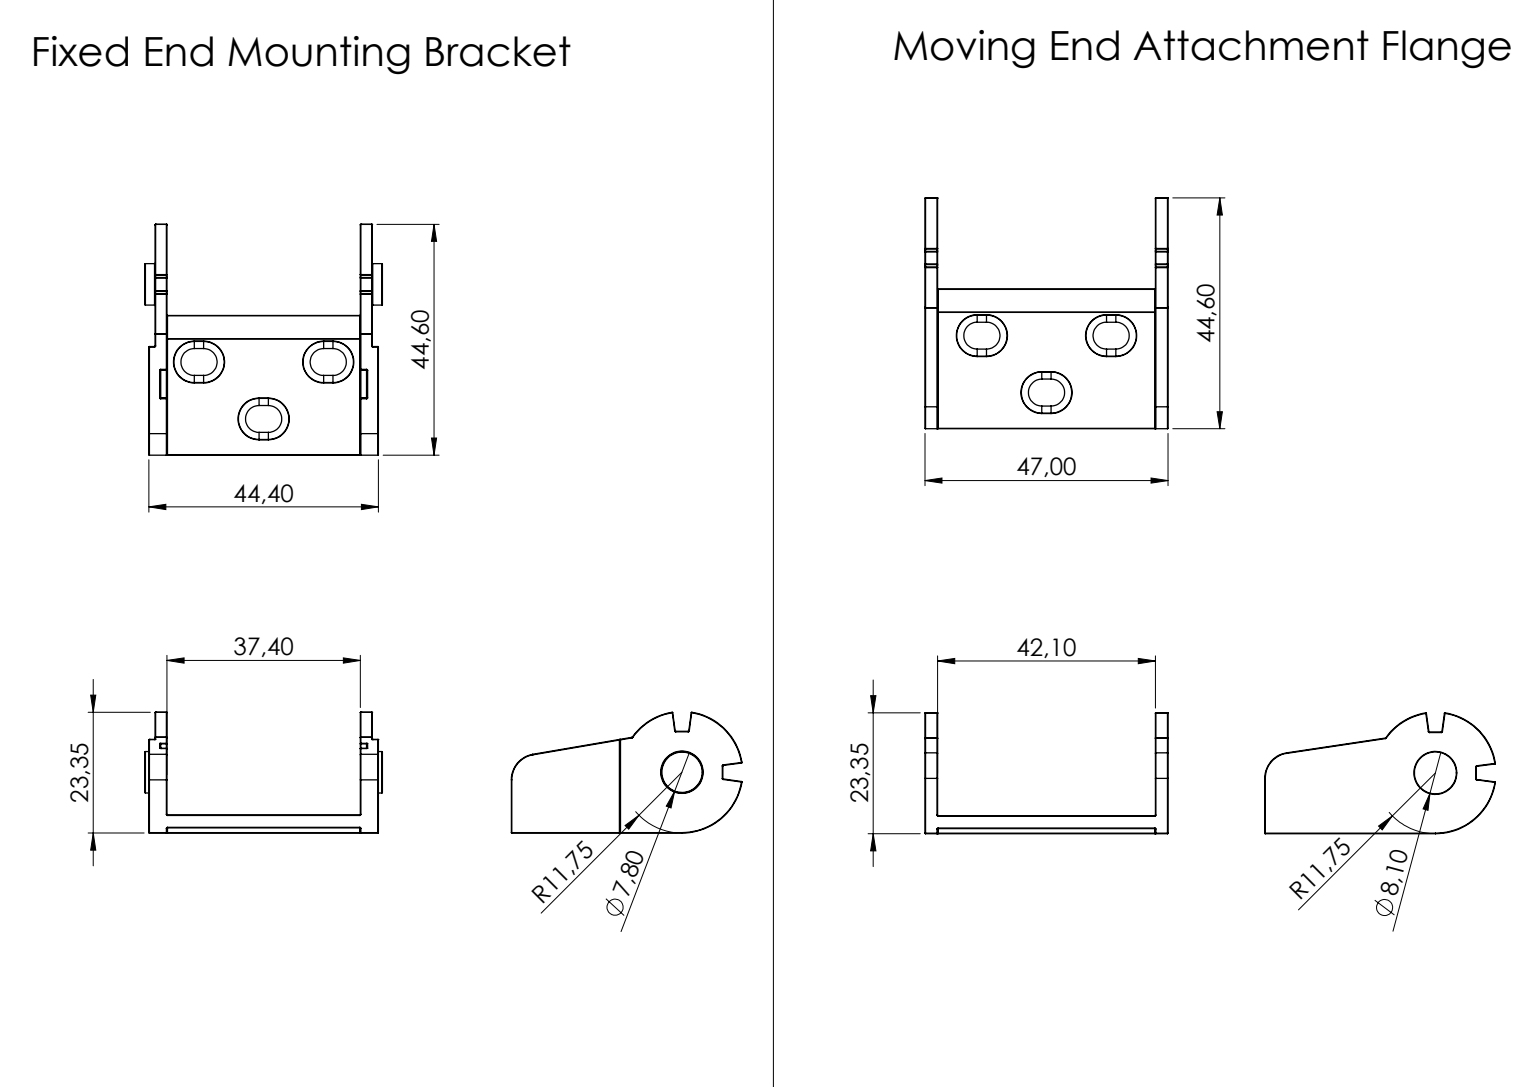
ISO-10303-21;
HEADER;
FILE_DESCRIPTION (('STEP AP214'),
    '1' );
FILE_NAME ('Fixed End Mounting Bracket.step',
    '2026-10-08T22:59:04',
    ( '' ),
    ( '' ),
    'SwSTEP 2.0',
    'SolidWorks 2020',
    '' );
FILE_SCHEMA (( 'AUTOMOTIVE_DESIGN' ));
ENDSEC;

DATA;
#41=ADVANCED_FACE ( 'NONE', ( #121306 ), #43023, .F. ) ;
#64=DIRECTION ( 'NONE',  ( 0.000000000000000000, 0.000000000000000000, 1.000000000000000000 ) ) ;
#92=CARTESIAN_POINT ( 'NONE',  ( -20.90000000000000213, 6.336640076952988920, 12.03401928653448572 ) ) ;
#126=VERTEX_POINT ( 'NONE', #92393 ) ;
#149=AXIS2_PLACEMENT_3D ( 'NONE', #44529, #5360, #61520 ) ;
#183=ADVANCED_FACE ( 'NONE', ( #7745 ), #109386, .T. ) ;
#187=EDGE_LOOP ( 'NONE', ( #19437, #210011, #114046, #182505, #122843 ) ) ;
#208=CIRCLE ( 'NONE', #96054, 11.75000000000000000 ) ;
#224=AXIS2_PLACEMENT_3D ( 'NONE', #149688, #207076, #227918 ) ;
#237=AXIS2_PLACEMENT_3D ( 'NONE', #83814, #157333, #257616 ) ;
#267=DIRECTION ( 'NONE',  ( 0.000000000000000000, -1.000000000000000000, 0.000000000000000000 ) ) ;
#284=EDGE_CURVE ( 'NONE', #234077, #216189, #164488, .T. ) ;
#339=ADVANCED_FACE ( 'NONE', ( #38863 ), #118398, .T. ) ;
#453=DIRECTION ( 'NONE',  ( 1.000000000000000000, 0.000000000000000000, -0.000000000000000000 ) ) ;
#495=VECTOR ( 'NONE', #96044, 1000.000000000000000 ) ;
#497=CARTESIAN_POINT ( 'NONE',  ( -22.10000000000000142, -11.65000000000000036, 12.09999999999999609 ) ) ;
#504=DIRECTION ( 'NONE',  ( 0.000000000000000000, 1.000000000000000000, 0.000000000000000000 ) ) ;
#539=FACE_OUTER_BOUND ( 'NONE', #95996, .T. ) ;
#576=DIRECTION ( 'NONE',  ( 0.000000000000000000, 1.000000000000000000, 0.000000000000000000 ) ) ;
#604=SPHERICAL_SURFACE ( 'NONE', #217070, 0.1000000000000000056 ) ;
#605=DIRECTION ( 'NONE',  ( 1.000000000000000000, -0.000000000000000000, 0.000000000000000000 ) ) ;
#660=CIRCLE ( 'NONE', #167314, 0.1000000000000002554 ) ;
#678=ORIENTED_EDGE ( 'NONE', *, *, #100875, .T. ) ;
#691=VERTEX_POINT ( 'NONE', #157234 ) ;
#709=CARTESIAN_POINT ( 'NONE',  ( 18.69999999999999929, -11.65000000000000036, -15.00000000000000000 ) ) ;
#736=ORIENTED_EDGE ( 'NONE', *, *, #51566, .T. ) ;
#739=CARTESIAN_POINT ( 'NONE',  ( 21.10000000000000142, 6.223900101154156594, 12.09999999999999964 ) ) ;
#754=EDGE_LOOP ( 'NONE', ( #252584, #112082, #982, #102048 ) ) ;
#803=EDGE_LOOP ( 'NONE', ( #185870, #252756, #109743, #49629 ) ) ;
#825=CARTESIAN_POINT ( 'NONE',  ( -21.00000000000000000, 7.800000000000000711, -1.212568896937008089 ) ) ;
#890=DIRECTION ( 'NONE',  ( -1.476360405086644309E-16, -1.000000000000000000, -0.000000000000000000 ) ) ;
#959=CARTESIAN_POINT ( 'NONE',  ( 13.40000000000000036, -11.65000000000000036, 17.70000000000000284 ) ) ;
#967=VECTOR ( 'NONE', #117987, 1000.000000000000114 ) ;
#975=VERTEX_POINT ( 'NONE', #144040 ) ;
#982=ORIENTED_EDGE ( 'NONE', *, *, #230832, .F. ) ;
#998=VECTOR ( 'NONE', #226913, 1000.000000000000000 ) ;
#1011=CYLINDRICAL_SURFACE ( 'NONE', #164253, 0.1000000000000001443 ) ;
#1037=TOROIDAL_SURFACE ( 'NONE', #71828, 0.2000000000000000111, 0.1000000000000000056 ) ;
#1051=ADVANCED_FACE ( 'NONE', ( #15824 ), #217817, .T. ) ;
#1072=CARTESIAN_POINT ( 'NONE',  ( 18.79999999999999716, 6.841561409100513025, 9.675512259591560138 ) ) ;
#1117=ORIENTED_EDGE ( 'NONE', *, *, #211260, .F. ) ;
#1141=EDGE_CURVE ( 'NONE', #118769, #81824, #59092, .T. ) ;
#1148=DIRECTION ( 'NONE',  ( 0.000000000000000000, -0.1335171055202864221, 0.9910465087640865089 ) ) ;
#1165=ORIENTED_EDGE ( 'NONE', *, *, #245877, .T. ) ;
#1224=VERTEX_POINT ( 'NONE', #31242 ) ;
#1234=CARTESIAN_POINT ( 'NONE',  ( -18.59999999999999787, -11.75000000000000000, 29.89999999999999858 ) ) ;
#1236=CARTESIAN_POINT ( 'NONE',  ( -18.59999999999999787, 11.75000000000000000, 30.09999999999999787 ) ) ;
#1243=ORIENTED_EDGE ( 'NONE', *, *, #90316, .T. ) ;
#1267=EDGE_CURVE ( 'NONE', #34286, #18345, #17600, .T. ) ;
#1279=DIRECTION ( 'NONE',  ( -0.000000000000000000, 1.000000000000000000, -0.000000000000000000 ) ) ;
#1290=FACE_OUTER_BOUND ( 'NONE', #252660, .T. ) ;
#1333=DIRECTION ( 'NONE',  ( 0.000000000000000000, 0.000000000000000000, 1.000000000000000000 ) ) ;
#1339=FACE_BOUND ( 'NONE', #186909, .T. ) ;
#1346=ADVANCED_FACE ( 'NONE', ( #229406 ), #188493, .T. ) ;
#1351=EDGE_LOOP ( 'NONE', ( #149134, #36739, #59727, #188975 ) ) ;
#1352=CARTESIAN_POINT ( 'NONE',  ( 13.40000000000000036, -8.350000000000004974, 19.04142135623731136 ) ) ;
#1419=DIRECTION ( 'NONE',  ( 0.000000000000000000, 0.000000000000000000, -1.000000000000000000 ) ) ;
#1439=ORIENTED_EDGE ( 'NONE', *, *, #171966, .F. ) ;
#1461=ADVANCED_FACE ( 'NONE', ( #80550 ), #121028, .T. ) ;
#1491=DIRECTION ( 'NONE',  ( 0.000000000000000000, -0.8164989248600462712, 0.5773469543544753613 ) ) ;
#1524=FACE_OUTER_BOUND ( 'NONE', #20858, .T. ) ;
#1526=VECTOR ( 'NONE', #257656, 1000.000000000000000 ) ;
#1596=AXIS2_PLACEMENT_3D ( 'NONE', #245526, #66878, #107284 ) ;
#1654=ADVANCED_FACE ( 'NONE', ( #246089 ), #129957, .F. ) ;
#1677=ORIENTED_EDGE ( 'NONE', *, *, #116347, .F. ) ;
#1687=ORIENTED_EDGE ( 'NONE', *, *, #137543, .F. ) ;
#1729=VERTEX_POINT ( 'NONE', #175549 ) ;
#1745=DIRECTION ( 'NONE',  ( 1.000000000000000000, 0.000000000000000000, 0.000000000000000000 ) ) ;
#1778=ADVANCED_FACE ( 'NONE', ( #195115 ), #16473, .T. ) ;
#1785=CIRCLE ( 'NONE', #147559, 0.09999999999999939493 ) ;
#1792=LINE ( 'NONE', #116623, #180804 ) ;
#1819=DIRECTION ( 'NONE',  ( 1.000000000000000000, 0.000000000000000000, 0.000000000000000000 ) ) ;
#1843=CARTESIAN_POINT ( 'NONE',  ( -6.000000000000003553, -11.65000000000000036, 10.00000000000000178 ) ) ;
#1922=CIRCLE ( 'NONE', #18693, 4.900000000000003020 ) ;
#2023=DIRECTION ( 'NONE',  ( -0.000000000000000000, 1.000000000000000000, -0.000000000000000000 ) ) ;
#2042=ORIENTED_EDGE ( 'NONE', *, *, #74139, .F. ) ;
#2050=CARTESIAN_POINT ( 'NONE',  ( -0.8999999999999994671, -8.350000000000003197, 21.95857864376269220 ) ) ;
#2071=AXIS2_PLACEMENT_3D ( 'NONE', #163669, #185794, #86661 ) ;
#2114=ADVANCED_FACE ( 'NONE', ( #116537 ), #211788, .T. ) ;
#2129=DIRECTION ( 'NONE',  ( 0.000000000000000000, 0.000000000000000000, -1.000000000000000000 ) ) ;
#2147=VERTEX_POINT ( 'NONE', #216897 ) ;
#2150=CARTESIAN_POINT ( 'NONE',  ( 20.09999999673965121, 5.571292164246353984, 16.50791943615039514 ) ) ;
#2234=VECTOR ( 'NONE', #4879, 1000.000000000000000 ) ;
#2304=CARTESIAN_POINT ( 'NONE',  ( -6.000000000000002665, -11.25000000000000000, 14.00000000000000178 ) ) ;
#2307=DIRECTION ( 'NONE',  ( 4.336808689942017736E-16, 0.000000000000000000, 1.000000000000000000 ) ) ;
#2318=CARTESIAN_POINT ( 'NONE',  ( -22.10000000000000497, 6.223900101154156594, 12.09999999999999964 ) ) ;
#2328=AXIS2_PLACEMENT_3D ( 'NONE', #70395, #7830, #149920 ) ;
#2358=EDGE_CURVE ( 'NONE', #239783, #205125, #234657, .T. ) ;
#2425=AXIS2_PLACEMENT_3D ( 'NONE', #153513, #135160, #16531 ) ;
#2475=ORIENTED_EDGE ( 'NONE', *, *, #234542, .T. ) ;
#2486=EDGE_CURVE ( 'NONE', #219374, #227995, #238605, .T. ) ;
#2561=CARTESIAN_POINT ( 'NONE',  ( -22.10000000000000142, -11.64999999999999858, 12.09999999999999609 ) ) ;
#2564=DIRECTION ( 'NONE',  ( 1.000000000000000000, 5.204170427930452838E-14, 0.000000000000000000 ) ) ;
#2588=CARTESIAN_POINT ( 'NONE',  ( -37.88850191057539973, 11.75000000000000000, 6.000000000000001776 ) ) ;
#2624=CYLINDRICAL_SURFACE ( 'NONE', #233334, 0.09999999999999990841 ) ;
#2683=ORIENTED_EDGE ( 'NONE', *, *, #33531, .T. ) ;
#2711=AXIS2_PLACEMENT_3D ( 'NONE', #47359, #90346, #129493 ) ;
#2743=CARTESIAN_POINT ( 'NONE',  ( -18.70000000000000284, 7.900000000000000355, 1.212568896937007867 ) ) ;
#2774=CIRCLE ( 'NONE', #236010, 0.09999999999999990841 ) ;
#2777=PLANE ( 'NONE',  #123368 ) ;
#2798=VECTOR ( 'NONE', #76671, 1000.000000000000000 ) ;
#2843=CARTESIAN_POINT ( 'NONE',  ( 18.79999999999999716, 6.783826713665066066, 9.593862367105556288 ) ) ;
#2853=VECTOR ( 'NONE', #232428, 1000.000000000000114 ) ;
#2924=EDGE_CURVE ( 'NONE', #166883, #29111, #110106, .T. ) ;
#2933=CYLINDRICAL_SURFACE ( 'NONE', #81036, 0.09999999999999939493 ) ;
#3014=CARTESIAN_POINT ( 'NONE',  ( -22.84999999999999787, 0.000000000000000000, 0.000000000000000000 ) ) ;
#3017=CARTESIAN_POINT ( 'NONE',  ( -21.10000000000000142, -11.64999999999999858, 11.99999999999999645 ) ) ;
#3030=CARTESIAN_POINT ( 'NONE',  ( 20.10000000000000853, 4.645987002755569861, 21.91686199900910736 ) ) ;
#3071=CARTESIAN_POINT ( 'NONE',  ( 20.89999999999999858, -11.75000000000000000, 11.89999999999999680 ) ) ;
#3085=AXIS2_PLACEMENT_3D ( 'NONE', #145893, #127634, #7698 ) ;
#3098=CARTESIAN_POINT ( 'NONE',  ( 18.59999999999999787, -9.849999999999994316, 30.09999999999999787 ) ) ;
#3161=CARTESIAN_POINT ( 'NONE',  ( 18.79999999999999716, -1.885425182446134107, -11.59641995933507808 ) ) ;
#3206=CARTESIAN_POINT ( 'NONE',  ( 18.79999999999999716, 11.49641995933507843, 1.885425182446133885 ) ) ;
#3219=DIRECTION ( 'NONE',  ( -0.000000000000000000, 0.9910465087640860649, 0.1335171055202901413 ) ) ;
#3268=CIRCLE ( 'NONE', #36650, 0.1000000000000000472 ) ;
#3271=ORIENTED_EDGE ( 'NONE', *, *, #83209, .F. ) ;
#3359=CYLINDRICAL_SURFACE ( 'NONE', #28672, 0.1000000000000000472 ) ;
#3419=DIRECTION ( 'NONE',  ( 0.000000000000000000, 0.000000000000000000, -1.000000000000000000 ) ) ;
#3449=EDGE_CURVE ( 'NONE', #86236, #255967, #27127, .T. ) ;
#3491=DIRECTION ( 'NONE',  ( 1.000000000000000000, 0.000000000000000000, 0.000000000000000000 ) ) ;
#3501=EDGE_CURVE ( 'NONE', #252739, #56541, #35327, .T. ) ;
#3516=ORIENTED_EDGE ( 'NONE', *, *, #242810, .F. ) ;
#3541=DIRECTION ( 'NONE',  ( 0.000000000000000000, 0.000000000000000000, -1.000000000000000000 ) ) ;
#3551=ORIENTED_EDGE ( 'NONE', *, *, #74542, .T. ) ;
#3558=DIRECTION ( 'NONE',  ( 2.168404344971008868E-16, 0.000000000000000000, 1.000000000000000000 ) ) ;
#3600=FACE_OUTER_BOUND ( 'NONE', #170206, .T. ) ;
#3613=CARTESIAN_POINT ( 'NONE',  ( 18.59999999999999787, -8.150000000000007461, 33.00000000000000000 ) ) ;
#3619=ORIENTED_EDGE ( 'NONE', *, *, #97666, .T. ) ;
#3638=DIRECTION ( 'NONE',  ( 0.000000000000000000, 0.000000000000000000, -1.000000000000000000 ) ) ;
#3653=AXIS2_PLACEMENT_3D ( 'NONE', #213131, #137431, #235256 ) ;
#3657=ORIENTED_EDGE ( 'NONE', *, *, #144860, .T. ) ;
#3734=VECTOR ( 'NONE', #55279, 1000.000000000000114 ) ;
#3738=VERTEX_POINT ( 'NONE', #126244 ) ;
#3792=DIRECTION ( 'NONE',  ( 1.000000000000000000, 0.000000000000000000, -0.000000000000000000 ) ) ;
#3847=CARTESIAN_POINT ( 'NONE',  ( 18.69999999999999929, 13.48082180182240819, -2.152770446119438130 ) ) ;
#3921=ORIENTED_EDGE ( 'NONE', *, *, #230794, .T. ) ;
#3965=EDGE_CURVE ( 'NONE', #120372, #6846, #74023, .T. ) ;
#4061=CARTESIAN_POINT ( 'NONE',  ( 20.90000000000000213, 6.783826713665066066, 9.593862367105556288 ) ) ;
#4072=DIRECTION ( 'NONE',  ( 1.000000000000000000, 0.000000000000000000, 0.000000000000000000 ) ) ;
#4080=ADVANCED_FACE ( 'NONE', ( #122104 ), #257691, .F. ) ;
#4122=FACE_OUTER_BOUND ( 'NONE', #6960, .T. ) ;
#4146=AXIS2_PLACEMENT_3D ( 'NONE', #228967, #90718, #131136 ) ;
#4152=LINE ( 'NONE', #44579, #184468 ) ;
#4188=AXIS2_PLACEMENT_3D ( 'NONE', #227607, #206772, #110226 ) ;
#4213=LINE ( 'NONE', #22529, #191256 ) ;
#4245=CARTESIAN_POINT ( 'NONE',  ( 22.10000000000000142, -3.262756495241484158E-15, 33.00000000000000000 ) ) ;
#4267=EDGE_CURVE ( 'NONE', #92180, #44902, #131505, .T. ) ;
#4282=ORIENTED_EDGE ( 'NONE', *, *, #241945, .T. ) ;
#4370=ADVANCED_FACE ( 'NONE', ( #539 ), #103482, .F. ) ;
#4421=LINE ( 'NONE', #83919, #253429 ) ;
#4438=CARTESIAN_POINT ( 'NONE',  ( -18.59999999999999787, -9.849999999999994316, 30.09999999999999787 ) ) ;
#4483=DIRECTION ( 'NONE',  ( 0.000000000000000000, 0.000000000000000000, -1.000000000000000000 ) ) ;
#4552=ORIENTED_EDGE ( 'NONE', *, *, #61719, .T. ) ;
#4630=ORIENTED_EDGE ( 'NONE', *, *, #141720, .T. ) ;
#4636=ORIENTED_EDGE ( 'NONE', *, *, #215592, .T. ) ;
#4637=DIRECTION ( 'NONE',  ( 1.000000000000000000, -0.000000000000000000, -0.000000000000000000 ) ) ;
#4689=CARTESIAN_POINT ( 'NONE',  ( -18.59999999999999787, -8.350000000000004974, 10.52591260281975138 ) ) ;
#4690=FACE_OUTER_BOUND ( 'NONE', #81853, .T. ) ;
#4754=TOROIDAL_SURFACE ( 'NONE', #38128, 2.699999999999999734, 0.1000000000000000056 ) ;
#4815=CARTESIAN_POINT ( 'NONE',  ( 18.59999999999999787, -11.75000000000000000, 29.89999999999999858 ) ) ;
#4828=ORIENTED_EDGE ( 'NONE', *, *, #139777, .F. ) ;
#4859=ORIENTED_EDGE ( 'NONE', *, *, #16669, .F. ) ;
#4879=DIRECTION ( 'NONE',  ( 1.000000000000000000, 0.000000000000000000, 0.000000000000000000 ) ) ;
#4900=LINE ( 'NONE', #234236, #76259 ) ;
#4904=CARTESIAN_POINT ( 'NONE',  ( -18.69999999999999929, -8.175168544775697654, 10.42878401658402510 ) ) ;
#4929=DIRECTION ( 'NONE',  ( 0.000000000000000000, 0.000000000000000000, -1.000000000000000000 ) ) ;
#4955=ORIENTED_EDGE ( 'NONE', *, *, #96401, .T. ) ;
#4967=EDGE_CURVE ( 'NONE', #172933, #119804, #217712, .T. ) ;
#4990=DIRECTION ( 'NONE',  ( -0.000000000000000000, 0.000000000000000000, -1.000000000000000000 ) ) ;
#4992=FACE_OUTER_BOUND ( 'NONE', #63102, .T. ) ;
#5028=DIRECTION ( 'NONE',  ( 0.000000000000000000, -0.9910465087640861759, -0.1335171055202901691 ) ) ;
#5031=LINE ( 'NONE', #44202, #91258 ) ;
#5040=DIRECTION ( 'NONE',  ( 1.000000000000000000, 0.000000000000000000, 0.000000000000000000 ) ) ;
#5080=VERTEX_POINT ( 'NONE', #116060 ) ;
#5094=EDGE_CURVE ( 'NONE', #73306, #188929, #47029, .T. ) ;
#5097=CARTESIAN_POINT ( 'NONE',  ( -18.79999999999999716, -8.150000000000005684, 32.89999999999999858 ) ) ;
#5118=CARTESIAN_POINT ( 'NONE',  ( -11.60000000000000320, -11.75000000000000000, 12.30000000000000426 ) ) ;
#5188=ADVANCED_FACE ( 'NONE', ( #244973 ), #230202, .F. ) ;
#5266=ORIENTED_EDGE ( 'NONE', *, *, #96420, .F. ) ;
#5299=AXIS2_PLACEMENT_3D ( 'NONE', #140383, #159989, #178273 ) ;
#5313=DIRECTION ( 'NONE',  ( 0.000000000000000000, -0.9910465087640860649, -0.1335171055202901413 ) ) ;
#5331=DIRECTION ( 'NONE',  ( 1.000000000000000000, 0.000000000000000000, 0.000000000000000000 ) ) ;
#5360=DIRECTION ( 'NONE',  ( 0.000000000000000000, -1.000000000000000000, 0.000000000000000000 ) ) ;
#5371=CIRCLE ( 'NONE', #159540, 2.699999999999999289 ) ;
#5385=CARTESIAN_POINT ( 'NONE',  ( -18.59999999999999787, -11.75000000000000000, 5.900000000000001243 ) ) ;
#5427=PRODUCT_DEFINITION ( 'UNKNOWN', '', #69634, #100050 ) ;
#5432=CARTESIAN_POINT ( 'NONE',  ( -21.10000000000000142, 0.000000000000000000, 0.000000000000000000 ) ) ;
#5456=EDGE_LOOP ( 'NONE', ( #217930, #251861, #121783, #237435 ) ) ;
#5556=DIRECTION ( 'NONE',  ( 1.000000000000000000, -0.000000000000000000, 0.000000000000000000 ) ) ;
#5568=VERTEX_POINT ( 'NONE', #108688 ) ;
#5645=EDGE_CURVE ( 'NONE', #194417, #150252, #248397, .T. ) ;
#5669=VERTEX_POINT ( 'NONE', #7013 ) ;
#5674=FACE_OUTER_BOUND ( 'NONE', #24234, .T. ) ;
#5678=FACE_OUTER_BOUND ( 'NONE', #72669, .T. ) ;
#5679=FACE_OUTER_BOUND ( 'NONE', #105384, .T. ) ;
#5712=DIRECTION ( 'NONE',  ( 0.000000000000000000, 0.000000000000000000, 1.000000000000000000 ) ) ;
#5762=AXIS2_PLACEMENT_3D ( 'NONE', #31364, #249105, #129143 ) ;
#5812=EDGE_CURVE ( 'NONE', #155056, #32241, #211000, .T. ) ;
#5833=AXIS2_PLACEMENT_3D ( 'NONE', #21551, #101019, #180617 ) ;
#5834=CARTESIAN_POINT ( 'NONE',  ( 11.60000000000000142, -8.350000000000004974, 10.95857864376269575 ) ) ;
#5907=ORIENTED_EDGE ( 'NONE', *, *, #56458, .T. ) ;
#5926=FACE_OUTER_BOUND ( 'NONE', #220597, .T. ) ;
#5938=TOROIDAL_SURFACE ( 'NONE', #47632, 0.2000000000000000111, 0.1000000000000000056 ) ;
#5962=ORIENTED_EDGE ( 'NONE', *, *, #10052, .F. ) ;
#5977=CYLINDRICAL_SURFACE ( 'NONE', #90984, 0.09999999999999939493 ) ;
#6001=CARTESIAN_POINT ( 'NONE',  ( 21.00000000000000000, 6.726092018229619995, 9.512212474619552438 ) ) ;
#6100=CARTESIAN_POINT ( 'NONE',  ( -18.79999999999999716, 3.362550747017869490, 28.82623795144604983 ) ) ;
#6120=LINE ( 'NONE', #100076, #98789 ) ;
#6126=DIRECTION ( 'NONE',  ( -0.000000000000000000, 1.000000000000000000, -0.000000000000000000 ) ) ;
#6150=ORIENTED_EDGE ( 'NONE', *, *, #36982, .T. ) ;
#6158=ORIENTED_EDGE ( 'NONE', *, *, #5645, .T. ) ;
#6172=ORIENTED_EDGE ( 'NONE', *, *, #225918, .F. ) ;
#6218=DIRECTION ( 'NONE',  ( -1.000000000000000000, 0.000000000000000000, -0.000000000000000000 ) ) ;
#6242=EDGE_LOOP ( 'NONE', ( #236481, #171353, #241692, #160210 ) ) ;
#6249=DIRECTION ( 'NONE',  ( -0.000000000000000000, 1.000000000000000000, -0.000000000000000000 ) ) ;
#6288=EDGE_CURVE ( 'NONE', #23890, #34850, #119612, .T. ) ;
#6301=DIRECTION ( 'NONE',  ( -0.000000000000000000, -0.000000000000000000, 1.000000000000000000 ) ) ;
#6322=DIRECTION ( 'NONE',  ( 0.000000000000000000, -1.000000000000000000, -1.445602896647339410E-16 ) ) ;
#6340=LINE ( 'NONE', #108033, #219074 ) ;
#6348=EDGE_CURVE ( 'NONE', #248319, #79944, #173820, .T. ) ;
#6387=CARTESIAN_POINT ( 'NONE',  ( -20.09999999999999787, 5.552655413246003313, 16.61686199900910310 ) ) ;
#6398=DIRECTION ( 'NONE',  ( 0.000000000000000000, 0.000000000000000000, 1.000000000000000000 ) ) ;
#6400=EDGE_CURVE ( 'NONE', #192900, #109505, #117252, .T. ) ;
#6406=ORIENTED_EDGE ( 'NONE', *, *, #148673, .F. ) ;
#6447=EDGE_LOOP ( 'NONE', ( #197308, #76668, #190493 ) ) ;
#6463=ORIENTED_EDGE ( 'NONE', *, *, #103505, .F. ) ;
#6496=VERTEX_POINT ( 'NONE', #242317 ) ;
#6499=DIRECTION ( 'NONE',  ( 0.000000000000000000, -0.4856429311786307212, -0.8741572761215384846 ) ) ;
#6503=EDGE_CURVE ( 'NONE', #103588, #211037, #118553, .T. ) ;
#6504=DIRECTION ( 'NONE',  ( -1.000000000000000000, -0.000000000000000000, -0.000000000000000000 ) ) ;
#6562=DIRECTION ( 'NONE',  ( 0.000000000000000000, 0.000000000000000000, -1.000000000000000000 ) ) ;
#6570=DIRECTION ( 'NONE',  ( 0.000000000000000000, -8.881784197001252323E-16, 1.000000000000000000 ) ) ;
#6639=CARTESIAN_POINT ( 'NONE',  ( 21.00000000000000000, 0.000000000000000000, 0.000000000000000000 ) ) ;
#6645=CIRCLE ( 'NONE', #214927, 4.041421356237310469 ) ;
#6690=CARTESIAN_POINT ( 'NONE',  ( -11.60000000000000320, -8.250000000000007105, 15.00000000000000355 ) ) ;
#6722=DIRECTION ( 'NONE',  ( 0.000000000000000000, 1.000000000000000000, 0.000000000000000000 ) ) ;
#6757=DIRECTION ( 'NONE',  ( 1.000000000000000000, 0.000000000000000000, -3.469446951953635015E-14 ) ) ;
#6794=DIRECTION ( 'NONE',  ( 2.895190717381441586E-16, -0.1335171055202867274, -0.9910465087640865089 ) ) ;
#6823=VECTOR ( 'NONE', #171824, 1000.000000000000000 ) ;
#6844=VECTOR ( 'NONE', #230845, 1000.000000000000000 ) ;
#6846=VERTEX_POINT ( 'NONE', #126886 ) ;
#6897=CARTESIAN_POINT ( 'NONE',  ( 19.90000000000000568, 4.631764625546185066, 22.00000000000000355 ) ) ;
#6960=EDGE_LOOP ( 'NONE', ( #51440, #18902, #50376, #104913 ) ) ;
#6966=DIRECTION ( 'NONE',  ( -1.000000000000000000, -0.000000000000000000, -0.000000000000000000 ) ) ;
#7013=CARTESIAN_POINT ( 'NONE',  ( 18.69999999999999929, 11.49641995933507843, 1.885425182446133441 ) ) ;
#7040=CARTESIAN_POINT ( 'NONE',  ( -20.90000000000000213, 7.800000000000000711, 1.212568896937007867 ) ) ;
#7083=CARTESIAN_POINT ( 'NONE',  ( 5.899999999999995914, -11.34999999999999964, 10.00000000000000178 ) ) ;
#7107=DIRECTION ( 'NONE',  ( 1.000000000000000000, 0.000000000000000000, 0.000000000000000000 ) ) ;
#7108=EDGE_CURVE ( 'NONE', #167847, #138780, #231144, .T. ) ;
#7188=CIRCLE ( 'NONE', #3085, 0.09999999999999939493 ) ;
#7204=CIRCLE ( 'NONE', #36295, 0.09999999999999993616 ) ;
#7218=DIRECTION ( 'NONE',  ( 0.000000000000000000, -0.000000000000000000, -1.000000000000000000 ) ) ;
#7276=ORIENTED_EDGE ( 'NONE', *, *, #119630, .F. ) ;
#7295=FACE_OUTER_BOUND ( 'NONE', #254168, .T. ) ;
#7312=AXIS2_PLACEMENT_3D ( 'NONE', #21356, #56565, #254752 ) ;
#7332=EDGE_CURVE ( 'NONE', #8702, #160911, #181931, .T. ) ;
#7385=DIRECTION ( 'NONE',  ( -1.000000000000000000, 0.000000000000000000, 0.000000000000000000 ) ) ;
#7390=DIRECTION ( 'NONE',  ( -1.462545276649575732E-15, 0.1686199900910455851, -0.9856811345164804283 ) ) ;
#7441=VECTOR ( 'NONE', #223820, 1000.000000000000000 ) ;
#7442=EDGE_CURVE ( 'NONE', #171697, #210883, #219514, .T. ) ;
#7521=VERTEX_POINT ( 'NONE', #191725 ) ;
#7531=DIRECTION ( 'NONE',  ( 0.000000000000000000, -1.000000000000000000, 0.000000000000000000 ) ) ;
#7605=CIRCLE ( 'NONE', #28302, 0.09999999999999939493 ) ;
#7635=AXIS2_PLACEMENT_3D ( 'NONE', #49675, #32725, #129220 ) ;
#7640=DIRECTION ( 'NONE',  ( -1.000000000000000000, 0.000000000000000000, 0.000000000000000000 ) ) ;
#7659=EDGE_LOOP ( 'NONE', ( #228235, #166303, #8737, #34445 ) ) ;
#7692=LINE ( 'NONE', #241169, #95485 ) ;
#7698=DIRECTION ( 'NONE',  ( 0.000000000000000000, 0.000000000000000000, 1.000000000000000000 ) ) ;
#7730=CARTESIAN_POINT ( 'NONE',  ( -20.90000000000000213, 3.362550747017865493, 28.82623795144604983 ) ) ;
#7745=FACE_OUTER_BOUND ( 'NONE', #18036, .T. ) ;
#7770=CARTESIAN_POINT ( 'NONE',  ( 13.40000000000000036, -11.65000000000000036, 12.40000000000000391 ) ) ;
#7808=EDGE_CURVE ( 'NONE', #248444, #169606, #115663, .T. ) ;
#7810=DIRECTION ( 'NONE',  ( 0.000000000000000000, -1.776356839400250465E-15, -1.000000000000000000 ) ) ;
#7830=DIRECTION ( 'NONE',  ( 1.000000000000000000, -0.000000000000000000, -0.000000000000000000 ) ) ;
#7880=AXIS2_PLACEMENT_3D ( 'NONE', #73088, #18213, #152619 ) ;
#7884=DIRECTION ( 'NONE',  ( 0.000000000000000000, 1.000000000000000000, 0.000000000000000000 ) ) ;
#7949=CIRCLE ( 'NONE', #74603, 2.600000000000000089 ) ;
#7966=ORIENTED_EDGE ( 'NONE', *, *, #255799, .F. ) ;
#8033=VERTEX_POINT ( 'NONE', #212246 ) ;
#8035=CARTESIAN_POINT ( 'NONE',  ( -11.60000000000000320, -11.75000000000000000, 17.70000000000000639 ) ) ;
#8038=DIRECTION ( 'NONE',  ( -0.000000000000000000, -0.1686199900910312910, 0.9856811345164826488 ) ) ;
#8040=DIRECTION ( 'NONE',  ( -1.000000000000000000, 0.000000000000000000, 0.000000000000000000 ) ) ;
#8093=ORIENTED_EDGE ( 'NONE', *, *, #45722, .T. ) ;
#8100=VERTEX_POINT ( 'NONE', #233102 ) ;
#8156=CARTESIAN_POINT ( 'NONE',  ( 18.79999999999999716, 8.000000000000000000, 1.212568896937007867 ) ) ;
#8168=ORIENTED_EDGE ( 'NONE', *, *, #181764, .T. ) ;
#8225=CARTESIAN_POINT ( 'NONE',  ( 22.94999999999999929, 6.223900101154157483, 12.00000000000000000 ) ) ;
#8268=DIRECTION ( 'NONE',  ( 1.000000000000000000, 0.000000000000000000, 0.000000000000000000 ) ) ;
#8316=ORIENTED_EDGE ( 'NONE', *, *, #63567, .T. ) ;
#8338=LINE ( 'NONE', #33074, #105846 ) ;
#8379=TOROIDAL_SURFACE ( 'NONE', #41707, 0.2000000000000000111, 0.1000000000000000056 ) ;
#8392=CIRCLE ( 'NONE', #32802, 0.2000000000000000944 ) ;
#8418=EDGE_CURVE ( 'NONE', #79944, #210883, #257433, .T. ) ;
#8444=ORIENTED_EDGE ( 'NONE', *, *, #28789, .F. ) ;
#8461=LINE ( 'NONE', #149270, #238692 ) ;
#8468=DIRECTION ( 'NONE',  ( 0.000000000000000000, -0.9910465087640860649, 0.1335171055202901413 ) ) ;
#8473=DIRECTION ( 'NONE',  ( 0.000000000000000000, -0.9856811345164803173, -0.1686199900910455851 ) ) ;
#8554=DIRECTION ( 'NONE',  ( 0.000000000000000000, 0.000000000000000000, 1.000000000000000000 ) ) ;
#8617=CARTESIAN_POINT ( 'NONE',  ( 13.40000000000000036, -9.650000000000002132, 15.00000000000000355 ) ) ;
#8618=ORIENTED_EDGE ( 'NONE', *, *, #211407, .F. ) ;
#8650=ORIENTED_EDGE ( 'NONE', *, *, #117411, .T. ) ;
#8671=ADVANCED_FACE ( 'NONE', ( #5678 ), #226001, .T. ) ;
#8680=ADVANCED_FACE ( 'NONE', ( #246877 ), #29170, .T. ) ;
#8702=VERTEX_POINT ( 'NONE', #244305 ) ;
#8737=ORIENTED_EDGE ( 'NONE', *, *, #202652, .F. ) ;
#8769=DIRECTION ( 'NONE',  ( -1.000000000000000000, 0.000000000000000000, -0.000000000000000000 ) ) ;
#8910=CARTESIAN_POINT ( 'NONE',  ( -22.94999999999999929, 0.000000000000000000, -4.000000000000000000 ) ) ;
#8923=PLANE ( 'NONE',  #39786 ) ;
#8968=ORIENTED_EDGE ( 'NONE', *, *, #146894, .T. ) ;
#8980=DIRECTION ( 'NONE',  ( -1.000000000000000000, 0.000000000000000000, 0.000000000000000000 ) ) ;
#9039=ORIENTED_EDGE ( 'NONE', *, *, #252839, .T. ) ;
#9057=DIRECTION ( 'NONE',  ( -1.000000000000000000, -0.000000000000000000, -0.000000000000000000 ) ) ;
#9119=ADVANCED_FACE ( 'NONE', ( #88441 ), #236973, .F. ) ;
#9122=ORIENTED_EDGE ( 'NONE', *, *, #132131, .T. ) ;
#9309=ORIENTED_EDGE ( 'NONE', *, *, #186911, .F. ) ;
#9347=CARTESIAN_POINT ( 'NONE',  ( -0.8999999999999994671, -8.279289321881350361, 22.02928932188134326 ) ) ;
#9446=CIRCLE ( 'NONE', #159487, 0.2000000000000005107 ) ;
#9467=AXIS2_PLACEMENT_3D ( 'NONE', #37202, #154593, #175434 ) ;
#9474=ORIENTED_EDGE ( 'NONE', *, *, #181279, .T. ) ;
#9487=CARTESIAN_POINT ( 'NONE',  ( 20.90000000000000213, -1.212568896937008089, -7.800000000000000711 ) ) ;
#9509=ORIENTED_EDGE ( 'NONE', *, *, #68971, .F. ) ;
#9513=PLANE ( 'NONE',  #94477 ) ;
#9516=EDGE_CURVE ( 'NONE', #161437, #149939, #154045, .T. ) ;
#9527=AXIS2_PLACEMENT_3D ( 'NONE', #133334, #155498, #115051 ) ;
#9530=EDGE_CURVE ( 'NONE', #87211, #166805, #162377, .T. ) ;
#9566=LINE ( 'NONE', #244318, #140856 ) ;
#9592=DIRECTION ( 'NONE',  ( 0.000000000000000000, 0.000000000000000000, -1.000000000000000000 ) ) ;
#9628=DIRECTION ( 'NONE',  ( -0.000000000000000000, 1.000000000000000000, -0.000000000000000000 ) ) ;
#9632=CARTESIAN_POINT ( 'NONE',  ( -18.59999999999999787, -10.80884033489985363, 6.000000000000001776 ) ) ;
#9654=CIRCLE ( 'NONE', #126158, 0.09999999999999939493 ) ;
#9657=CIRCLE ( 'NONE', #130273, 0.1000000000000002554 ) ;
#9700=VERTEX_POINT ( 'NONE', #200106 ) ;
#9732=CARTESIAN_POINT ( 'NONE',  ( -22.94999999999999929, 11.61130914238355771, -1.800000000000000044 ) ) ;
#9748=ORIENTED_EDGE ( 'NONE', *, *, #249884, .F. ) ;
#9750=CARTESIAN_POINT ( 'NONE',  ( 19.90000000000000568, 1.350000000000000089, 21.90000000000000213 ) ) ;
#9751=ADVANCED_FACE ( 'NONE', ( #108711 ), #20930, .T. ) ;
#9850=DIRECTION ( 'NONE',  ( 0.000000000000000000, 0.9856811345164803173, 0.1686199900910455851 ) ) ;
#9860=EDGE_LOOP ( 'NONE', ( #137346, #244851, #139743, #56344 ) ) ;
#9899=CIRCLE ( 'NONE', #88993, 0.09999999999999939493 ) ;
#9958=CIRCLE ( 'NONE', #84755, 0.09999999999999939493 ) ;
#10010=VERTEX_POINT ( 'NONE', #39381 ) ;
#10023=AXIS2_PLACEMENT_3D ( 'NONE', #137310, #133476, #257219 ) ;
#10024=CARTESIAN_POINT ( 'NONE',  ( -18.79999999999999716, -11.65000000000000036, 33.00000000000000000 ) ) ;
#10045=DIRECTION ( 'NONE',  ( 0.000000000000000000, 0.000000000000000000, 1.000000000000000000 ) ) ;
#10052=EDGE_CURVE ( 'NONE', #245021, #45997, #175675, .T. ) ;
#10074=TOROIDAL_SURFACE ( 'NONE', #159945, 0.2000000000000000111, 0.1000000000000000056 ) ;
#10148=EDGE_CURVE ( 'NONE', #219738, #36888, #213057, .T. ) ;
#10149=AXIS2_PLACEMENT_3D ( 'NONE', #196970, #220411, #41791 ) ;
#10199=CARTESIAN_POINT ( 'NONE',  ( -11.60000000000000320, -12.25000000000000178, 15.00000000000000355 ) ) ;
#10202=DIRECTION ( 'NONE',  ( 0.000000000000000000, 0.000000000000000000, -1.000000000000000000 ) ) ;
#10206=CIRCLE ( 'NONE', #26777, 0.09999999999999993616 ) ;
#10231=CARTESIAN_POINT ( 'NONE',  ( -20.90000000326035590, 6.338045365888075544, 12.02580456186802138 ) ) ;
#10247=ORIENTED_EDGE ( 'NONE', *, *, #217423, .T. ) ;
#10267=ADVANCED_FACE ( 'NONE', ( #88718 ), #129163, .F. ) ;
#10270=FACE_OUTER_BOUND ( 'NONE', #187, .T. ) ;
#10287=AXIS2_PLACEMENT_3D ( 'NONE', #186442, #104300, #69069 ) ;
#10294=EDGE_CURVE ( 'NONE', #213256, #179078, #237994, .T. ) ;
#10308=EDGE_LOOP ( 'NONE', ( #230650, #214838, #47259, #48492 ) ) ;
#10311=AXIS2_PLACEMENT_3D ( 'NONE', #247977, #108476, #186748 ) ;
#10322=DIRECTION ( 'NONE',  ( 1.000000000000000000, -0.000000000000000000, -0.000000000000000000 ) ) ;
#10323=AXIS2_PLACEMENT_3D ( 'NONE', #156268, #216187, #137934 ) ;
#10387=ORIENTED_EDGE ( 'NONE', *, *, #241945, .F. ) ;
#10394=ORIENTED_EDGE ( 'NONE', *, *, #15881, .T. ) ;
#10411=ORIENTED_EDGE ( 'NONE', *, *, #225642, .F. ) ;
#10421=CIRCLE ( 'NONE', #210339, 0.09999999999999939493 ) ;
#10423=VERTEX_POINT ( 'NONE', #133020 ) ;
#10447=DIRECTION ( 'NONE',  ( 1.000000000000000000, 0.000000000000000000, 0.000000000000000000 ) ) ;
#10449=ORIENTED_EDGE ( 'NONE', *, *, #228397, .T. ) ;
#10454=ORIENTED_EDGE ( 'NONE', *, *, #177305, .T. ) ;
#10471=LINE ( 'NONE', #226942, #57164 ) ;
#10483=ORIENTED_EDGE ( 'NONE', *, *, #16578, .F. ) ;
#10495=AXIS2_PLACEMENT_3D ( 'NONE', #120614, #99710, #159724 ) ;
#10519=CARTESIAN_POINT ( 'NONE',  ( -6.000000000000002665, -11.65000000000000036, 13.90000000000000213 ) ) ;
#10528=DIRECTION ( 'NONE',  ( -1.000000000000000000, 0.000000000000000000, 0.000000000000000000 ) ) ;
#10555=ORIENTED_EDGE ( 'NONE', *, *, #237569, .T. ) ;
#10587=ORIENTED_EDGE ( 'NONE', *, *, #253546, .T. ) ;
#10603=DIRECTION ( 'NONE',  ( -1.000000000000000000, 0.000000000000000000, 0.000000000000000000 ) ) ;
#10671=CARTESIAN_POINT ( 'NONE',  ( 21.00000000000000000, 8.000000000000000000, 1.212568896937007867 ) ) ;
#10722=AXIS2_PLACEMENT_3D ( 'NONE', #97401, #238224, #15355 ) ;
#10746=AXIS2_PLACEMENT_3D ( 'NONE', #152283, #191418, #231811 ) ;
#10758=DIRECTION ( 'NONE',  ( -1.000000000000000000, -0.000000000000000000, -0.000000000000000000 ) ) ;
#10771=CARTESIAN_POINT ( 'NONE',  ( 18.79999999999999716, 5.488301202077012775, 16.40000000000000213 ) ) ;
#10787=CARTESIAN_POINT ( 'NONE',  ( -20.09999999999999787, 3.362550747017865493, 28.82623795144604983 ) ) ;
#10810=VERTEX_POINT ( 'NONE', #32349 ) ;
#10840=CYLINDRICAL_SURFACE ( 'NONE', #139892, 0.09999999999999939493 ) ;
#10857=AXIS2_PLACEMENT_3D ( 'NONE', #56051, #141699, #101244 ) ;
#10876=ADVANCED_FACE ( 'NONE', ( #59541 ), #77845, .T. ) ;
#10904=EDGE_CURVE ( 'NONE', #128875, #66482, #122127, .T. ) ;
#10954=DIRECTION ( 'NONE',  ( 0.000000000000000000, 1.734723475976817507E-14, -1.000000000000000000 ) ) ;
#11005=DIRECTION ( 'NONE',  ( -0.000000000000000000, -1.156482317317873105E-15, 1.000000000000000000 ) ) ;
#11027=STYLED_ITEM ( 'NONE', ( #144184 ), #108017 ) ;
#11082=CARTESIAN_POINT ( 'NONE',  ( 20.90000000000000213, 0.000000000000000000, 0.000000000000000000 ) ) ;
#11158=VERTEX_POINT ( 'NONE', #30747 ) ;
#11186=DIRECTION ( 'NONE',  ( -0.000000000000000000, -0.1335171055202867274, -0.9910465087640865089 ) ) ;
#11223=CARTESIAN_POINT ( 'NONE',  ( -13.40000000000000213, -11.65000000000000036, 17.60000000000000497 ) ) ;
#11249=DIRECTION ( 'NONE',  ( -0.000000000000000000, -0.000000000000000000, 1.000000000000000000 ) ) ;
#11255=ORIENTED_EDGE ( 'NONE', *, *, #236033, .T. ) ;
#11291=DIRECTION ( 'NONE',  ( 1.000000000000000000, 0.000000000000000000, 0.000000000000000000 ) ) ;
#11311=ORIENTED_EDGE ( 'NONE', *, *, #87543, .T. ) ;
#11315=EDGE_CURVE ( 'NONE', #162811, #248722, #167853, .T. ) ;
#11339=AXIS2_PLACEMENT_3D ( 'NONE', #8617, #145541, #84235 ) ;
#11346=DIRECTION ( 'NONE',  ( 0.000000000000000000, 0.000000000000000000, -1.000000000000000000 ) ) ;
#11372=ORIENTED_EDGE ( 'NONE', *, *, #75310, .T. ) ;
#11419=EDGE_CURVE ( 'NONE', #97541, #73948, #251191, .T. ) ;
#11441=AXIS2_PLACEMENT_3D ( 'NONE', #44698, #244153, #240329 ) ;
#11480=CARTESIAN_POINT ( 'NONE',  ( 19.90000000000000924, 1.249999999999999334, 22.00000000000000355 ) ) ;
#11486=DIRECTION ( 'NONE',  ( 0.000000000000000000, -0.9868171638914228216, 0.1618390714546044939 ) ) ;
#11487=CARTESIAN_POINT ( 'NONE',  ( -22.94999999999999929, 1.885425182446134107, -11.49641995933507843 ) ) ;
#11497=ADVANCED_FACE ( 'NONE', ( #216426 ), #36551, .T. ) ;
#11504=FACE_OUTER_BOUND ( 'NONE', #183244, .T. ) ;
#11522=ORIENTED_EDGE ( 'NONE', *, *, #115315, .T. ) ;
#11525=CARTESIAN_POINT ( 'NONE',  ( 19.90000000000000568, 5.488301202077012775, 16.40000000000000213 ) ) ;
#11529=EDGE_CURVE ( 'NONE', #20074, #156872, #13701, .T. ) ;
#11538=EDGE_CURVE ( 'NONE', #169297, #132306, #116065, .T. ) ;
#11570=EDGE_CURVE ( 'NONE', #155056, #142179, #209513, .T. ) ;
#11652=DIRECTION ( 'NONE',  ( 0.000000000000000000, -1.000000000000000000, 0.000000000000000000 ) ) ;
#11660=ORIENTED_EDGE ( 'NONE', *, *, #58865, .T. ) ;
#11688=ORIENTED_EDGE ( 'NONE', *, *, #84971, .T. ) ;
#11712=AXIS2_PLACEMENT_3D ( 'NONE', #104097, #144514, #1148 ) ;
#11745=DIRECTION ( 'NONE',  ( 1.000000000000000000, -0.000000000000000000, 0.000000000000000000 ) ) ;
#11811=AXIS2_PLACEMENT_3D ( 'NONE', #70802, #171206, #150323 ) ;
#11876=EDGE_CURVE ( 'NONE', #89611, #174523, #154900, .T. ) ;
#11882=EDGE_CURVE ( 'NONE', #201448, #252440, #195309, .T. ) ;
#11888=EDGE_CURVE ( 'NONE', #221991, #217842, #16657, .T. ) ;
#11896=DIRECTION ( 'NONE',  ( -1.000000000000000000, 0.000000000000000000, 0.000000000000000000 ) ) ;
#11905=ORIENTED_EDGE ( 'NONE', *, *, #114747, .T. ) ;
#11921=CYLINDRICAL_SURFACE ( 'NONE', #168739, 0.09999999999999939493 ) ;
#11936=EDGE_CURVE ( 'NONE', #172629, #99187, #72798, .T. ) ;
#11946=ORIENTED_EDGE ( 'NONE', *, *, #17270, .T. ) ;
#11958=DIRECTION ( 'NONE',  ( -1.000000000000000000, -0.000000000000000000, -0.000000000000000000 ) ) ;
#11959=ORIENTED_EDGE ( 'NONE', *, *, #84250, .F. ) ;
#11970=SPHERICAL_SURFACE ( 'NONE', #10311, 0.1000000000000000056 ) ;
#11976=EDGE_CURVE ( 'NONE', #163656, #254080, #252670, .T. ) ;
#11979=ORIENTED_EDGE ( 'NONE', *, *, #34248, .F. ) ;
#11984=EDGE_LOOP ( 'NONE', ( #34816, #148366, #187214, #80304 ) ) ;
#11999=ORIENTED_EDGE ( 'NONE', *, *, #134145, .F. ) ;
#12024=CARTESIAN_POINT ( 'NONE',  ( 18.79999999999999716, -1.311673547813416718, -7.986648289447971116 ) ) ;
#12045=ORIENTED_EDGE ( 'NONE', *, *, #117720, .T. ) ;
#12076=LINE ( 'NONE', #206401, #78413 ) ;
#12148=CARTESIAN_POINT ( 'NONE',  ( 18.59999999999999787, 11.75000000000000000, 30.09999999999999787 ) ) ;
#12157=CARTESIAN_POINT ( 'NONE',  ( 0.8999999999999995781, -9.650000000000003908, 23.40000000000000213 ) ) ;
#12203=CARTESIAN_POINT ( 'NONE',  ( -5.900000000000002132, -11.65000000000000036, 14.00000000000000178 ) ) ;
#12245=EDGE_CURVE ( 'NONE', #137004, #78394, #30843, .T. ) ;
#12264=DIRECTION ( 'NONE',  ( 0.000000000000000000, 0.000000000000000000, -1.000000000000000000 ) ) ;
#12337=DIRECTION ( 'NONE',  ( 0.000000000000000000, 0.000000000000000000, -1.000000000000000000 ) ) ;
#12364=PLANE ( 'NONE',  #60579 ) ;
#12418=ORIENTED_EDGE ( 'NONE', *, *, #2486, .F. ) ;
#12437=CARTESIAN_POINT ( 'NONE',  ( 18.59999999999999787, -11.65000000000000036, 6.100000000000001421 ) ) ;
#12454=ORIENTED_EDGE ( 'NONE', *, *, #11315, .F. ) ;
#12492=TOROIDAL_SURFACE ( 'NONE', #257929, 0.2000000000000000111, 0.1000000000000000056 ) ;
#12497=EDGE_LOOP ( 'NONE', ( #173993, #29341, #244810, #162677 ) ) ;
#12514=DIRECTION ( 'NONE',  ( 0.000000000000000000, 0.000000000000000000, -1.000000000000000000 ) ) ;
#12529=AXIS2_PLACEMENT_3D ( 'NONE', #92469, #74238, #250270 ) ;
#12624=DIRECTION ( 'NONE',  ( 0.000000000000000000, 0.000000000000000000, 1.000000000000000000 ) ) ;
#12676=ADVANCED_FACE ( 'NONE', ( #214237 ), #85129, .T. ) ;
#12728=VERTEX_POINT ( 'NONE', #12203 ) ;
#12756=VERTEX_POINT ( 'NONE', #211683 ) ;
#12788=ORIENTED_EDGE ( 'NONE', *, *, #242862, .F. ) ;
#12824=ORIENTED_EDGE ( 'NONE', *, *, #158539, .T. ) ;
#12888=ORIENTED_EDGE ( 'NONE', *, *, #103593, .T. ) ;
#12891=CARTESIAN_POINT ( 'NONE',  ( 20.90000000000000213, 8.000000000000000000, 1.212568896937007867 ) ) ;
#12945=ORIENTED_EDGE ( 'NONE', *, *, #133328, .T. ) ;
#12958=AXIS2_PLACEMENT_3D ( 'NONE', #42367, #121918, #102299 ) ;
#12989=VERTEX_POINT ( 'NONE', #227055 ) ;
#12991=ORIENTED_EDGE ( 'NONE', *, *, #172799, .F. ) ;
#13002=ORIENTED_EDGE ( 'NONE', *, *, #201292, .F. ) ;
#13058=ORIENTED_EDGE ( 'NONE', *, *, #175695, .T. ) ;
#13079=DIRECTION ( 'NONE',  ( 0.000000000000000000, -0.9910465087640866200, -0.1335171055202867274 ) ) ;
#13112=DIRECTION ( 'NONE',  ( 0.000000000000000000, 0.000000000000000000, -1.000000000000000000 ) ) ;
#13160=ADVANCED_FACE ( 'NONE', ( #16697 ), #64977, .T. ) ;
#13170=LINE ( 'NONE', #228366, #220567 ) ;
#13201=CIRCLE ( 'NONE', #121551, 0.1000000000000002554 ) ;
#13219=CIRCLE ( 'NONE', #29814, 0.09999999999999939493 ) ;
#13297=EDGE_LOOP ( 'NONE', ( #120657, #78355, #68704, #47370 ) ) ;
#13302=ORIENTED_EDGE ( 'NONE', *, *, #36304, .F. ) ;
#13311=CIRCLE ( 'NONE', #46592, 0.09999999999999993616 ) ;
#13312=DIRECTION ( 'NONE',  ( 0.000000000000000000, -0.1335171055202870327, 0.9910465087640865089 ) ) ;
#13321=ADVANCED_FACE ( 'NONE', ( #46491 ), #248553, .T. ) ;
#13342=AXIS2_PLACEMENT_3D ( 'NONE', #134185, #194195, #32571 ) ;
#13357=DIRECTION ( 'NONE',  ( 0.000000000000000000, -0.9856811345164744331, -0.1686199900910800020 ) ) ;
#13358=AXIS2_PLACEMENT_3D ( 'NONE', #128893, #88439, #247548 ) ;
#13374=CARTESIAN_POINT ( 'NONE',  ( -22.94999999999999929, 5.488301202077012775, 16.40000000000000213 ) ) ;
#13375=CYLINDRICAL_SURFACE ( 'NONE', #162195, 0.09999999999999939493 ) ;
#13384=VERTEX_POINT ( 'NONE', #171627 ) ;
#13390=CIRCLE ( 'NONE', #146622, 0.09999999999999963085 ) ;
#13394=EDGE_CURVE ( 'NONE', #209282, #152492, #222298, .T. ) ;
#13462=CIRCLE ( 'NONE', #117685, 0.09999999999999982514 ) ;
#13469=AXIS2_PLACEMENT_3D ( 'NONE', #236899, #238170, #79088 ) ;
#13504=CIRCLE ( 'NONE', #117538, 0.1999999999999987899 ) ;
#13511=DIRECTION ( 'NONE',  ( 1.000000000000000000, -0.000000000000000000, 0.000000000000000000 ) ) ;
#13593=DIRECTION ( 'NONE',  ( -1.000000000000000000, 0.000000000000000000, -0.000000000000000000 ) ) ;
#13639=EDGE_CURVE ( 'NONE', #66482, #193487, #64304, .T. ) ;
#13701=CIRCLE ( 'NONE', #159462, 0.09999999999999939493 ) ;
#13707=AXIS2_PLACEMENT_3D ( 'NONE', #143477, #108217, #63951 ) ;
#13738=DIRECTION ( 'NONE',  ( 0.000000000000000000, -0.7071067811865472397, -0.7071067811865479058 ) ) ;
#13747=DIRECTION ( 'NONE',  ( 1.000000000000000000, 0.000000000000000000, 0.000000000000000000 ) ) ;
#13795=EDGE_CURVE ( 'NONE', #49052, #40449, #55897, .T. ) ;
#13835=LINE ( 'NONE', #73836, #153931 ) ;
#13842=CARTESIAN_POINT ( 'NONE',  ( 18.79999999999999716, 11.59510167572422112, 1.901609089591594470 ) ) ;
#13853=AXIS2_PLACEMENT_3D ( 'NONE', #244330, #203927, #104792 ) ;
#13954=EDGE_CURVE ( 'NONE', #88476, #128875, #226604, .T. ) ;
#13986=ORIENTED_EDGE ( 'NONE', *, *, #131058, .F. ) ;
#14029=ORIENTED_EDGE ( 'NONE', *, *, #104167, .T. ) ;
#14051=CARTESIAN_POINT ( 'NONE',  ( 20.90000000000000213, 7.973296578895943121, -1.410778198689825347 ) ) ;
#14083=VERTEX_POINT ( 'NONE', #5118 ) ;
#14085=CIRCLE ( 'NONE', #101506, 0.09999999999999939493 ) ;
#14118=DIRECTION ( 'NONE',  ( 0.000000000000000000, -0.8741572761215355980, 0.4856429311786357172 ) ) ;
#14159=DIRECTION ( 'NONE',  ( -0.000000000000000000, -1.156482317317873105E-15, 1.000000000000000000 ) ) ;
#14170=ORIENTED_EDGE ( 'NONE', *, *, #139728, .F. ) ;
#14187=ORIENTED_EDGE ( 'NONE', *, *, #29971, .T. ) ;
#14197=DIRECTION ( 'NONE',  ( 0.000000000000000000, 1.156482317317873105E-15, -1.000000000000000000 ) ) ;
#14201=ORIENTED_EDGE ( 'NONE', *, *, #133144, .F. ) ;
#14204=CARTESIAN_POINT ( 'NONE',  ( 18.69999999999999929, 2.524878688533307880, -16.24283924587617989 ) ) ;
#14271=EDGE_CURVE ( 'NONE', #62919, #95570, #1922, .T. ) ;
#14318=CARTESIAN_POINT ( 'NONE',  ( -18.79999999999999716, -1.885425182446133885, -11.49641995933507843 ) ) ;
#14322=ORIENTED_EDGE ( 'NONE', *, *, #165214, .F. ) ;
#14336=DIRECTION ( 'NONE',  ( 0.000000000000000000, 0.000000000000000000, 1.000000000000000000 ) ) ;
#14337=ORIENTED_EDGE ( 'NONE', *, *, #230648, .F. ) ;
#14401=AXIS2_PLACEMENT_3D ( 'NONE', #140571, #242238, #220125 ) ;
#14410=DIRECTION ( 'NONE',  ( 0.000000000000000000, 0.000000000000000000, 1.000000000000000000 ) ) ;
#14424=EDGE_LOOP ( 'NONE', ( #214815, #115077, #248360, #133082 ) ) ;
#14503=EDGE_LOOP ( 'NONE', ( #225605, #195805, #159133, #98854 ) ) ;
#14509=FACE_OUTER_BOUND ( 'NONE', #94682, .T. ) ;
#14547=ORIENTED_EDGE ( 'NONE', *, *, #235614, .F. ) ;
#14556=ORIENTED_EDGE ( 'NONE', *, *, #59806, .T. ) ;
#14557=CYLINDRICAL_SURFACE ( 'NONE', #82072, 0.09999999999999939493 ) ;
#14623=CARTESIAN_POINT ( 'NONE',  ( -18.59999999999999787, -9.749999999999943157, -15.00000000000002309 ) ) ;
#14628=VECTOR ( 'NONE', #146285, 1000.000000000000000 ) ;
#14635=AXIS2_PLACEMENT_3D ( 'NONE', #43369, #82453, #162045 ) ;
#14663=EDGE_CURVE ( 'NONE', #1729, #176334, #28969, .T. ) ;
#14664=EDGE_CURVE ( 'NONE', #162415, #75205, #81211, .T. ) ;
#14671=EDGE_CURVE ( 'NONE', #129212, #144252, #163302, .T. ) ;
#14682=FACE_OUTER_BOUND ( 'NONE', #142517, .T. ) ;
#14698=ORIENTED_EDGE ( 'NONE', *, *, #23138, .T. ) ;
#14725=CIRCLE ( 'NONE', #123030, 0.1000000000000028644 ) ;
#14782=LINE ( 'NONE', #144272, #7441 ) ;
#14875=VERTEX_POINT ( 'NONE', #74508 ) ;
#14877=VECTOR ( 'NONE', #103440, 1000.000000000000000 ) ;
#14879=VECTOR ( 'NONE', #222544, 1000.000000000000000 ) ;
#14935=VERTEX_POINT ( 'NONE', #79574 ) ;
#14940=AXIS2_PLACEMENT_3D ( 'NONE', #190681, #250611, #168575 ) ;
#14968=FACE_OUTER_BOUND ( 'NONE', #254370, .T. ) ;
#15039=PLANE ( 'NONE',  #178602 ) ;
#15044=ORIENTED_EDGE ( 'NONE', *, *, #18388, .T. ) ;
#15066=CARTESIAN_POINT ( 'NONE',  ( 21.00000000000000000, 7.973296578895943121, 1.410778198689825347 ) ) ;
#15086=AXIS2_PLACEMENT_3D ( 'NONE', #248507, #37183, #249795 ) ;
#15095=DIRECTION ( 'NONE',  ( 0.000000000000000000, 0.000000000000000000, -1.000000000000000000 ) ) ;
#15109=( BOUNDED_CURVE ( )  B_SPLINE_CURVE ( 3, ( #57258, #178545, #42856, #216349 ),
 .UNSPECIFIED., .F., .F. ) 
 B_SPLINE_CURVE_WITH_KNOTS ( ( 4, 4 ),
 ( 3.141592653589793116, 4.712388980384692339 ),
 .UNSPECIFIED. ) 
 CURVE ( )  GEOMETRIC_REPRESENTATION_ITEM ( )  RATIONAL_B_SPLINE_CURVE ( ( 1.000000000000000000, 0.8047378541243643824, 0.8047378541243643824, 1.000000000000000000 ) ) 
 REPRESENTATION_ITEM ( '' )  );
#15143=ORIENTED_EDGE ( 'NONE', *, *, #199853, .F. ) ;
#15144=DIRECTION ( 'NONE',  ( -0.000000000000000000, 1.000000000000000000, -0.000000000000000000 ) ) ;
#15167=DIRECTION ( 'NONE',  ( -0.000000000000000000, 0.000000000000000000, -1.000000000000000000 ) ) ;
#15189=CARTESIAN_POINT ( 'NONE',  ( 18.69999999999999929, -10.64999999999999325, 31.39999999999999858 ) ) ;
#15202=CARTESIAN_POINT ( 'NONE',  ( -18.69999999999999929, -8.250000000000005329, -15.00000000000000000 ) ) ;
#15253=ORIENTED_EDGE ( 'NONE', *, *, #152843, .T. ) ;
#15309=FACE_OUTER_BOUND ( 'NONE', #203605, .T. ) ;
#15354=DIRECTION ( 'NONE',  ( 0.000000000000000000, 0.000000000000000000, 1.000000000000000000 ) ) ;
#15355=DIRECTION ( 'NONE',  ( 0.000000000000000000, 0.000000000000000000, -1.000000000000000000 ) ) ;
#15372=CARTESIAN_POINT ( 'NONE',  ( -21.06025298249096522, 6.342459739380975847, 12.00000000173892722 ) ) ;
#15480=ADVANCED_FACE ( 'NONE', ( #220086 ), #145664, .T. ) ;
#15482=DIRECTION ( 'NONE',  ( -1.000000000000000000, -0.000000000000000000, -0.000000000000000000 ) ) ;
#15519=VECTOR ( 'NONE', #128860, 1000.000000000000000 ) ;
#15531=FACE_OUTER_BOUND ( 'NONE', #248955, .T. ) ;
#15542=TOROIDAL_SURFACE ( 'NONE', #257073, 0.2000000000000000111, 0.1000000000000000056 ) ;
#15648=CIRCLE ( 'NONE', #107361, 0.2000000000000000944 ) ;
#15652=ORIENTED_EDGE ( 'NONE', *, *, #222922, .T. ) ;
#15660=DIRECTION ( 'NONE',  ( 0.000000000000000000, 1.000000000000000000, -0.000000000000000000 ) ) ;
#15716=AXIS2_PLACEMENT_3D ( 'NONE', #68861, #4990, #84503 ) ;
#15722=CARTESIAN_POINT ( 'NONE',  ( 18.59999999999999787, -8.150000000000007461, 32.89999999999999858 ) ) ;
#15770=VERTEX_POINT ( 'NONE', #180649 ) ;
#15824=FACE_OUTER_BOUND ( 'NONE', #23735, .T. ) ;
#15854=ORIENTED_EDGE ( 'NONE', *, *, #219217, .T. ) ;
#15872=( BOUNDED_SURFACE ( )  B_SPLINE_SURFACE ( 3, 2, ( 
 ( #123744, #115072, #237590 ),
 ( #19840, #195909, #194637 ),
 ( #203268, #58911, #96754 ),
 ( #15998, #176349, #135891 ) ),
 .UNSPECIFIED., .F., .F., .F. ) 
 B_SPLINE_SURFACE_WITH_KNOTS ( ( 4, 4 ),
 ( 3, 3 ),
 ( 0.000000000000000000, 1.570796326794896558 ),
 ( 0.000000000000000000, 1.000000000000000000 ),
 .UNSPECIFIED. ) 
 GEOMETRIC_REPRESENTATION_ITEM ( )  RATIONAL_B_SPLINE_SURFACE ( (
 ( 1.000000000000000000, 0.7644017236018784134, 1.000000000000000000),
 ( 1.000000000000000000, 0.7651312202474060964, 1.000000000000000000),
 ( 1.000000000000000000, 0.7389971855005991186, 1.000000000000000000),
 ( 1.000000000000000000, 0.7071067811865444641, 1.000000000000000000) ) ) 
 REPRESENTATION_ITEM ( '' )  SURFACE ( )  );
#15881=EDGE_CURVE ( 'NONE', #184818, #33376, #223591, .T. ) ;
#15933=ORIENTED_EDGE ( 'NONE', *, *, #11419, .F. ) ;
#15944=EDGE_CURVE ( 'NONE', #184818, #79286, #170120, .T. ) ;
#15961=ORIENTED_EDGE ( 'NONE', *, *, #198290, .T. ) ;
#15966=CARTESIAN_POINT ( 'NONE',  ( -13.40000000000000213, -8.350000000000004974, 15.00000000000000355 ) ) ;
#15998=CARTESIAN_POINT ( 'NONE',  ( -20.09999999999999787, 5.552655413246002425, 16.61686199900910310 ) ) ;
#16026=AXIS2_PLACEMENT_3D ( 'NONE', #184443, #110046, #25397 ) ;
#16050=AXIS2_PLACEMENT_3D ( 'NONE', #62857, #221905, #182838 ) ;
#16100=VECTOR ( 'NONE', #64020, 1000.000000000000000 ) ;
#16132=DIRECTION ( 'NONE',  ( -1.000000000000000000, 0.000000000000000000, 0.000000000000000000 ) ) ;
#16133=EDGE_LOOP ( 'NONE', ( #41152, #86266, #230424, #8093 ) ) ;
#16155=ADVANCED_FACE ( 'NONE', ( #179095 ), #121677, .T. ) ;
#16198=EDGE_LOOP ( 'NONE', ( #152724, #48434, #228400, #146662 ) ) ;
#16204=ORIENTED_EDGE ( 'NONE', *, *, #115386, .F. ) ;
#16207=EDGE_CURVE ( 'NONE', #120003, #97490, #69699, .T. ) ;
#16216=FACE_OUTER_BOUND ( 'NONE', #141349, .T. ) ;
#16243=AXIS2_PLACEMENT_3D ( 'NONE', #202019, #143315, #44236 ) ;
#16244=EDGE_LOOP ( 'NONE', ( #61321, #223840 ) ) ;
#16265=DIRECTION ( 'NONE',  ( 0.000000000000000000, 0.9868171638914216004, -0.1618390714546136255 ) ) ;
#16295=CARTESIAN_POINT ( 'NONE',  ( -18.60000000000000142, -8.250000000000005329, 32.89999999999999858 ) ) ;
#16315=DIRECTION ( 'NONE',  ( 1.000000000000000000, 0.000000000000000000, 0.000000000000000000 ) ) ;
#16351=DIRECTION ( 'NONE',  ( 1.000000000000000000, 0.000000000000000000, 0.000000000000000000 ) ) ;
#16353=ADVANCED_FACE ( 'NONE', ( #95037 ), #15542, .T. ) ;
#16378=DIRECTION ( 'NONE',  ( 0.000000000000000000, -1.000000000000000000, -2.081668171172166936E-15 ) ) ;
#16390=CIRCLE ( 'NONE', #20489, 11.75000000000000000 ) ;
#16403=VECTOR ( 'NONE', #116291, 1000.000000000000000 ) ;
#16433=EDGE_CURVE ( 'NONE', #254080, #162811, #20659, .T. ) ;
#16443=ADVANCED_FACE ( 'NONE', ( #155051 ), #186410, .F. ) ;
#16473=CYLINDRICAL_SURFACE ( 'NONE', #92803, 0.1000000000000028644 ) ;
#16508=EDGE_LOOP ( 'NONE', ( #246935, #73339, #81065, #98287 ) ) ;
#16531=DIRECTION ( 'NONE',  ( 1.000000000000000000, 0.000000000000000000, 0.000000000000000000 ) ) ;
#16573=ORIENTED_EDGE ( 'NONE', *, *, #118486, .T. ) ;
#16578=EDGE_CURVE ( 'NONE', #171633, #169815, #136479, .T. ) ;
#16582=CARTESIAN_POINT ( 'NONE',  ( -22.94999999999999929, -1.901609089591594692, -11.59510167572422112 ) ) ;
#16587=VECTOR ( 'NONE', #149468, 1000.000000000000000 ) ;
#16594=DIRECTION ( 'NONE',  ( 1.476360405086644309E-16, 1.000000000000000000, 0.000000000000000000 ) ) ;
#16657=LINE ( 'NONE', #250122, #184741 ) ;
#16669=EDGE_CURVE ( 'NONE', #129072, #97490, #247373, .T. ) ;
#16676=DIRECTION ( 'NONE',  ( 0.000000000000000000, 0.000000000000000000, 1.000000000000000000 ) ) ;
#16677=DIRECTION ( 'NONE',  ( -1.000000000000000000, -0.000000000000000000, -0.000000000000000000 ) ) ;
#16688=VERTEX_POINT ( 'NONE', #29657 ) ;
#16697=FACE_OUTER_BOUND ( 'NONE', #69200, .T. ) ;
#16724=DIRECTION ( 'NONE',  ( 1.000000000000000000, -1.476360405086644309E-16, 0.000000000000000000 ) ) ;
#16759=AXIS2_PLACEMENT_3D ( 'NONE', #48021, #46732, #27218 ) ;
#16767=EDGE_CURVE ( 'NONE', #145044, #176334, #57379, .T. ) ;
#16789=DIRECTION ( 'NONE',  ( 0.000000000000000000, 0.1335171055202901691, -0.9910465087640861759 ) ) ;
#16903=VERTEX_POINT ( 'NONE', #166300 ) ;
#16923=FACE_OUTER_BOUND ( 'NONE', #55468, .T. ) ;
#16930=DIRECTION ( 'NONE',  ( -1.000000000000000000, 0.000000000000000000, 0.000000000000000000 ) ) ;
#16935=AXIS2_PLACEMENT_3D ( 'NONE', #201747, #220035, #3541 ) ;
#16982=EDGE_CURVE ( 'NONE', #194417, #51689, #107640, .T. ) ;
#17018=AXIS2_PLACEMENT_3D ( 'NONE', #182977, #37372, #256329 ) ;
#17029=LINE ( 'NONE', #96522, #233441 ) ;
#17037=DIRECTION ( 'NONE',  ( 1.000000000000000000, -0.000000000000000000, 0.000000000000000000 ) ) ;
#17041=FACE_OUTER_BOUND ( 'NONE', #138564, .T. ) ;
#17096=CARTESIAN_POINT ( 'NONE',  ( 20.90000000000000213, 6.644425182197214674, 9.641788261573355001 ) ) ;
#17105=DIRECTION ( 'NONE',  ( 0.000000000000000000, 0.000000000000000000, -1.000000000000000000 ) ) ;
#17116=ADVANCED_FACE ( 'NONE', ( #202543 ), #119163, .F. ) ;
#17208=CARTESIAN_POINT ( 'NONE',  ( -18.79999999999999716, 3.461118860469513336, 28.84309995045515507 ) ) ;
#17218=AXIS2_PLACEMENT_3D ( 'NONE', #196053, #216878, #99481 ) ;
#17270=EDGE_CURVE ( 'NONE', #173345, #168528, #70070, .T. ) ;
#17319=EDGE_CURVE ( 'NONE', #216189, #31617, #12076, .T. ) ;
#17356=CARTESIAN_POINT ( 'NONE',  ( 18.79999999999999716, 11.75000000000000000, -7.800000000000000711 ) ) ;
#17370=AXIS2_PLACEMENT_3D ( 'NONE', #161654, #24717, #6398 ) ;
#17407=EDGE_CURVE ( 'NONE', #120569, #207660, #257032, .T. ) ;
#17410=DIRECTION ( 'NONE',  ( 0.000000000000000000, 1.000000000000000000, -0.000000000000000000 ) ) ;
#17413=ORIENTED_EDGE ( 'NONE', *, *, #127127, .T. ) ;
#17438=VERTEX_POINT ( 'NONE', #34213 ) ;
#17442=ORIENTED_EDGE ( 'NONE', *, *, #29178, .F. ) ;
#17463=DIRECTION ( 'NONE',  ( -0.000000000000000000, 1.000000000000000000, -0.000000000000000000 ) ) ;
#17525=CARTESIAN_POINT ( 'NONE',  ( -22.10000000000000142, -11.65000000000000036, 12.09999999999999609 ) ) ;
#17527=EDGE_CURVE ( 'NONE', #188417, #169022, #23646, .T. ) ;
#17534=FACE_OUTER_BOUND ( 'NONE', #60167, .T. ) ;
#17600=CIRCLE ( 'NONE', #159116, 0.1999999999999987899 ) ;
#17605=CIRCLE ( 'NONE', #13358, 0.09999999999999939493 ) ;
#17635=EDGE_CURVE ( 'NONE', #65906, #119824, #10471, .T. ) ;
#17645=AXIS2_PLACEMENT_3D ( 'NONE', #223811, #182143, #45185 ) ;
#17681=DIRECTION ( 'NONE',  ( 0.000000000000000000, 0.000000000000000000, 1.000000000000000000 ) ) ;
#17701=CIRCLE ( 'NONE', #163469, 0.09999999999999990841 ) ;
#17750=EDGE_CURVE ( 'NONE', #5080, #122251, #213798, .T. ) ;
#17778=CARTESIAN_POINT ( 'NONE',  ( -13.40000000000000213, -12.25000000000000178, 15.00000000000000355 ) ) ;
#17781=ORIENTED_EDGE ( 'NONE', *, *, #62343, .T. ) ;
#17788=CARTESIAN_POINT ( 'NONE',  ( 18.69999999999999929, 1.350000000000000089, 22.10000000000000142 ) ) ;
#17867=LINE ( 'NONE', #157431, #23859 ) ;
#17874=ORIENTED_EDGE ( 'NONE', *, *, #17635, .T. ) ;
#17875=CARTESIAN_POINT ( 'NONE',  ( -21.00000000000000000, 7.800000000000000711, 0.000000000000000000 ) ) ;
#17901=ORIENTED_EDGE ( 'NONE', *, *, #90739, .T. ) ;
#17903=LINE ( 'NONE', #33682, #20796 ) ;
#17912=CARTESIAN_POINT ( 'NONE',  ( -19.99999999999999645, 4.513204987021263825, 22.00000000000000355 ) ) ;
#17917=AXIS2_PLACEMENT_3D ( 'NONE', #161004, #163570, #61899 ) ;
#17927=LINE ( 'NONE', #33703, #257199 ) ;
#17955=CYLINDRICAL_SURFACE ( 'NONE', #25600, 4.000000000000000000 ) ;
#17969=LINE ( 'NONE', #192778, #201482 ) ;
#17973=VECTOR ( 'NONE', #77416, 1000.000000000000227 ) ;
#17995=EDGE_CURVE ( 'NONE', #227995, #19574, #199026, .T. ) ;
#18000=DIRECTION ( 'NONE',  ( 1.000000000000000000, 0.000000000000000000, 0.000000000000000000 ) ) ;
#18002=LINE ( 'NONE', #256567, #42699 ) ;
#18013=ORIENTED_EDGE ( 'NONE', *, *, #6288, .F. ) ;
#18036=EDGE_LOOP ( 'NONE', ( #71969, #246943, #126998, #181418 ) ) ;
#18078=ADVANCED_FACE ( 'NONE', ( #167979 ), #247476, .F. ) ;
#18109=EDGE_LOOP ( 'NONE', ( #83442, #141340, #74889 ) ) ;
#18127=ORIENTED_EDGE ( 'NONE', *, *, #173328, .T. ) ;
#18143=EDGE_LOOP ( 'NONE', ( #167267, #140934, #34819, #250659 ) ) ;
#18159=ORIENTED_EDGE ( 'NONE', *, *, #234208, .T. ) ;
#18210=AXIS2_PLACEMENT_3D ( 'NONE', #44694, #244148, #21297 ) ;
#18213=DIRECTION ( 'NONE',  ( 1.000000000000000000, 0.000000000000000000, 0.000000000000000000 ) ) ;
#18232=CARTESIAN_POINT ( 'NONE',  ( 18.79999999999999716, 1.149999999999999911, 21.90000000000000213 ) ) ;
#18234=PLANE ( 'NONE',  #242477 ) ;
#18240=EDGE_CURVE ( 'NONE', #131589, #23059, #57542, .T. ) ;
#18282=ORIENTED_EDGE ( 'NONE', *, *, #11888, .T. ) ;
#18292=CARTESIAN_POINT ( 'NONE',  ( -22.10000000000000142, -11.65000000000000036, 32.89999999999999858 ) ) ;
#18331=AXIS2_PLACEMENT_3D ( 'NONE', #232873, #55455, #15095 ) ;
#18345=VERTEX_POINT ( 'NONE', #127224 ) ;
#18388=EDGE_CURVE ( 'NONE', #252739, #79944, #63379, .T. ) ;
#18468=CIRCLE ( 'NONE', #14401, 4.041421356237306917 ) ;
#18475=FACE_OUTER_BOUND ( 'NONE', #7659, .T. ) ;
#18477=DIRECTION ( 'NONE',  ( 0.000000000000000000, 0.000000000000000000, -1.000000000000000000 ) ) ;
#18516=ORIENTED_EDGE ( 'NONE', *, *, #133655, .F. ) ;
#18539=ADVANCED_FACE ( 'NONE', ( #95774 ), #57933, .T. ) ;
#18565=DIRECTION ( 'NONE',  ( 1.000000000000000000, 0.000000000000000000, 0.000000000000000000 ) ) ;
#18596=DIRECTION ( 'NONE',  ( 0.000000000000000000, 1.000000000000000000, 0.000000000000000000 ) ) ;
#18617=CARTESIAN_POINT ( 'NONE',  ( -18.79999999999999716, 1.885425182446137438, -11.49641995933507843 ) ) ;
#18635=ORIENTED_EDGE ( 'NONE', *, *, #117869, .F. ) ;
#18658=DIRECTION ( 'NONE',  ( 0.000000000000000000, 0.000000000000000000, 1.000000000000000000 ) ) ;
#18686=FACE_OUTER_BOUND ( 'NONE', #94763, .T. ) ;
#18688=CARTESIAN_POINT ( 'NONE',  ( 5.899999999999997691, -11.25000000000000000, 13.90000000000000213 ) ) ;
#18693=AXIS2_PLACEMENT_3D ( 'NONE', #75429, #16724, #96232 ) ;
#18734=ORIENTED_EDGE ( 'NONE', *, *, #139777, .T. ) ;
#18756=ADVANCED_FACE ( 'NONE', ( #97712 ), #234692, .T. ) ;
#18783=ADVANCED_FACE ( 'NONE', ( #96437 ), #120337, .T. ) ;
#18890=DIRECTION ( 'NONE',  ( 0.000000000000000000, 0.9856811345164832039, 0.1686199900910280158 ) ) ;
#18902=ORIENTED_EDGE ( 'NONE', *, *, #59822, .T. ) ;
#18910=CARTESIAN_POINT ( 'NONE',  ( 20.89999999999999858, -11.65000000000000036, 11.89999999999999680 ) ) ;
#18914=DIRECTION ( 'NONE',  ( -1.476360405086644309E-16, 1.000000000000000000, -0.000000000000000000 ) ) ;
#18915=CARTESIAN_POINT ( 'NONE',  ( -21.00000000000000000, 0.000000000000000000, 0.000000000000000000 ) ) ;
#18932=VERTEX_POINT ( 'NONE', #218964 ) ;
#18940=EDGE_LOOP ( 'NONE', ( #84965, #239730, #165000, #251265 ) ) ;
#18943=EDGE_CURVE ( 'NONE', #36331, #108582, #5031, .T. ) ;
#18949=EDGE_LOOP ( 'NONE', ( #100185, #247221, #47829, #251205 ) ) ;
#18951=ORIENTED_EDGE ( 'NONE', *, *, #44673, .F. ) ;
#18967=ORIENTED_EDGE ( 'NONE', *, *, #105931, .T. ) ;
#18975=AXIS2_PLACEMENT_3D ( 'NONE', #75948, #77213, #3792 ) ;
#18977=DIRECTION ( 'NONE',  ( 0.000000000000000000, -1.000000000000000000, -1.445602896647339410E-16 ) ) ;
#19008=AXIS2_PLACEMENT_3D ( 'NONE', #76998, #193111, #93985 ) ;
#19074=AXIS2_PLACEMENT_3D ( 'NONE', #51509, #230175, #74986 ) ;
#19077=CYLINDRICAL_SURFACE ( 'NONE', #61509, 0.09999999999999939493 ) ;
#19107=LINE ( 'NONE', #81612, #1526 ) ;
#19135=CARTESIAN_POINT ( 'NONE',  ( 22.19999999999999929, -11.75000000000000000, -15.00000000000000000 ) ) ;
#19161=ORIENTED_EDGE ( 'NONE', *, *, #215541, .T. ) ;
#19177=VECTOR ( 'NONE', #170491, 1000.000000000000000 ) ;
#19278=ORIENTED_EDGE ( 'NONE', *, *, #101176, .T. ) ;
#19285=DIRECTION ( 'NONE',  ( -1.000000000000000000, 0.000000000000000000, 0.000000000000000000 ) ) ;
#19304=CARTESIAN_POINT ( 'NONE',  ( -11.60000000000000320, -11.65000000000000036, 17.60000000000000497 ) ) ;
#19322=DIRECTION ( 'NONE',  ( -1.000000000000000000, 0.000000000000000000, 0.000000000000000000 ) ) ;
#19437=ORIENTED_EDGE ( 'NONE', *, *, #50449, .T. ) ;
#19532=EDGE_LOOP ( 'NONE', ( #33983, #125396, #11979, #55453 ) ) ;
#19545=CARTESIAN_POINT ( 'NONE',  ( -19.89999999999999858, 1.250000000000000000, 22.00000000000000355 ) ) ;
#19574=VERTEX_POINT ( 'NONE', #213200 ) ;
#19608=DIRECTION ( 'NONE',  ( 1.000000000000000000, -0.000000000000000000, 0.000000000000000000 ) ) ;
#19609=ADVANCED_FACE ( 'NONE', ( #76261 ), #78816, .T. ) ;
#19735=ORIENTED_EDGE ( 'NONE', *, *, #211857, .F. ) ;
#19762=CARTESIAN_POINT ( 'NONE',  ( -13.40000000000000213, -11.65000000000000036, 12.40000000000000391 ) ) ;
#19801=ADVANCED_FACE ( 'NONE', ( #46128 ), #183092, .F. ) ;
#19811=VECTOR ( 'NONE', #252968, 1000.000000000000000 ) ;
#19840=CARTESIAN_POINT ( 'NONE',  ( -20.00894256274684579, 5.586869314946281584, 16.41686200241345261 ) ) ;
#19897=ORIENTED_EDGE ( 'NONE', *, *, #36092, .T. ) ;
#19960=DIRECTION ( 'NONE',  ( 1.000000000000000000, 0.000000000000000000, 0.000000000000000000 ) ) ;
#19964=CARTESIAN_POINT ( 'NONE',  ( -22.94999999999999929, -11.75000000000000178, 0.000000000000000000 ) ) ;
#19969=AXIS2_PLACEMENT_3D ( 'NONE', #153206, #232727, #133600 ) ;
#19980=VECTOR ( 'NONE', #96398, 1000.000000000000000 ) ;
#19994=CYLINDRICAL_SURFACE ( 'NONE', #17218, 0.09999999999999939493 ) ;
#20002=ADVANCED_FACE ( 'NONE', ( #56391 ), #79797, .T. ) ;
#20010=DIRECTION ( 'NONE',  ( 0.000000000000000000, 0.000000000000000000, -1.000000000000000000 ) ) ;
#20023=EDGE_CURVE ( 'NONE', #168244, #103469, #175126, .T. ) ;
#20074=VERTEX_POINT ( 'NONE', #40737 ) ;
#20157=AXIS2_PLACEMENT_3D ( 'NONE', #60811, #200345, #42540 ) ;
#20162=LINE ( 'NONE', #1843, #55145 ) ;
#20173=DIRECTION ( 'NONE',  ( 0.000000000000000000, 0.9856811345164829818, 0.1686199900910294314 ) ) ;
#20174=AXIS2_PLACEMENT_3D ( 'NONE', #9750, #29365, #89280 ) ;
#20180=DIRECTION ( 'NONE',  ( 1.000000000000000000, -0.000000000000000000, 0.000000000000000000 ) ) ;
#20216=DIRECTION ( 'NONE',  ( 0.000000000000000000, 0.000000000000000000, 1.000000000000000000 ) ) ;
#20242=AXIS2_PLACEMENT_3D ( 'NONE', #5432, #245369, #206233 ) ;
#20299=VECTOR ( 'NONE', #267, 1000.000000000000000 ) ;
#20332=ORIENTED_EDGE ( 'NONE', *, *, #163347, .F. ) ;
#20401=CARTESIAN_POINT ( 'NONE',  ( 21.00000000000000000, 1.885425182446133885, -11.49641995933507843 ) ) ;
#20406=EDGE_CURVE ( 'NONE', #108582, #247506, #166651, .T. ) ;
#20429=AXIS2_PLACEMENT_3D ( 'NONE', #211271, #16930, #172193 ) ;
#20434=ORIENTED_EDGE ( 'NONE', *, *, #229921, .T. ) ;
#20446=CARTESIAN_POINT ( 'NONE',  ( -18.59999999999999787, -11.65000000000000036, 29.89999999999999858 ) ) ;
#20458=CARTESIAN_POINT ( 'NONE',  ( -0.8999999999999991340, -9.650000000000003908, 23.40000000000000213 ) ) ;
#20471=DIRECTION ( 'NONE',  ( 0.000000000000000000, 0.1335171055202867274, -0.9910465087640866200 ) ) ;
#20475=ADVANCED_FACE ( 'NONE', ( #114345 ), #72676, .T. ) ;
#20489=AXIS2_PLACEMENT_3D ( 'NONE', #172493, #73371, #233712 ) ;
#20492=VECTOR ( 'NONE', #131473, 1000.000000000000000 ) ;
#20593=ORIENTED_EDGE ( 'NONE', *, *, #172732, .T. ) ;
#20640=DIRECTION ( 'NONE',  ( 1.000000000000000000, -0.000000000000000000, -0.000000000000000000 ) ) ;
#20655=EDGE_CURVE ( 'NONE', #158566, #5080, #136642, .T. ) ;
#20659=LINE ( 'NONE', #157627, #61313 ) ;
#20708=DIRECTION ( 'NONE',  ( -0.000000000000000000, -0.1335171055202864221, -0.9910465087640866200 ) ) ;
#20742=CIRCLE ( 'NONE', #216529, 0.09999999999999939493 ) ;
#20752=DIRECTION ( 'NONE',  ( -1.000000000000000000, 0.000000000000000000, 0.000000000000000000 ) ) ;
#20791=CARTESIAN_POINT ( 'NONE',  ( -18.69999999999999929, 6.841561409100513025, 9.675512259591560138 ) ) ;
#20795=EDGE_LOOP ( 'NONE', ( #52094, #134652, #183435, #229665 ) ) ;
#20796=VECTOR ( 'NONE', #97416, 1000.000000000000000 ) ;
#20849=FACE_OUTER_BOUND ( 'NONE', #123880, .T. ) ;
#20857=ORIENTED_EDGE ( 'NONE', *, *, #193902, .T. ) ;
#20858=EDGE_LOOP ( 'NONE', ( #102424, #24838, #211377, #184603 ) ) ;
#20859=VECTOR ( 'NONE', #119664, 1000.000000000000114 ) ;
#20889=CARTESIAN_POINT ( 'NONE',  ( 18.79999999999999005, 1.212568896937007645, -8.000000000000000000 ) ) ;
#20918=EDGE_CURVE ( 'NONE', #5568, #691, #161809, .T. ) ;
#20930=TOROIDAL_SURFACE ( 'NONE', #154225, 0.2000000000000000111, 0.1000000000000000056 ) ;
#20953=CARTESIAN_POINT ( 'NONE',  ( -18.60000000000000142, -8.250000000000005329, 33.00000000000000000 ) ) ;
#20955=FACE_OUTER_BOUND ( 'NONE', #234031, .T. ) ;
#21010=DIRECTION ( 'NONE',  ( 0.000000000000000000, 0.000000000000000000, 1.000000000000000000 ) ) ;
#21059=DIRECTION ( 'NONE',  ( 0.000000000000000000, 0.000000000000000000, 1.000000000000000000 ) ) ;
#21094=LINE ( 'NONE', #83569, #250090 ) ;
#21157=CARTESIAN_POINT ( 'NONE',  ( -11.60000000000000320, -8.250000000000007105, 17.60000000000000497 ) ) ;
#21163=EDGE_CURVE ( 'NONE', #27371, #239767, #58121, .T. ) ;
#21213=ORIENTED_EDGE ( 'NONE', *, *, #228397, .F. ) ;
#21241=AXIS2_PLACEMENT_3D ( 'NONE', #30959, #206998, #107889 ) ;
#21297=DIRECTION ( 'NONE',  ( 0.000000000000000000, 0.000000000000000000, -1.000000000000000000 ) ) ;
#21334=DIRECTION ( 'NONE',  ( 0.000000000000000000, 0.000000000000000000, -1.000000000000000000 ) ) ;
#21336=ORIENTED_EDGE ( 'NONE', *, *, #251827, .F. ) ;
#21337=CIRCLE ( 'NONE', #12958, 0.09999999999999982514 ) ;
#21356=CARTESIAN_POINT ( 'NONE',  ( 5.899999999999997691, -11.34999999999999964, 13.90000000000000213 ) ) ;
#21399=VECTOR ( 'NONE', #19608, 1000.000000000000000 ) ;
#21409=ORIENTED_EDGE ( 'NONE', *, *, #134162, .T. ) ;
#21470=DIRECTION ( 'NONE',  ( 0.000000000000000000, 0.000000000000000000, -1.000000000000000000 ) ) ;
#21477=EDGE_CURVE ( 'NONE', #164655, #89756, #174099, .T. ) ;
#21478=DIRECTION ( 'NONE',  ( 0.000000000000000000, 0.000000000000000000, -1.000000000000000000 ) ) ;
#21551=CARTESIAN_POINT ( 'NONE',  ( 18.79999999999999716, 11.49641995933507665, -1.885425182446133663 ) ) ;
#21568=AXIS2_PLACEMENT_3D ( 'NONE', #235465, #157255, #232939 ) ;
#21606=ORIENTED_EDGE ( 'NONE', *, *, #224601, .F. ) ;
#21610=CARTESIAN_POINT ( 'NONE',  ( 20.90000000000000213, -1.885425182446133885, -11.49641995933507843 ) ) ;
#21648=ORIENTED_EDGE ( 'NONE', *, *, #252186, .T. ) ;
#21656=ADVANCED_FACE ( 'NONE', ( #207651 ), #86541, .T. ) ;
#21662=ORIENTED_EDGE ( 'NONE', *, *, #120871, .F. ) ;
#21663=VERTEX_POINT ( 'NONE', #205036 ) ;
#21695=DIRECTION ( 'NONE',  ( 0.000000000000000000, -1.000000000000000000, -0.000000000000000000 ) ) ;
#21727=CARTESIAN_POINT ( 'NONE',  ( 18.59999999999999787, -11.65000000000000036, 5.900000000000001243 ) ) ;
#21778=AXIS2_PLACEMENT_3D ( 'NONE', #11525, #71509, #151030 ) ;
#21784=LINE ( 'NONE', #84248, #166542 ) ;
#21787=DIRECTION ( 'NONE',  ( 0.000000000000000000, 0.000000000000000000, 1.000000000000000000 ) ) ;
#21811=CARTESIAN_POINT ( 'NONE',  ( -18.69999999999999929, -10.80884033489985363, 5.900000000000001243 ) ) ;
#21832=VECTOR ( 'NONE', #27190, 1000.000000000000000 ) ;
#21894=ADVANCED_FACE ( 'NONE', ( #195796 ), #144997, .T. ) ;
#21933=DIRECTION ( 'NONE',  ( 1.000000000000000000, -0.000000000000000000, -0.000000000000000000 ) ) ;
#22004=DIRECTION ( 'NONE',  ( -1.000000000000000000, -0.000000000000000000, -0.000000000000000000 ) ) ;
#22005=ORIENTED_EDGE ( 'NONE', *, *, #167827, .F. ) ;
#22035=LINE ( 'NONE', #24616, #21832 ) ;
#22076=( BOUNDED_CURVE ( )  B_SPLINE_CURVE ( 3, ( #218215, #113995, #134824, #235235 ),
 .UNSPECIFIED., .F., .T. ) 
 B_SPLINE_CURVE_WITH_KNOTS ( ( 4, 4 ),
 ( 4.712388980384695003, 6.283185307179586232 ),
 .UNSPECIFIED. ) 
 CURVE ( )  GEOMETRIC_REPRESENTATION_ITEM ( )  RATIONAL_B_SPLINE_CURVE ( ( 1.000000000000000000, 0.8047378541243662697, 0.8047378541243662697, 1.000000000000000000 ) ) 
 REPRESENTATION_ITEM ( '' )  );
#22108=ORIENTED_EDGE ( 'NONE', *, *, #158899, .T. ) ;
#22117=VERTEX_POINT ( 'NONE', #177668 ) ;
#22128=DIRECTION ( 'NONE',  ( -0.000000000000000000, -0.1335171055202901413, -0.9910465087640860649 ) ) ;
#22186=VERTEX_POINT ( 'NONE', #201047 ) ;
#22196=DIRECTION ( 'NONE',  ( 2.895190717381441586E-16, -0.9910465087640865089, 0.1335171055202867274 ) ) ;
#22251=CIRCLE ( 'NONE', #168025, 2.699999999999999289 ) ;
#22334=LINE ( 'NONE', #176271, #189450 ) ;
#22396=CARTESIAN_POINT ( 'NONE',  ( -22.19999999999999929, -11.64999999999999858, 11.99999999999999645 ) ) ;
#22399=CARTESIAN_POINT ( 'NONE',  ( 20.90000000000000213, -1.885425182446133885, -11.49641995933507843 ) ) ;
#22402=VERTEX_POINT ( 'NONE', #228324 ) ;
#22488=CIRCLE ( 'NONE', #205603, 0.2000000000000005107 ) ;
#22514=ADVANCED_FACE ( 'NONE', ( #56072 ), #135618, .F. ) ;
#22529=CARTESIAN_POINT ( 'NONE',  ( -18.69999999999999929, 2.168342339202988800, -13.59640602015278432 ) ) ;
#22552=VECTOR ( 'NONE', #157377, 1000.000000000000000 ) ;
#22561=ORIENTED_EDGE ( 'NONE', *, *, #201304, .F. ) ;
#22573=ADVANCED_FACE ( 'NONE', ( #20849 ), #174812, .F. ) ;
#22597=CIRCLE ( 'NONE', #151603, 0.09999999999999939493 ) ;
#22619=EDGE_CURVE ( 'NONE', #246378, #189583, #7692, .T. ) ;
#22636=CARTESIAN_POINT ( 'NONE',  ( 20.00000000000000711, 4.547418889303921574, 21.90000000000000213 ) ) ;
#22638=CIRCLE ( 'NONE', #10149, 3.970710678118653636 ) ;
#22639=CARTESIAN_POINT ( 'NONE',  ( -19.89999999999999858, 1.250000000000000000, 16.60000000000000142 ) ) ;
#22680=CARTESIAN_POINT ( 'NONE',  ( 13.40000000000000036, -8.279289321881350361, 18.97071067811865674 ) ) ;
#22797=FACE_OUTER_BOUND ( 'NONE', #99224, .T. ) ;
#22836=DIRECTION ( 'NONE',  ( 0.000000000000000000, -1.000000000000000000, 0.000000000000000000 ) ) ;
#22866=ORIENTED_EDGE ( 'NONE', *, *, #32888, .F. ) ;
#22867=VECTOR ( 'NONE', #233016, 1000.000000000000114 ) ;
#22879=ORIENTED_EDGE ( 'NONE', *, *, #151809, .T. ) ;
#22899=DIRECTION ( 'NONE',  ( 0.000000000000000000, -0.8164989248600462712, 0.5773469543544753613 ) ) ;
#22914=ORIENTED_EDGE ( 'NONE', *, *, #216849, .F. ) ;
#22928=ADVANCED_FACE ( 'NONE', ( #178331 ), #199152, .T. ) ;
#22949=CIRCLE ( 'NONE', #243495, 0.09999999999999939493 ) ;
#22965=ORIENTED_EDGE ( 'NONE', *, *, #94487, .T. ) ;
#23030=CARTESIAN_POINT ( 'NONE',  ( -18.79999999999999716, -1.901609089591594470, -11.59510167572422112 ) ) ;
#23042=DIRECTION ( 'NONE',  ( 0.000000000000000000, 0.1335171055202901413, 0.9910465087640860649 ) ) ;
#23059=VERTEX_POINT ( 'NONE', #140445 ) ;
#23125=FACE_OUTER_BOUND ( 'NONE', #6447, .T. ) ;
#23138=EDGE_CURVE ( 'NONE', #45997, #128875, #33178, .T. ) ;
#23145=CARTESIAN_POINT ( 'NONE',  ( -22.94999999999999929, -1.467286812112899463, 33.00000000000000000 ) ) ;
#23162=EDGE_CURVE ( 'NONE', #190881, #62787, #248541, .T. ) ;
#23199=DIRECTION ( 'NONE',  ( -1.000000000000000000, 0.000000000000000000, -0.000000000000000000 ) ) ;
#23239=AXIS2_PLACEMENT_3D ( 'NONE', #104760, #184321, #164776 ) ;
#23246=EDGE_CURVE ( 'NONE', #219544, #140091, #252375, .T. ) ;
#23270=EDGE_LOOP ( 'NONE', ( #133120, #39655, #110593 ) ) ;
#23281=CARTESIAN_POINT ( 'NONE',  ( 19.90000000000000924, 1.350000000000000089, 22.00000000000000355 ) ) ;
#23309=CARTESIAN_POINT ( 'NONE',  ( -22.10000000000000142, -11.75000000000000000, -15.00000000000000000 ) ) ;
#23390=DIRECTION ( 'NONE',  ( 0.000000000000000000, 0.000000000000000000, 1.000000000000000000 ) ) ;
#23418=CYLINDRICAL_SURFACE ( 'NONE', #136235, 11.75000000000000000 ) ;
#23450=AXIS2_PLACEMENT_3D ( 'NONE', #47023, #206123, #13079 ) ;
#23525=DIRECTION ( 'NONE',  ( 0.000000000000000000, -0.9910465087640861759, 0.1335171055202901691 ) ) ;
#23569=ORIENTED_EDGE ( 'NONE', *, *, #112902, .T. ) ;
#23596=EDGE_LOOP ( 'NONE', ( #75673, #89368, #212440, #165551 ) ) ;
#23609=DIRECTION ( 'NONE',  ( 0.000000000000000000, -0.1335171055202901413, 0.9910465087640860649 ) ) ;
#23633=CARTESIAN_POINT ( 'NONE',  ( 20.90000000000000213, 1.786320531569725478, -11.50977166988710820 ) ) ;
#23646=LINE ( 'NONE', #2743, #16100 ) ;
#23653=CYLINDRICAL_SURFACE ( 'NONE', #162578, 0.09999999999999939493 ) ;
#23683=EDGE_CURVE ( 'NONE', #71927, #107433, #17029, .T. ) ;
#23728=LINE ( 'NONE', #104480, #228514 ) ;
#23735=EDGE_LOOP ( 'NONE', ( #58433, #167495, #115406, #215906 ) ) ;
#23802=EDGE_CURVE ( 'NONE', #90690, #82095, #172554, .T. ) ;
#23808=CARTESIAN_POINT ( 'NONE',  ( 5.899999999999995914, -11.25000000000000000, 10.10000000000000142 ) ) ;
#23852=ORIENTED_EDGE ( 'NONE', *, *, #172448, .F. ) ;
#23859=VECTOR ( 'NONE', #199086, 1000.000000000000000 ) ;
#23886=CARTESIAN_POINT ( 'NONE',  ( 18.69999999999999929, 11.49641995933507843, -1.885425182446135661 ) ) ;
#23890=VERTEX_POINT ( 'NONE', #27679 ) ;
#23951=CARTESIAN_POINT ( 'NONE',  ( -0.8999999999999993561, -8.250000000000005329, 28.60000000000000142 ) ) ;
#24096=EDGE_CURVE ( 'NONE', #14875, #139556, #137709, .T. ) ;
#24122=VECTOR ( 'NONE', #207861, 1000.000000000000114 ) ;
#24143=ORIENTED_EDGE ( 'NONE', *, *, #101636, .F. ) ;
#24221=CARTESIAN_POINT ( 'NONE',  ( 18.79999999999999716, 7.986648289447971116, 1.311673547813416718 ) ) ;
#24226=ORIENTED_EDGE ( 'NONE', *, *, #157505, .F. ) ;
#24234=EDGE_LOOP ( 'NONE', ( #39587, #32908, #79339, #126250 ) ) ;
#24251=CARTESIAN_POINT ( 'NONE',  ( 18.69999999999999929, 1.212568896937007645, -8.000000000000000000 ) ) ;
#24285=AXIS2_PLACEMENT_3D ( 'NONE', #41173, #140218, #101060 ) ;
#24308=FACE_OUTER_BOUND ( 'NONE', #71397, .T. ) ;
#24337=ORIENTED_EDGE ( 'NONE', *, *, #217303, .F. ) ;
#24357=LINE ( 'NONE', #119606, #71040 ) ;
#24467=LINE ( 'NONE', #103947, #196135 ) ;
#24493=DIRECTION ( 'NONE',  ( 1.000000000000000000, -0.000000000000000000, -0.000000000000000000 ) ) ;
#24506=ORIENTED_EDGE ( 'NONE', *, *, #30944, .T. ) ;
#24562=CYLINDRICAL_SURFACE ( 'NONE', #185157, 0.09999999999999939493 ) ;
#24572=ORIENTED_EDGE ( 'NONE', *, *, #33837, .T. ) ;
#24594=CARTESIAN_POINT ( 'NONE',  ( 22.10000000000000142, -11.65000000000000036, 12.09999999999999609 ) ) ;
#24599=CARTESIAN_POINT ( 'NONE',  ( -22.94999999999999929, 11.50977166988710820, -1.786320531569725478 ) ) ;
#24616=CARTESIAN_POINT ( 'NONE',  ( -21.00000000000000000, 7.900000000000000355, -1.212568896937008089 ) ) ;
#24676=CARTESIAN_POINT ( 'NONE',  ( 0.8999999999999993561, -8.250000000000005329, 26.00000000000000355 ) ) ;
#24694=ORIENTED_EDGE ( 'NONE', *, *, #14664, .F. ) ;
#24717=DIRECTION ( 'NONE',  ( -0.000000000000000000, 1.000000000000000000, -0.000000000000000000 ) ) ;
#24756=AXIS2_PLACEMENT_3D ( 'NONE', #251452, #74135, #191516 ) ;
#24781=DIRECTION ( 'NONE',  ( 0.000000000000000000, 0.000000000000000000, -1.000000000000000000 ) ) ;
#24823=LINE ( 'NONE', #72593, #134799 ) ;
#24837=CARTESIAN_POINT ( 'NONE',  ( -20.90000000000000213, 6.356682116888462630, 11.91686199900910381 ) ) ;
#24838=ORIENTED_EDGE ( 'NONE', *, *, #219789, .T. ) ;
#24867=AXIS2_PLACEMENT_3D ( 'NONE', #157541, #80485, #76665 ) ;
#24887=CARTESIAN_POINT ( 'NONE',  ( 18.69999999999999574, -9.749999999999994671, 30.09999999999999076 ) ) ;
#24896=ORIENTED_EDGE ( 'NONE', *, *, #17750, .F. ) ;
#24924=EDGE_CURVE ( 'NONE', #27371, #155708, #192838, .T. ) ;
#24934=FACE_OUTER_BOUND ( 'NONE', #175623, .T. ) ;
#24951=CARTESIAN_POINT ( 'NONE',  ( -22.94999999999999929, 1.786320531569725478, -11.50977166988710820 ) ) ;
#24968=SPHERICAL_SURFACE ( 'NONE', #180507, 0.1000000000000000056 ) ;
#24973=TOROIDAL_SURFACE ( 'NONE', #174844, 11.65000000000000036, 0.1000000000000000056 ) ;
#25019=SPHERICAL_SURFACE ( 'NONE', #57613, 0.1000000000000000056 ) ;
#25043=EDGE_CURVE ( 'NONE', #160911, #31617, #109784, .T. ) ;
#25050=CARTESIAN_POINT ( 'NONE',  ( -18.59999999999999787, -10.64999999999999325, 32.89999999999999858 ) ) ;
#25065=CARTESIAN_POINT ( 'NONE',  ( 18.79999999999999716, -1.212568896937008089, -7.900000000000000355 ) ) ;
#25084=ORIENTED_EDGE ( 'NONE', *, *, #83187, .F. ) ;
#25089=DIRECTION ( 'NONE',  ( 0.000000000000000000, 0.000000000000000000, -1.000000000000000000 ) ) ;
#25125=LINE ( 'NONE', #189003, #192981 ) ;
#25146=CARTESIAN_POINT ( 'NONE',  ( -18.79999999999999716, -8.150000000000005684, 33.00000000000000000 ) ) ;
#25188=AXIS2_PLACEMENT_3D ( 'NONE', #43720, #22899, #166271 ) ;
#25203=CARTESIAN_POINT ( 'NONE',  ( -18.79999999999999716, 0.000000000000000000, 32.89999999999999858 ) ) ;
#25242=DIRECTION ( 'NONE',  ( 0.000000000000000000, -1.000000000000000000, 0.000000000000000000 ) ) ;
#25273=ORIENTED_EDGE ( 'NONE', *, *, #10052, .T. ) ;
#25305=CIRCLE ( 'NONE', #171083, 0.1999999999999996503 ) ;
#25320=DIRECTION ( 'NONE',  ( 0.000000000000000000, 0.1686199900910313187, -0.9856811345164828708 ) ) ;
#25323=DIRECTION ( 'NONE',  ( -2.489438768765009500E-17, 0.1686199900910313187, -0.9856811345164828708 ) ) ;
#25338=VECTOR ( 'NONE', #226655, 1000.000000000000000 ) ;
#25343=EDGE_CURVE ( 'NONE', #190169, #158009, #130641, .T. ) ;
#25349=AXIS2_PLACEMENT_3D ( 'NONE', #92500, #149938, #251577 ) ;
#25360=VERTEX_POINT ( 'NONE', #4815 ) ;
#25377=VERTEX_POINT ( 'NONE', #60958 ) ;
#25386=AXIS2_PLACEMENT_3D ( 'NONE', #90258, #224640, #165997 ) ;
#25397=DIRECTION ( 'NONE',  ( 0.000000000000000000, 0.000000000000000000, -1.000000000000000000 ) ) ;
#25472=ORIENTED_EDGE ( 'NONE', *, *, #185533, .T. ) ;
#25479=DIRECTION ( 'NONE',  ( 0.000000000000000000, -1.224646799147358384E-16, 1.000000000000000000 ) ) ;
#25525=ADVANCED_FACE ( 'NONE', ( #88200 ), #109975, .F. ) ;
#25562=AXIS2_PLACEMENT_3D ( 'NONE', #79030, #98578, #97303 ) ;
#25566=CONICAL_SURFACE ( 'NONE', #17370, 4.000000000000000000, 0.7853981633974489451 ) ;
#25584=ORIENTED_EDGE ( 'NONE', *, *, #115315, .F. ) ;
#25593=CARTESIAN_POINT ( 'NONE',  ( -22.94999999999999929, -1.800000000000000044, -11.61130914238355771 ) ) ;
#25600=AXIS2_PLACEMENT_3D ( 'NONE', #97471, #195350, #152373 ) ;
#25625=CARTESIAN_POINT ( 'NONE',  ( 20.90000000000000213, -1.212568896937008089, -7.900000000000000355 ) ) ;
#25642=CARTESIAN_POINT ( 'NONE',  ( -18.59999999999999787, -14.27107483842559610, -0.5438473119858301397 ) ) ;
#25681=DIRECTION ( 'NONE',  ( 0.000000000000000000, 0.9910465087640861759, -0.1335171055202901691 ) ) ;
#25719=ADVANCED_FACE ( 'NONE', ( #180502 ), #160947, .T. ) ;
#25734=DIRECTION ( 'NONE',  ( 0.000000000000000000, -0.9910465087640860649, 0.1335171055202901413 ) ) ;
#25749=PLANE ( 'NONE',  #214312 ) ;
#25758=LINE ( 'NONE', #105250, #35623 ) ;
#25791=DIRECTION ( 'NONE',  ( 0.000000000000000000, 0.000000000000000000, 1.000000000000000000 ) ) ;
#25823=ADVANCED_FACE ( 'NONE', ( #250730 ), #188700, .T. ) ;
#25875=AXIS2_PLACEMENT_3D ( 'NONE', #128899, #127613, #207154 ) ;
#25884=CARTESIAN_POINT ( 'NONE',  ( 22.94999999999999929, 0.000000000000000000, 0.000000000000000000 ) ) ;
#25912=FACE_OUTER_BOUND ( 'NONE', #157589, .T. ) ;
#25927=DIRECTION ( 'NONE',  ( 0.000000000000000000, -1.000000000000000000, 0.000000000000000000 ) ) ;
#25963=CARTESIAN_POINT ( 'NONE',  ( 22.10000000000000497, 10.21702379168713115, -11.24211197275198160 ) ) ;
#26033=AXIS2_PLACEMENT_3D ( 'NONE', #119835, #40312, #58533 ) ;
#26143=ORIENTED_EDGE ( 'NONE', *, *, #36546, .F. ) ;
#26164=DIRECTION ( 'NONE',  ( 0.000000000000000000, 1.000000000000000000, 0.000000000000000000 ) ) ;
#26190=ADVANCED_FACE ( 'NONE', ( #77878 ), #76447, .T. ) ;
#26211=DIRECTION ( 'NONE',  ( 0.000000000000000000, 0.000000000000000000, 1.000000000000000000 ) ) ;
#26216=DIRECTION ( 'NONE',  ( 0.000000000000000000, -1.000000000000000000, 0.000000000000000000 ) ) ;
#26259=CARTESIAN_POINT ( 'NONE',  ( -18.79999999999999716, 8.000000000000000000, -1.212568896937008089 ) ) ;
#26263=AXIS2_PLACEMENT_3D ( 'NONE', #206115, #27520, #106995 ) ;
#26281=ORIENTED_EDGE ( 'NONE', *, *, #194516, .F. ) ;
#26292=FACE_OUTER_BOUND ( 'NONE', #13297, .T. ) ;
#26293=EDGE_CURVE ( 'NONE', #95570, #99741, #255186, .T. ) ;
#26312=VECTOR ( 'NONE', #212509, 1000.000000000000000 ) ;
#26357=CARTESIAN_POINT ( 'NONE',  ( -19.95447128016622429, 4.513204987603615770, 22.00000000000000355 ) ) ;
#26429=ORIENTED_EDGE ( 'NONE', *, *, #96420, .T. ) ;
#26430=CARTESIAN_POINT ( 'NONE',  ( 18.79999999999999716, -11.65000000000000036, 33.00000000000000000 ) ) ;
#26431=DIRECTION ( 'NONE',  ( 1.000000000000000000, 0.000000000000000000, 0.000000000000000000 ) ) ;
#26451=ORIENTED_EDGE ( 'NONE', *, *, #209548, .T. ) ;
#26465=CARTESIAN_POINT ( 'NONE',  ( 18.79999999999999716, 1.311673547813416718, -7.986648289447971116 ) ) ;
#26472=CYLINDRICAL_SURFACE ( 'NONE', #118368, 0.09999999999999939493 ) ;
#26479=CARTESIAN_POINT ( 'NONE',  ( 19.90000000000000924, 4.611773100472912112, 22.11686199900910665 ) ) ;
#26552=AXIS2_PLACEMENT_3D ( 'NONE', #241543, #126731, #104566 ) ;
#26555=CARTESIAN_POINT ( 'NONE',  ( 20.90000000000000213, -1.786320531569725478, -11.50977166988710820 ) ) ;
#26559=PLANE ( 'NONE',  #191858 ) ;
#26640=VERTEX_POINT ( 'NONE', #77554 ) ;
#26671=EDGE_CURVE ( 'NONE', #10810, #176282, #180705, .T. ) ;
#26676=DIRECTION ( 'NONE',  ( 0.000000000000000000, 1.000000000000000000, 1.734723475976817507E-14 ) ) ;
#26721=EDGE_CURVE ( 'NONE', #32241, #161437, #224781, .T. ) ;
#26730=EDGE_CURVE ( 'NONE', #79286, #139556, #61880, .T. ) ;
#26731=DIRECTION ( 'NONE',  ( -1.000000000000000000, 0.000000000000000000, 0.000000000000000000 ) ) ;
#26747=VECTOR ( 'NONE', #82064, 1000.000000000000114 ) ;
#26765=VERTEX_POINT ( 'NONE', #3161 ) ;
#26777=AXIS2_PLACEMENT_3D ( 'NONE', #235534, #56873, #36079 ) ;
#26813=EDGE_CURVE ( 'NONE', #16688, #78593, #8338, .T. ) ;
#26923=DIRECTION ( 'NONE',  ( 0.000000000000000000, 0.9910465087640866200, -0.1335171055202867274 ) ) ;
#26937=EDGE_CURVE ( 'NONE', #216189, #66123, #164327, .T. ) ;
#26953=DIRECTION ( 'NONE',  ( -0.000000000000000000, 0.4856429311786307212, 0.8741572761215384846 ) ) ;
#26973=CARTESIAN_POINT ( 'NONE',  ( 21.00000000000000000, -1.410778198689825347, -7.973296578895943121 ) ) ;
#26976=CARTESIAN_POINT ( 'NONE',  ( -0.8999999999999993561, -11.65000000000000036, 23.30000000000000426 ) ) ;
#26984=CYLINDRICAL_SURFACE ( 'NONE', #252070, 0.09999999999999990841 ) ;
#27037=LINE ( 'NONE', #144349, #245562 ) ;
#27042=DIRECTION ( 'NONE',  ( -0.000000000000000000, 0.1686199900910463068, -0.9856811345164802063 ) ) ;
#27048=AXIS2_PLACEMENT_3D ( 'NONE', #253847, #94784, #53090 ) ;
#27071=DIRECTION ( 'NONE',  ( 1.000000000000000000, 0.000000000000000000, 0.000000000000000000 ) ) ;
#27127=CIRCLE ( 'NONE', #193697, 0.09999999999999939493 ) ;
#27130=AXIS2_PLACEMENT_3D ( 'NONE', #143875, #81309, #164741 ) ;
#27160=VECTOR ( 'NONE', #231104, 1000.000000000000114 ) ;
#27190=DIRECTION ( 'NONE',  ( -1.000000000000000000, 0.000000000000000000, -0.000000000000000000 ) ) ;
#27212=CARTESIAN_POINT ( 'NONE',  ( 18.59999999999999787, -11.65000000000000036, 6.000000000000001776 ) ) ;
#27218=DIRECTION ( 'NONE',  ( 1.000000000000000000, 0.000000000000000000, 0.000000000000000000 ) ) ;
#27290=DIRECTION ( 'NONE',  ( -1.000000000000000000, -1.476360405086644309E-16, 0.000000000000000000 ) ) ;
#27313=ORIENTED_EDGE ( 'NONE', *, *, #177474, .T. ) ;
#27327=FACE_OUTER_BOUND ( 'NONE', #50114, .T. ) ;
#27335=EDGE_LOOP ( 'NONE', ( #155686, #2683, #208275, #26451 ) ) ;
#27362=DIRECTION ( 'NONE',  ( 0.000000000000000000, 0.000000000000000000, 1.000000000000000000 ) ) ;
#27371=VERTEX_POINT ( 'NONE', #153993 ) ;
#27386=DIRECTION ( 'NONE',  ( 0.000000000000000000, -0.9910465087640866200, -0.1335171055202867274 ) ) ;
#27440=DIRECTION ( 'NONE',  ( -1.000000000000000000, -0.000000000000000000, -0.000000000000000000 ) ) ;
#27466=CIRCLE ( 'NONE', #10857, 0.09999999999999939493 ) ;
#27495=DIRECTION ( 'NONE',  ( 0.000000000000000000, -1.000000000000000000, 0.000000000000000000 ) ) ;
#27520=DIRECTION ( 'NONE',  ( -1.000000000000000000, 0.000000000000000000, 0.000000000000000000 ) ) ;
#27540=CYLINDRICAL_SURFACE ( 'NONE', #194477, 0.09999999999999939493 ) ;
#27570=CARTESIAN_POINT ( 'NONE',  ( -37.88850191057539973, -10.74999999999999289, -15.00000000000000000 ) ) ;
#27572=ORIENTED_EDGE ( 'NONE', *, *, #24924, .F. ) ;
#27605=CARTESIAN_POINT ( 'NONE',  ( 22.10000000000000497, 6.223900101154157483, 12.09999999999999964 ) ) ;
#27616=CARTESIAN_POINT ( 'NONE',  ( -18.79999999999999716, -8.250000000000005329, -7.800000000000000711 ) ) ;
#27663=DIRECTION ( 'NONE',  ( 0.000000000000000000, 0.000000000000000000, -1.000000000000000000 ) ) ;
#27679=CARTESIAN_POINT ( 'NONE',  ( -5.900000000000003020, -11.75000000000000000, 9.900000000000002132 ) ) ;
#27684=DIRECTION ( 'NONE',  ( -1.000000000000000000, -0.000000000000000000, -0.000000000000000000 ) ) ;
#27687=CARTESIAN_POINT ( 'NONE',  ( 18.79999999999999716, -1.410778198689825347, -7.973296578895943121 ) ) ;
#27707=CARTESIAN_POINT ( 'NONE',  ( 22.10000000000000497, 6.223900101154156594, 12.09999999999999964 ) ) ;
#27716=ORIENTED_EDGE ( 'NONE', *, *, #230025, .F. ) ;
#27767=CIRCLE ( 'NONE', #131783, 0.09999999999999939493 ) ;
#27792=ORIENTED_EDGE ( 'NONE', *, *, #138511, .F. ) ;
#27813=CIRCLE ( 'NONE', #240176, 4.900000000000004796 ) ;
#27830=CARTESIAN_POINT ( 'NONE',  ( 18.79999999999999716, 4.611773100472912112, 22.11686199900910665 ) ) ;
#27839=ORIENTED_EDGE ( 'NONE', *, *, #234520, .F. ) ;
#27860=DIRECTION ( 'NONE',  ( -0.000000000000000000, 0.000000000000000000, 1.000000000000000000 ) ) ;
#27867=DIRECTION ( 'NONE',  ( 0.000000000000000000, -1.000000000000000000, 0.000000000000000000 ) ) ;
#27929=CARTESIAN_POINT ( 'NONE',  ( -18.79999999999999716, -11.65000000000000036, 5.900000000000001243 ) ) ;
#27940=VERTEX_POINT ( 'NONE', #167459 ) ;
#27953=DIRECTION ( 'NONE',  ( 0.000000000000000000, 0.000000000000000000, 1.000000000000000000 ) ) ;
#28092=ORIENTED_EDGE ( 'NONE', *, *, #31759, .F. ) ;
#28103=EDGE_LOOP ( 'NONE', ( #188056, #115608, #156701, #63572 ) ) ;
#28105=ORIENTED_EDGE ( 'NONE', *, *, #190891, .T. ) ;
#28154=DIRECTION ( 'NONE',  ( 1.000000000000000000, 0.000000000000000000, 0.000000000000000000 ) ) ;
#28188=VERTEX_POINT ( 'NONE', #143699 ) ;
#28197=ORIENTED_EDGE ( 'NONE', *, *, #248824, .T. ) ;
#28220=CYLINDRICAL_SURFACE ( 'NONE', #49057, 0.09999999999999990841 ) ;
#28284=DIRECTION ( 'NONE',  ( 0.000000000000000000, 1.000000000000000000, 0.000000000000000000 ) ) ;
#28286=DIRECTION ( 'NONE',  ( 0.000000000000000000, 0.9856811345164803173, 0.1686199900910455851 ) ) ;
#28302=AXIS2_PLACEMENT_3D ( 'NONE', #228485, #188064, #49827 ) ;
#28361=ORIENTED_EDGE ( 'NONE', *, *, #179370, .F. ) ;
#28413=ORIENTED_EDGE ( 'NONE', *, *, #256561, .T. ) ;
#28416=DIRECTION ( 'NONE',  ( 0.000000000000000000, 0.000000000000000000, -1.000000000000000000 ) ) ;
#28424=ORIENTED_EDGE ( 'NONE', *, *, #63427, .T. ) ;
#28472=EDGE_LOOP ( 'NONE', ( #243184, #223803, #139535 ) ) ;
#28521=DIRECTION ( 'NONE',  ( 0.000000000000000000, 0.1335171055202867274, -0.9910465087640866200 ) ) ;
#28533=CARTESIAN_POINT ( 'NONE',  ( -18.79999999999999716, 1.800000000000000044, -11.61130914238355771 ) ) ;
#28591=DIRECTION ( 'NONE',  ( 1.000000000000000000, 0.000000000000000000, 0.000000000000000000 ) ) ;
#28603=TOROIDAL_SURFACE ( 'NONE', #207627, 4.100000000000000533, 0.1000000000000000056 ) ;
#28631=ORIENTED_EDGE ( 'NONE', *, *, #214398, .T. ) ;
#28672=AXIS2_PLACEMENT_3D ( 'NONE', #43797, #244548, #106306 ) ;
#28685=LINE ( 'NONE', #113303, #231133 ) ;
#28763=VERTEX_POINT ( 'NONE', #37264 ) ;
#28768=VECTOR ( 'NONE', #172786, 1000.000000000000227 ) ;
#28789=EDGE_CURVE ( 'NONE', #92927, #57247, #65268, .T. ) ;
#28791=ORIENTED_EDGE ( 'NONE', *, *, #151485, .F. ) ;
#28792=ORIENTED_EDGE ( 'NONE', *, *, #256894, .T. ) ;
#28823=CARTESIAN_POINT ( 'NONE',  ( -18.79999999999999716, 8.000000000000000000, -1.212568896937008089 ) ) ;
#28850=CARTESIAN_POINT ( 'NONE',  ( 22.10000000000000142, -3.262756495241484158E-15, 32.89999999999999858 ) ) ;
#28873=TOROIDAL_SURFACE ( 'NONE', #145331, 11.65000000000000036, 0.1000000000000000056 ) ;
#28901=CARTESIAN_POINT ( 'NONE',  ( 18.59999999999999787, -10.64999999999999325, 31.59999999999999787 ) ) ;
#28916=FACE_OUTER_BOUND ( 'NONE', #213179, .T. ) ;
#28930=CARTESIAN_POINT ( 'NONE',  ( -18.79999999999999716, 1.885425182446133885, -11.49641995933507843 ) ) ;
#28935=DIRECTION ( 'NONE',  ( 0.000000000000000000, 0.1335171055202821200, -0.9910465087640870641 ) ) ;
#28969=LINE ( 'NONE', #143719, #106160 ) ;
#28971=CYLINDRICAL_SURFACE ( 'NONE', #111337, 0.1000000000000000472 ) ;
#28993=ORIENTED_EDGE ( 'NONE', *, *, #49354, .T. ) ;
#29029=CARTESIAN_POINT ( 'NONE',  ( -18.69999999999999929, 1.350000000000000089, 16.60000000000000142 ) ) ;
#29048=EDGE_CURVE ( 'NONE', #105944, #213256, #244320, .T. ) ;
#29079=CIRCLE ( 'NONE', #149867, 0.1000000000000002554 ) ;
#29111=VERTEX_POINT ( 'NONE', #155646 ) ;
#29170=PLANE ( 'NONE',  #253563 ) ;
#29178=EDGE_CURVE ( 'NONE', #55862, #102889, #202818, .T. ) ;
#29236=DIRECTION ( 'NONE',  ( 0.000000000000000000, 0.000000000000000000, 1.000000000000000000 ) ) ;
#29259=AXIS2_PLACEMENT_3D ( 'NONE', #12148, #27867, #186935 ) ;
#29273=AXIS2_PLACEMENT_3D ( 'NONE', #163162, #228268, #232125 ) ;
#29303=EDGE_LOOP ( 'NONE', ( #174258, #138070, #138580, #55651 ) ) ;
#29328=FACE_OUTER_BOUND ( 'NONE', #130502, .T. ) ;
#29339=CYLINDRICAL_SURFACE ( 'NONE', #72201, 0.1000000000000000472 ) ;
#29341=ORIENTED_EDGE ( 'NONE', *, *, #237310, .F. ) ;
#29365=DIRECTION ( 'NONE',  ( 0.000000000000000000, 0.000000000000000000, -1.000000000000000000 ) ) ;
#29398=EDGE_CURVE ( 'NONE', #235390, #158566, #108472, .T. ) ;
#29407=CARTESIAN_POINT ( 'NONE',  ( -22.19999999999999929, -11.75000000000000000, -15.00000000000000000 ) ) ;
#29419=CARTESIAN_POINT ( 'NONE',  ( -22.94999999999999929, 7.900000000000000355, -1.300000000000000044 ) ) ;
#29448=DIRECTION ( 'NONE',  ( 1.000000000000000000, -0.000000000000000000, -0.000000000000000000 ) ) ;
#29470=EDGE_LOOP ( 'NONE', ( #160152, #221436, #160524, #98651 ) ) ;
#29476=AXIS2_PLACEMENT_3D ( 'NONE', #137040, #221687, #196994 ) ;
#29481=CYLINDRICAL_SURFACE ( 'NONE', #215822, 0.1000000000000002554 ) ;
#29521=EDGE_LOOP ( 'NONE', ( #165931, #72918, #122384, #209941 ) ) ;
#29524=LINE ( 'NONE', #68624, #103430 ) ;
#29530=CARTESIAN_POINT ( 'NONE',  ( -18.79999999999999716, 0.000000000000000000, 0.000000000000000000 ) ) ;
#29531=VECTOR ( 'NONE', #245709, 1000.000000000000000 ) ;
#29618=CIRCLE ( 'NONE', #204552, 0.09999999999999939493 ) ;
#29621=VERTEX_POINT ( 'NONE', #96583 ) ;
#29657=CARTESIAN_POINT ( 'NONE',  ( 20.00000000000000355, 5.454087299794355914, 16.60000000000000142 ) ) ;
#29670=CARTESIAN_POINT ( 'NONE',  ( 22.10000000000000497, -11.75000000000000000, 32.89999999999999858 ) ) ;
#29676=VECTOR ( 'NONE', #6301, 1000.000000000000000 ) ;
#29702=CARTESIAN_POINT ( 'NONE',  ( -19.89999999999999858, 4.611773100472912112, 22.11686199900910665 ) ) ;
#29742=ORIENTED_EDGE ( 'NONE', *, *, #15944, .T. ) ;
#29751=CYLINDRICAL_SURFACE ( 'NONE', #224, 0.09999999999999939493 ) ;
#29773=CARTESIAN_POINT ( 'NONE',  ( -18.79999999999999716, 3.461118860469513336, 28.84309995045515507 ) ) ;
#29814=AXIS2_PLACEMENT_3D ( 'NONE', #219036, #142067, #61261 ) ;
#29849=FACE_OUTER_BOUND ( 'NONE', #12497, .T. ) ;
#29889=DIRECTION ( 'NONE',  ( 0.000000000000000000, 0.000000000000000000, -1.000000000000000000 ) ) ;
#29910=FACE_OUTER_BOUND ( 'NONE', #82322, .T. ) ;
#29961=DIRECTION ( 'NONE',  ( 1.000000000000000000, 0.000000000000000000, -0.000000000000000000 ) ) ;
#29964=EDGE_LOOP ( 'NONE', ( #122229, #11959, #86804, #141231 ) ) ;
#29971=EDGE_CURVE ( 'NONE', #245573, #69468, #135411, .T. ) ;
#30045=CARTESIAN_POINT ( 'NONE',  ( 22.94999999999999929, 0.000000000000000000, 0.000000000000000000 ) ) ;
#30062=ORIENTED_EDGE ( 'NONE', *, *, #70594, .T. ) ;
#30076=VERTEX_POINT ( 'NONE', #119730 ) ;
#30081=CARTESIAN_POINT ( 'NONE',  ( 20.89999999999999503, 1.212568896937007645, -8.000000000000000000 ) ) ;
#30085=DIRECTION ( 'NONE',  ( 0.000000000000000000, 0.000000000000000000, 1.000000000000000000 ) ) ;
#30104=DIRECTION ( 'NONE',  ( 1.000000000000000000, 0.000000000000000000, 0.000000000000000000 ) ) ;
#30142=AXIS2_PLACEMENT_3D ( 'NONE', #74988, #97041, #137478 ) ;
#30154=ADVANCED_FACE ( 'NONE', ( #144377 ), #25749, .F. ) ;
#30178=CYLINDRICAL_SURFACE ( 'NONE', #226827, 0.09999999999999939493 ) ;
#30215=VECTOR ( 'NONE', #179963, 1000.000000000000000 ) ;
#30239=ADVANCED_FACE ( 'NONE', ( #132555 ), #135179, .T. ) ;
#30257=DIRECTION ( 'NONE',  ( -1.000000000000000000, 0.000000000000000000, 0.000000000000000000 ) ) ;
#30292=VECTOR ( 'NONE', #78080, 1000.000000000000000 ) ;
#30340=ADVANCED_FACE ( 'NONE', ( #222316 ), #43715, .T. ) ;
#30362=CYLINDRICAL_SURFACE ( 'NONE', #88679, 0.1000000000000000472 ) ;
#30411=ORIENTED_EDGE ( 'NONE', *, *, #71398, .F. ) ;
#30420=DIRECTION ( 'NONE',  ( 0.000000000000000000, 0.000000000000000000, -1.000000000000000000 ) ) ;
#30424=VECTOR ( 'NONE', #221152, 1000.000000000000000 ) ;
#30425=CARTESIAN_POINT ( 'NONE',  ( 18.79999999999999716, 11.75000000000000000, 22.10000000000000142 ) ) ;
#30429=CIRCLE ( 'NONE', #255212, 4.900000000000004796 ) ;
#30451=CARTESIAN_POINT ( 'NONE',  ( -18.79999999999999716, 6.783826713665066066, 9.593862367105556288 ) ) ;
#30457=DIRECTION ( 'NONE',  ( 1.000000000000000000, -0.000000000000000000, 0.000000000000000000 ) ) ;
#30459=ORIENTED_EDGE ( 'NONE', *, *, #256556, .T. ) ;
#30482=AXIS2_PLACEMENT_3D ( 'NONE', #3014, #141266, #82537 ) ;
#30523=ORIENTED_EDGE ( 'NONE', *, *, #252746, .F. ) ;
#30603=CARTESIAN_POINT ( 'NONE',  ( 21.10000000000000142, 5.021051876504148371E-16, 4.100000000000000533 ) ) ;
#30719=CARTESIAN_POINT ( 'NONE',  ( 22.19999999999999929, -11.65000000000000036, 32.89999999999999858 ) ) ;
#30726=DIRECTION ( 'NONE',  ( 1.000000000000000000, 0.000000000000000000, 0.000000000000000000 ) ) ;
#30747=CARTESIAN_POINT ( 'NONE',  ( 20.90000000000000213, 11.50977166988710820, -1.786320531569725478 ) ) ;
#30757=FACE_OUTER_BOUND ( 'NONE', #45458, .T. ) ;
#30776=AXIS2_PLACEMENT_3D ( 'NONE', #163598, #144011, #220979 ) ;
#30794=EDGE_LOOP ( 'NONE', ( #130918, #202320, #243620, #249465 ) ) ;
#30795=DIRECTION ( 'NONE',  ( 1.000000000000000000, 0.000000000000000000, 0.000000000000000000 ) ) ;
#30830=AXIS2_PLACEMENT_3D ( 'NONE', #245043, #70290, #48119 ) ;
#30843=CIRCLE ( 'NONE', #189045, 0.09999999999999939493 ) ;
#30847=DIRECTION ( 'NONE',  ( -1.000000000000000000, 0.000000000000000000, 0.000000000000000000 ) ) ;
#30861=ORIENTED_EDGE ( 'NONE', *, *, #239238, .T. ) ;
#30865=ADVANCED_FACE ( 'NONE', ( #97454 ), #58332, .T. ) ;
#30944=EDGE_CURVE ( 'NONE', #207912, #5669, #89758, .T. ) ;
#30948=CIRCLE ( 'NONE', #64231, 0.09999999999999939493 ) ;
#30959=CARTESIAN_POINT ( 'NONE',  ( -20.90000000000000213, 6.841561409100513025, 9.675512259591560138 ) ) ;
#31068=DIRECTION ( 'NONE',  ( 0.000000000000000000, -0.9910465087640865089, 0.1335171055202867274 ) ) ;
#31075=CYLINDRICAL_SURFACE ( 'NONE', #125139, 0.09999999999999939493 ) ;
#31089=DIRECTION ( 'NONE',  ( 0.000000000000000000, 0.9856811345164800953, 0.1686199900910462790 ) ) ;
#31105=CARTESIAN_POINT ( 'NONE',  ( -21.10000000000000497, 6.342459739679071618, 12.00000000000000355 ) ) ;
#31132=DIRECTION ( 'NONE',  ( 0.000000000000000000, 0.000000000000000000, 1.000000000000000000 ) ) ;
#31171=ADVANCED_FACE ( 'NONE', ( #26292 ), #189216, .F. ) ;
#31178=ADVANCED_FACE ( 'NONE', ( #167113 ), #148809, .T. ) ;
#31202=ORIENTED_EDGE ( 'NONE', *, *, #236248, .T. ) ;
#31232=FACE_OUTER_BOUND ( 'NONE', #162114, .T. ) ;
#31237=AXIS2_PLACEMENT_3D ( 'NONE', #183985, #144847, #88713 ) ;
#31242=CARTESIAN_POINT ( 'NONE',  ( 13.40000000000000036, -8.250000000000005329, 19.04142135623731136 ) ) ;
#31255=TOROIDAL_SURFACE ( 'NONE', #72939, 0.2000000000000000111, 0.1000000000000000056 ) ;
#31285=ORIENTED_EDGE ( 'NONE', *, *, #84250, .T. ) ;
#31335=DIRECTION ( 'NONE',  ( -0.000000000000000000, 1.000000000000000000, -0.000000000000000000 ) ) ;
#31339=DIRECTION ( 'NONE',  ( 0.000000000000000000, 0.000000000000000000, -1.000000000000000000 ) ) ;
#31355=FACE_OUTER_BOUND ( 'NONE', #57405, .T. ) ;
#31364=CARTESIAN_POINT ( 'NONE',  ( 18.79999999999999361, -11.65000000000000036, 32.89999999999999858 ) ) ;
#31466=CARTESIAN_POINT ( 'NONE',  ( 21.00000000000000000, 6.239477252822119624, 11.95447128030241224 ) ) ;
#31483=ORIENTED_EDGE ( 'NONE', *, *, #2486, .T. ) ;
#31600=ORIENTED_EDGE ( 'NONE', *, *, #13639, .F. ) ;
#31617=VERTEX_POINT ( 'NONE', #132797 ) ;
#31635=LINE ( 'NONE', #250634, #170052 ) ;
#31711=DIRECTION ( 'NONE',  ( 1.000000000000000000, 0.000000000000000000, 0.000000000000000000 ) ) ;
#31730=EDGE_CURVE ( 'NONE', #184818, #159030, #164418, .T. ) ;
#31759=EDGE_CURVE ( 'NONE', #75451, #52766, #98736, .T. ) ;
#31762=ORIENTED_EDGE ( 'NONE', *, *, #37549, .T. ) ;
#31828=CARTESIAN_POINT ( 'NONE',  ( -22.10000000000000142, -11.65000000000000036, 32.89999999999999858 ) ) ;
#31853=EDGE_CURVE ( 'NONE', #200951, #121041, #107445, .T. ) ;
#31900=EDGE_LOOP ( 'NONE', ( #41490, #179690, #102546, #199935 ) ) ;
#31909=DIRECTION ( 'NONE',  ( 0.000000000000000000, -0.1686199900910528293, 0.9856811345164792071 ) ) ;
#31962=PLANE ( 'NONE',  #120947 ) ;
#32025=ORIENTED_EDGE ( 'NONE', *, *, #22619, .T. ) ;
#32034=CIRCLE ( 'NONE', #215168, 0.09999999999999939493 ) ;
#32125=FACE_OUTER_BOUND ( 'NONE', #14503, .T. ) ;
#32130=VECTOR ( 'NONE', #16677, 1000.000000000000000 ) ;
#32142=DIRECTION ( 'NONE',  ( -0.000000000000000000, 1.000000000000000000, -0.000000000000000000 ) ) ;
#32178=DIRECTION ( 'NONE',  ( 1.000000000000000000, 0.000000000000000000, 0.000000000000000000 ) ) ;
#32182=ORIENTED_EDGE ( 'NONE', *, *, #211764, .T. ) ;
#32233=DIRECTION ( 'NONE',  ( -1.000000000000000000, 0.000000000000000000, -0.000000000000000000 ) ) ;
#32237=FACE_OUTER_BOUND ( 'NONE', #23270, .T. ) ;
#32241=VERTEX_POINT ( 'NONE', #247927 ) ;
#32268=ADVANCED_FACE ( 'NONE', ( #126708 ), #11921, .F. ) ;
#32283=ORIENTED_EDGE ( 'NONE', *, *, #33837, .F. ) ;
#32298=FACE_OUTER_BOUND ( 'NONE', #96395, .T. ) ;
#32309=ORIENTED_EDGE ( 'NONE', *, *, #14663, .F. ) ;
#32327=ORIENTED_EDGE ( 'NONE', *, *, #6400, .T. ) ;
#32335=EDGE_CURVE ( 'NONE', #227995, #149638, #73228, .T. ) ;
#32342=DIRECTION ( 'NONE',  ( 0.000000000000000000, 0.000000000000000000, -1.000000000000000000 ) ) ;
#32349=CARTESIAN_POINT ( 'NONE',  ( -18.59999999999999787, -10.64999999999999325, 33.00000000000000000 ) ) ;
#32356=CARTESIAN_POINT ( 'NONE',  ( -21.00000000000000000, -1.720267447010333833E-15, 11.89999999999999858 ) ) ;
#32400=ORIENTED_EDGE ( 'NONE', *, *, #86158, .T. ) ;
#32407=LINE ( 'NONE', #230585, #20492 ) ;
#32523=ORIENTED_EDGE ( 'NONE', *, *, #190891, .F. ) ;
#32531=FACE_OUTER_BOUND ( 'NONE', #29470, .T. ) ;
#32571=DIRECTION ( 'NONE',  ( 0.000000000000000000, 0.000000000000000000, 1.000000000000000000 ) ) ;
#32581=FACE_OUTER_BOUND ( 'NONE', #257660, .T. ) ;
#32635=CIRCLE ( 'NONE', #153630, 0.09999999999999939493 ) ;
#32661=ORIENTED_EDGE ( 'NONE', *, *, #215935, .F. ) ;
#32667=DIRECTION ( 'NONE',  ( 0.000000000000000000, 0.1618390714546045217, 0.9868171638914230437 ) ) ;
#32703=CARTESIAN_POINT ( 'NONE',  ( 18.59999999999999787, -10.80884033489985363, 5.900000000000001243 ) ) ;
#32725=DIRECTION ( 'NONE',  ( 0.000000000000000000, 1.000000000000000000, 0.000000000000000000 ) ) ;
#32753=AXIS2_PLACEMENT_3D ( 'NONE', #205735, #67512, #45386 ) ;
#32775=ORIENTED_EDGE ( 'NONE', *, *, #108959, .F. ) ;
#32802=AXIS2_PLACEMENT_3D ( 'NONE', #44788, #124328, #142579 ) ;
#32816=ORIENTED_EDGE ( 'NONE', *, *, #59149, .T. ) ;
#32884=CARTESIAN_POINT ( 'NONE',  ( -22.94999999999999929, 5.488301202077012775, 16.40000000000000213 ) ) ;
#32888=EDGE_CURVE ( 'NONE', #110926, #257982, #162656, .T. ) ;
#32901=ORIENTED_EDGE ( 'NONE', *, *, #239815, .F. ) ;
#32908=ORIENTED_EDGE ( 'NONE', *, *, #234361, .F. ) ;
#32935=ADVANCED_FACE ( 'NONE', ( #119681 ), #231594, .T. ) ;
#32951=LINE ( 'NONE', #156742, #126407 ) ;
#32983=AXIS2_PLACEMENT_3D ( 'NONE', #108966, #188512, #89403 ) ;
#32988=ORIENTED_EDGE ( 'NONE', *, *, #55320, .F. ) ;
#33047=CIRCLE ( 'NONE', #212072, 0.09999999999999939493 ) ;
#33074=CARTESIAN_POINT ( 'NONE',  ( 20.00000000000000355, 1.249999999999999334, 16.60000000000000142 ) ) ;
#33096=CARTESIAN_POINT ( 'NONE',  ( 18.79999999999999716, 11.61130914238355771, 22.00000000000000355 ) ) ;
#33111=FACE_OUTER_BOUND ( 'NONE', #133507, .T. ) ;
#33123=ORIENTED_EDGE ( 'NONE', *, *, #208992, .F. ) ;
#33156=ORIENTED_EDGE ( 'NONE', *, *, #233549, .T. ) ;
#33178=CIRCLE ( 'NONE', #249625, 11.75000000000000000 ) ;
#33189=DIRECTION ( 'NONE',  ( -1.000000000000000000, -0.000000000000000000, -0.000000000000000000 ) ) ;
#33256=DIRECTION ( 'NONE',  ( -0.000000000000000000, 0.1335171055202901413, -0.9910465087640860649 ) ) ;
#33302=CARTESIAN_POINT ( 'NONE',  ( -18.69999999999999929, 1.410778198689828900, -7.973296578895943121 ) ) ;
#33369=AXIS2_PLACEMENT_3D ( 'NONE', #76191, #197427, #215695 ) ;
#33376=VERTEX_POINT ( 'NONE', #85336 ) ;
#33400=ORIENTED_EDGE ( 'NONE', *, *, #205370, .F. ) ;
#33461=EDGE_LOOP ( 'NONE', ( #110578, #123195, #14201 ) ) ;
#33531=EDGE_CURVE ( 'NONE', #49507, #240745, #119551, .T. ) ;
#33596=ORIENTED_EDGE ( 'NONE', *, *, #118921, .F. ) ;
#33599=AXIS2_PLACEMENT_3D ( 'NONE', #101508, #144507, #124974 ) ;
#33682=CARTESIAN_POINT ( 'NONE',  ( 20.00000000000000355, 1.250000000000000000, 21.90000000000000213 ) ) ;
#33703=CARTESIAN_POINT ( 'NONE',  ( 18.59999999999999787, -10.74999999999999289, 33.00000000000000000 ) ) ;
#33777=LINE ( 'NONE', #62275, #226534 ) ;
#33781=DIRECTION ( 'NONE',  ( 0.000000000000000000, -1.734723475976817507E-14, 1.000000000000000000 ) ) ;
#33829=ADVANCED_FACE ( 'NONE', ( #48180 ), #106863, .T. ) ;
#33837=EDGE_CURVE ( 'NONE', #233025, #237894, #128094, .T. ) ;
#33843=DIRECTION ( 'NONE',  ( -0.000000000000000000, 1.000000000000000000, -0.000000000000000000 ) ) ;
#33864=EDGE_LOOP ( 'NONE', ( #6150, #126818, #164840, #152487 ) ) ;
#33872=TOROIDAL_SURFACE ( 'NONE', #150539, 4.900000000000003020, 0.1000000000000000056 ) ;
#33911=DIRECTION ( 'NONE',  ( -1.000000000000000000, 0.000000000000000000, 0.000000000000000000 ) ) ;
#33923=DIRECTION ( 'NONE',  ( 1.000000000000000000, -0.000000000000000000, -0.000000000000000000 ) ) ;
#33955=DIRECTION ( 'NONE',  ( 0.000000000000000000, -1.000000000000000000, 0.000000000000000000 ) ) ;
#33983=ORIENTED_EDGE ( 'NONE', *, *, #63256, .F. ) ;
#33990=EDGE_LOOP ( 'NONE', ( #46067, #14337, #73615, #87738 ) ) ;
#34006=VECTOR ( 'NONE', #187275, 1000.000000000000114 ) ;
#34090=AXIS2_PLACEMENT_3D ( 'NONE', #241200, #99073, #116112 ) ;
#34112=ADVANCED_FACE ( 'NONE', ( #101374 ), #180976, .T. ) ;
#34117=CARTESIAN_POINT ( 'NONE',  ( -20.90000000000000213, 11.49641995933507843, -1.885425182446133885 ) ) ;
#34197=LINE ( 'NONE', #14623, #68657 ) ;
#34213=CARTESIAN_POINT ( 'NONE',  ( -18.59999999999999787, -11.75000000000000000, 6.100000000000001421 ) ) ;
#34218=ORIENTED_EDGE ( 'NONE', *, *, #188246, .F. ) ;
#34222=AXIS2_PLACEMENT_3D ( 'NONE', #165588, #160468, #142150 ) ;
#34242=DIRECTION ( 'NONE',  ( 1.000000000000000000, -0.000000000000000000, -0.000000000000000000 ) ) ;
#34248=EDGE_CURVE ( 'NONE', #109505, #126, #128706, .T. ) ;
#34269=AXIS2_PLACEMENT_3D ( 'NONE', #197836, #113177, #192721 ) ;
#34286=VERTEX_POINT ( 'NONE', #77678 ) ;
#34307=ORIENTED_EDGE ( 'NONE', *, *, #34948, .F. ) ;
#34417=CARTESIAN_POINT ( 'NONE',  ( 20.90000000000000213, -1.800000000000000044, -11.61130914238355771 ) ) ;
#34433=EDGE_LOOP ( 'NONE', ( #15143, #221995, #103743, #178720 ) ) ;
#34445=ORIENTED_EDGE ( 'NONE', *, *, #235983, .F. ) ;
#34451=TOROIDAL_SURFACE ( 'NONE', #9467, 0.2000000000000000111, 0.1000000000000000056 ) ;
#34453=AXIS2_PLACEMENT_3D ( 'NONE', #7730, #218086, #87235 ) ;
#34497=CARTESIAN_POINT ( 'NONE',  ( 21.00000000000000000, -0.04453801223857078301, -0.3305886640091971196 ) ) ;
#34547=EDGE_CURVE ( 'NONE', #93865, #41107, #154293, .T. ) ;
#34569=CYLINDRICAL_SURFACE ( 'NONE', #30142, 0.09999999999999939493 ) ;
#34600=AXIS2_PLACEMENT_3D ( 'NONE', #131604, #33843, #53355 ) ;
#34613=LINE ( 'NONE', #55398, #67457 ) ;
#34620=CARTESIAN_POINT ( 'NONE',  ( 20.00000000000000355, 1.350000000000000089, 21.90000000000000213 ) ) ;
#34649=FACE_OUTER_BOUND ( 'NONE', #73185, .T. ) ;
#34657=EDGE_LOOP ( 'NONE', ( #243766, #79910, #70178, #76798 ) ) ;
#34687=CARTESIAN_POINT ( 'NONE',  ( 18.69999999999999929, 1.149999999999999911, 16.60000000000000142 ) ) ;
#34719=CARTESIAN_POINT ( 'NONE',  ( 18.79999999999999716, 1.885425182446133885, -11.49641995933507843 ) ) ;
#34721=ORIENTED_EDGE ( 'NONE', *, *, #171769, .T. ) ;
#34773=DIRECTION ( 'NONE',  ( -1.000000000000000000, 0.000000000000000000, 0.000000000000000000 ) ) ;
#34783=ORIENTED_EDGE ( 'NONE', *, *, #45630, .F. ) ;
#34807=FACE_OUTER_BOUND ( 'NONE', #136749, .T. ) ;
#34816=ORIENTED_EDGE ( 'NONE', *, *, #43261, .T. ) ;
#34819=ORIENTED_EDGE ( 'NONE', *, *, #123186, .F. ) ;
#34843=ORIENTED_EDGE ( 'NONE', *, *, #122979, .T. ) ;
#34850=VERTEX_POINT ( 'NONE', #68470 ) ;
#34931=EDGE_CURVE ( 'NONE', #89225, #248318, #257310, .T. ) ;
#34945=CIRCLE ( 'NONE', #234816, 0.1000000000000002554 ) ;
#34947=LINE ( 'NONE', #54464, #78275 ) ;
#34948=EDGE_CURVE ( 'NONE', #132961, #93865, #22076, .T. ) ;
#34953=CARTESIAN_POINT ( 'NONE',  ( 20.00000000000000355, 1.350000000000000089, 22.00000000000000355 ) ) ;
#35001=DIRECTION ( 'NONE',  ( -1.000000000000000000, -0.000000000000000000, -0.000000000000000000 ) ) ;
#35036=VECTOR ( 'NONE', #232249, 1000.000000000000000 ) ;
#35091=ORIENTED_EDGE ( 'NONE', *, *, #134603, .T. ) ;
#35148=VECTOR ( 'NONE', #76505, 1000.000000000000000 ) ;
#35153=ORIENTED_EDGE ( 'NONE', *, *, #50655, .F. ) ;
#35210=ORIENTED_EDGE ( 'NONE', *, *, #21477, .T. ) ;
#35231=ADVANCED_FACE ( 'NONE', ( #246783 ), #107277, .F. ) ;
#35295=DIRECTION ( 'NONE',  ( 1.000000000000000000, 0.000000000000000000, 0.000000000000000000 ) ) ;
#35327=CIRCLE ( 'NONE', #81234, 4.000000000000000000 ) ;
#35370=DIRECTION ( 'NONE',  ( 1.000000000000000000, -0.000000000000000000, -0.000000000000000000 ) ) ;
#35399=DIRECTION ( 'NONE',  ( 1.000000000000000000, -0.000000000000000000, -0.000000000000000000 ) ) ;
#35401=TOROIDAL_SURFACE ( 'NONE', #160292, 0.2000000000000000111, 0.1000000000000000056 ) ;
#35405=ORIENTED_EDGE ( 'NONE', *, *, #168326, .T. ) ;
#35431=EDGE_CURVE ( 'NONE', #12989, #225036, #215365, .T. ) ;
#35432=ORIENTED_EDGE ( 'NONE', *, *, #90316, .F. ) ;
#35466=CARTESIAN_POINT ( 'NONE',  ( -5.900000000000003020, -11.34999999999999964, 10.00000000000000178 ) ) ;
#35536=DIRECTION ( 'NONE',  ( -1.000000000000000000, -0.000000000000000000, 0.000000000000000000 ) ) ;
#35549=CARTESIAN_POINT ( 'NONE',  ( 21.10000000000000142, 6.223900101154157483, 12.00000000000000000 ) ) ;
#35623=VECTOR ( 'NONE', #183555, 1000.000000000000000 ) ;
#35630=ORIENTED_EDGE ( 'NONE', *, *, #56128, .T. ) ;
#35649=AXIS2_PLACEMENT_3D ( 'NONE', #25593, #122124, #23042 ) ;
#35700=CARTESIAN_POINT ( 'NONE',  ( -22.94999999999999929, 1.901609089591594692, -11.59510167572422112 ) ) ;
#35778=DIRECTION ( 'NONE',  ( 0.000000000000000000, 0.8741572761215393728, -0.4856429311786291669 ) ) ;
#35787=AXIS2_PLACEMENT_3D ( 'NONE', #158839, #212388, #33781 ) ;
#35824=DIRECTION ( 'NONE',  ( 0.000000000000000000, 1.000000000000000000, 0.000000000000000000 ) ) ;
#35885=DIRECTION ( 'NONE',  ( -0.000000000000000000, 0.000000000000000000, 1.000000000000000000 ) ) ;
#35908=AXIS2_PLACEMENT_3D ( 'NONE', #91317, #32667, #48326 ) ;
#35910=CARTESIAN_POINT ( 'NONE',  ( 18.59999999999999787, 11.75000000000000000, 31.39999999999999858 ) ) ;
#35923=DIRECTION ( 'NONE',  ( 0.000000000000000000, -0.9910465087640866200, 0.1335171055202861445 ) ) ;
#35930=DIRECTION ( 'NONE',  ( 1.000000000000000000, 0.000000000000000000, 0.000000000000000000 ) ) ;
#35970=DIRECTION ( 'NONE',  ( 0.000000000000000000, 0.000000000000000000, -1.000000000000000000 ) ) ;
#35999=DIRECTION ( 'NONE',  ( 0.000000000000000000, 0.000000000000000000, 1.000000000000000000 ) ) ;
#36075=EDGE_CURVE ( 'NONE', #86236, #188417, #187188, .T. ) ;
#36079=DIRECTION ( 'NONE',  ( 0.000000000000000000, 0.9868171638914228216, 0.1618390714546044939 ) ) ;
#36081=EDGE_LOOP ( 'NONE', ( #19278, #159204, #166593, #232669, #159177, #53910, #60021, #79419, #31483, #49830, #220427, #43774, #78830, #44910, #152805, #32816, #79049, #34721, #162293, #231337, #84163, #35405, #37486, #100398, #56643, #39271, #22005, #142092, #213429 ) ) ;
#36085=ORIENTED_EDGE ( 'NONE', *, *, #137657, .T. ) ;
#36092=EDGE_CURVE ( 'NONE', #193487, #190676, #241445, .T. ) ;
#36095=LINE ( 'NONE', #17778, #36600 ) ;
#36202=DIRECTION ( 'NONE',  ( 0.000000000000000000, -0.1335171055202867274, -0.9910465087640865089 ) ) ;
#36224=EDGE_CURVE ( 'NONE', #171414, #92448, #133287, .T. ) ;
#36275=CIRCLE ( 'NONE', #57066, 11.65000000000000036 ) ;
#36295=AXIS2_PLACEMENT_3D ( 'NONE', #142559, #43481, #184263 ) ;
#36304=EDGE_CURVE ( 'NONE', #10010, #256387, #8392, .T. ) ;
#36308=ORIENTED_EDGE ( 'NONE', *, *, #86373, .F. ) ;
#36331=VERTEX_POINT ( 'NONE', #22680 ) ;
#36411=CYLINDRICAL_SURFACE ( 'NONE', #164325, 0.1000000000000002554 ) ;
#36416=ADVANCED_FACE ( 'NONE', ( #192025 ), #231155, .T. ) ;
#36419=DIRECTION ( 'NONE',  ( 0.000000000000000000, 0.000000000000000000, -1.000000000000000000 ) ) ;
#36445=AXIS2_PLACEMENT_3D ( 'NONE', #75320, #218632, #20471 ) ;
#36448=AXIS2_PLACEMENT_3D ( 'NONE', #203254, #5028, #28521 ) ;
#36450=LINE ( 'NONE', #156404, #26312 ) ;
#36527=EDGE_LOOP ( 'NONE', ( #78486, #246618, #255392, #47106 ) ) ;
#36532=ADVANCED_FACE ( 'NONE', ( #215413 ), #232875, .T. ) ;
#36546=EDGE_CURVE ( 'NONE', #207912, #45068, #16390, .T. ) ;
#36551=CYLINDRICAL_SURFACE ( 'NONE', #138743, 5.000000000000004441 ) ;
#36581=ORIENTED_EDGE ( 'NONE', *, *, #124514, .T. ) ;
#36600=VECTOR ( 'NONE', #178183, 1000.000000000000000 ) ;
#36612=DIRECTION ( 'NONE',  ( -0.000000000000000000, -0.000000000000000000, -1.000000000000000000 ) ) ;
#36630=ORIENTED_EDGE ( 'NONE', *, *, #153882, .F. ) ;
#36650=AXIS2_PLACEMENT_3D ( 'NONE', #153025, #216798, #117704 ) ;
#36678=CIRCLE ( 'NONE', #132503, 0.09999999999999963085 ) ;
#36708=EDGE_LOOP ( 'NONE', ( #48915, #113114, #84453, #129194 ) ) ;
#36739=ORIENTED_EDGE ( 'NONE', *, *, #118921, .T. ) ;
#36778=CARTESIAN_POINT ( 'NONE',  ( -21.10000000000000142, 11.99999999999999822, 12.00000000000000000 ) ) ;
#36795=ORIENTED_EDGE ( 'NONE', *, *, #256305, .F. ) ;
#36818=DIRECTION ( 'NONE',  ( 0.000000000000000000, 0.000000000000000000, 1.000000000000000000 ) ) ;
#36865=DIRECTION ( 'NONE',  ( 0.000000000000000000, 0.000000000000000000, -1.000000000000000000 ) ) ;
#36876=FACE_OUTER_BOUND ( 'NONE', #257694, .T. ) ;
#36888=VERTEX_POINT ( 'NONE', #167038 ) ;
#36892=DIRECTION ( 'NONE',  ( 0.000000000000000000, 0.000000000000000000, -1.000000000000000000 ) ) ;
#36901=DIRECTION ( 'NONE',  ( 0.000000000000000000, -1.000000000000000000, 0.000000000000000000 ) ) ;
#36948=VECTOR ( 'NONE', #89777, 1000.000000000000000 ) ;
#36959=ADVANCED_FACE ( 'NONE', ( #133023 ), #256752, .F. ) ;
#36971=EDGE_LOOP ( 'NONE', ( #150936, #175204, #173672 ) ) ;
#36982=EDGE_CURVE ( 'NONE', #181665, #176716, #224646, .T. ) ;
#36990=ORIENTED_EDGE ( 'NONE', *, *, #106225, .T. ) ;
#37001=ORIENTED_EDGE ( 'NONE', *, *, #73680, .F. ) ;
#37013=AXIS2_PLACEMENT_3D ( 'NONE', #222392, #161179, #144153 ) ;
#37062=LINE ( 'NONE', #196113, #55170 ) ;
#37073=CIRCLE ( 'NONE', #232693, 0.09999999999999939493 ) ;
#37080=AXIS2_PLACEMENT_3D ( 'NONE', #99239, #237492, #217898 ) ;
#37082=ORIENTED_EDGE ( 'NONE', *, *, #122782, .T. ) ;
#37087=VERTEX_POINT ( 'NONE', #63738 ) ;
#37112=DIRECTION ( 'NONE',  ( -1.000000000000000000, 0.000000000000000000, 0.000000000000000000 ) ) ;
#37116=ORIENTED_EDGE ( 'NONE', *, *, #125912, .F. ) ;
#37165=FACE_OUTER_BOUND ( 'NONE', #199915, .T. ) ;
#37183=DIRECTION ( 'NONE',  ( 0.000000000000000000, -0.000000000000000000, -1.000000000000000000 ) ) ;
#37189=EDGE_CURVE ( 'NONE', #217337, #58261, #244941, .T. ) ;
#37202=CARTESIAN_POINT ( 'NONE',  ( -18.59999999999999787, -10.80884033489985363, 6.100000000000002309 ) ) ;
#37228=CARTESIAN_POINT ( 'NONE',  ( -18.69999999999999929, -1.212568896937008089, -8.000000000000000000 ) ) ;
#37256=ADVANCED_FACE ( 'NONE', ( #25912 ), #85837, .T. ) ;
#37264=CARTESIAN_POINT ( 'NONE',  ( 18.79999999999999716, 11.59510167572422112, -1.901609089591594470 ) ) ;
#37271=AXIS2_PLACEMENT_3D ( 'NONE', #157148, #197523, #18890 ) ;
#37279=CARTESIAN_POINT ( 'NONE',  ( 18.69999999999999929, -8.250000000000005329, 32.89999999999999858 ) ) ;
#37285=EDGE_CURVE ( 'NONE', #214793, #89225, #229120, .T. ) ;
#37298=DIRECTION ( 'NONE',  ( -0.000000000000000000, -1.000000000000000000, 0.000000000000000000 ) ) ;
#37344=ORIENTED_EDGE ( 'NONE', *, *, #141720, .F. ) ;
#37372=DIRECTION ( 'NONE',  ( 0.000000000000000000, -1.000000000000000000, 0.000000000000000000 ) ) ;
#37413=LINE ( 'NONE', #58216, #22552 ) ;
#37452=DIRECTION ( 'NONE',  ( 0.000000000000000000, -0.9910465087640860649, 0.1335171055202901413 ) ) ;
#37486=ORIENTED_EDGE ( 'NONE', *, *, #148673, .T. ) ;
#37498=CARTESIAN_POINT ( 'NONE',  ( -21.00000000000000000, 6.258114003436813455, 11.90000000000000036 ) ) ;
#37532=DIRECTION ( 'NONE',  ( 0.000000000000000000, 0.000000000000000000, 1.000000000000000000 ) ) ;
#37549=EDGE_CURVE ( 'NONE', #182139, #149370, #85199, .T. ) ;
#37572=CARTESIAN_POINT ( 'NONE',  ( -18.79999999999999716, 1.250000000000000000, 0.000000000000000000 ) ) ;
#37585=CARTESIAN_POINT ( 'NONE',  ( -22.94999999999999929, -1.885425182446134107, -11.49641995933507843 ) ) ;
#37595=ORIENTED_EDGE ( 'NONE', *, *, #172799, .T. ) ;
#37609=DIRECTION ( 'NONE',  ( 0.000000000000000000, 0.000000000000000000, -1.000000000000000000 ) ) ;
#37656=CARTESIAN_POINT ( 'NONE',  ( -5.900000000000002132, -11.25000000000000000, 13.90000000000000213 ) ) ;
#37687=ORIENTED_EDGE ( 'NONE', *, *, #236033, .F. ) ;
#37708=ORIENTED_EDGE ( 'NONE', *, *, #86373, .T. ) ;
#37930=VERTEX_POINT ( 'NONE', #84891 ) ;
#37931=DIRECTION ( 'NONE',  ( -0.000000000000000000, 1.000000000000000000, -0.000000000000000000 ) ) ;
#37981=VECTOR ( 'NONE', #32233, 1000.000000000000000 ) ;
#37994=CIRCLE ( 'NONE', #108709, 11.65000000000000036 ) ;
#37999=CARTESIAN_POINT ( 'NONE',  ( 6.099999999999997868, -11.65000000000000036, 13.90000000000000213 ) ) ;
#38017=DIRECTION ( 'NONE',  ( 0.000000000000000000, -0.000000000000000000, -1.000000000000000000 ) ) ;
#38128=AXIS2_PLACEMENT_3D ( 'NONE', #215146, #133055, #233451 ) ;
#38169=VECTOR ( 'NONE', #222182, 1000.000000000000000 ) ;
#38200=ADVANCED_FACE ( 'NONE', ( #209565 ), #229503, .T. ) ;
#38224=AXIS2_PLACEMENT_3D ( 'NONE', #75066, #225429, #154604 ) ;
#38254=EDGE_CURVE ( 'NONE', #66395, #242362, #131302, .T. ) ;
#38290=AXIS2_PLACEMENT_3D ( 'NONE', #208713, #190437, #30085 ) ;
#38299=ADVANCED_FACE ( 'NONE', ( #34807 ), #76457, .F. ) ;
#38337=DIRECTION ( 'NONE',  ( 0.000000000000000000, 0.000000000000000000, 1.000000000000000000 ) ) ;
#38392=DIRECTION ( 'NONE',  ( 0.000000000000000000, 0.000000000000000000, 1.000000000000000000 ) ) ;
#38407=DIRECTION ( 'NONE',  ( -0.000000000000000000, -1.734723475976817507E-14, 1.000000000000000000 ) ) ;
#38447=CARTESIAN_POINT ( 'NONE',  ( -0.8999999999999993561, -11.65000000000000036, 23.30000000000000426 ) ) ;
#38455=ADVANCED_FACE ( 'NONE', ( #30757 ), #71160, .T. ) ;
#38490=ORIENTED_EDGE ( 'NONE', *, *, #154004, .F. ) ;
#38494=DIRECTION ( 'NONE',  ( 0.000000000000000000, 0.000000000000000000, 1.000000000000000000 ) ) ;
#38500=EDGE_CURVE ( 'NONE', #91491, #173345, #137507, .T. ) ;
#38514=ADVANCED_FACE ( 'NONE', ( #37165 ), #171556, .T. ) ;
#38534=CARTESIAN_POINT ( 'NONE',  ( 18.79999999999999716, 11.50977166988710820, 1.786320531569725478 ) ) ;
#38565=DIRECTION ( 'NONE',  ( 0.000000000000000000, 0.000000000000000000, 1.000000000000000000 ) ) ;
#38571=DIRECTION ( 'NONE',  ( -0.000000000000000000, 1.000000000000000000, -5.204170427930272977E-14 ) ) ;
#38608=CIRCLE ( 'NONE', #184338, 0.1000000000000002554 ) ;
#38610=DIRECTION ( 'NONE',  ( 0.000000000000000000, 0.000000000000000000, 1.000000000000000000 ) ) ;
#38623=EDGE_CURVE ( 'NONE', #223175, #82512, #20162, .T. ) ;
#38632=CIRCLE ( 'NONE', #100936, 0.09999999999999939493 ) ;
#38753=ORIENTED_EDGE ( 'NONE', *, *, #152466, .T. ) ;
#38764=CARTESIAN_POINT ( 'NONE',  ( -18.70000000000000284, 7.986648289447971116, -1.311673547813416718 ) ) ;
#38774=EDGE_CURVE ( 'NONE', #136069, #212664, #242794, .T. ) ;
#38853=LINE ( 'NONE', #37572, #2798 ) ;
#38863=FACE_OUTER_BOUND ( 'NONE', #40628, .T. ) ;
#38871=EDGE_LOOP ( 'NONE', ( #63338, #223007, #89737, #211927 ) ) ;
#38920=AXIS2_PLACEMENT_3D ( 'NONE', #158178, #236379, #57729 ) ;
#38945=VERTEX_POINT ( 'NONE', #232501 ) ;
#38955=CYLINDRICAL_SURFACE ( 'NONE', #138926, 0.09999999999999939493 ) ;
#38962=CARTESIAN_POINT ( 'NONE',  ( -21.00000000000000000, -1.885425182446133885, -11.49641995933507843 ) ) ;
#38964=ORIENTED_EDGE ( 'NONE', *, *, #13639, .T. ) ;
#38968=FACE_OUTER_BOUND ( 'NONE', #82031, .T. ) ;
#38972=AXIS2_PLACEMENT_3D ( 'NONE', #104642, #5556, #44719 ) ;
#38986=EDGE_LOOP ( 'NONE', ( #194711, #253125, #136962, #235214 ) ) ;
#39090=TOROIDAL_SURFACE ( 'NONE', #51496, 3.900000000000000355, 0.1000000000000000056 ) ;
#39187=CARTESIAN_POINT ( 'NONE',  ( -18.69999999999999929, -8.250000000000005329, 32.89999999999999858 ) ) ;
#39190=VERTEX_POINT ( 'NONE', #86210 ) ;
#39213=AXIS2_PLACEMENT_3D ( 'NONE', #189894, #88191, #107783 ) ;
#39266=ORIENTED_EDGE ( 'NONE', *, *, #128534, .T. ) ;
#39271=ORIENTED_EDGE ( 'NONE', *, *, #31759, .T. ) ;
#39277=VECTOR ( 'NONE', #453, 1000.000000000000000 ) ;
#39285=CARTESIAN_POINT ( 'NONE',  ( 22.84999999999999787, 0.000000000000000000, 0.000000000000000000 ) ) ;
#39381=CARTESIAN_POINT ( 'NONE',  ( -18.69999999999999929, 7.799999999999999822, -1.212568896937008089 ) ) ;
#39401=AXIS2_PLACEMENT_3D ( 'NONE', #94332, #190912, #12264 ) ;
#39451=CARTESIAN_POINT ( 'NONE',  ( -22.94999999999999929, 1.885425182446134107, -11.49641995933507843 ) ) ;
#39492=FACE_OUTER_BOUND ( 'NONE', #108180, .T. ) ;
#39495=ORIENTED_EDGE ( 'NONE', *, *, #101176, .F. ) ;
#39504=ORIENTED_EDGE ( 'NONE', *, *, #234376, .T. ) ;
#39528=EDGE_CURVE ( 'NONE', #97490, #98150, #7188, .T. ) ;
#39540=CARTESIAN_POINT ( 'NONE',  ( -11.60000000000000320, -11.65000000000000036, 12.30000000000000426 ) ) ;
#39587=ORIENTED_EDGE ( 'NONE', *, *, #152429, .T. ) ;
#39588=CIRCLE ( 'NONE', #39401, 0.09999999999999939493 ) ;
#39609=DIRECTION ( 'NONE',  ( 1.000000000000000000, 0.000000000000000000, 0.000000000000000000 ) ) ;
#39655=ORIENTED_EDGE ( 'NONE', *, *, #102530, .T. ) ;
#39681=DIRECTION ( 'NONE',  ( 0.000000000000000000, 0.1618390714546129594, 0.9868171638914214894 ) ) ;
#39708=DIRECTION ( 'NONE',  ( -1.000000000000000000, 8.673617379884087537E-15, 0.000000000000000000 ) ) ;
#39719=DIRECTION ( 'NONE',  ( 0.000000000000000000, 1.000000000000000000, 1.734723475976817507E-14 ) ) ;
#39786=AXIS2_PLACEMENT_3D ( 'NONE', #54456, #88422, #49324 ) ;
#39802=DIRECTION ( 'NONE',  ( -0.000000000000000000, 1.000000000000000000, -0.000000000000000000 ) ) ;
#39867=ORIENTED_EDGE ( 'NONE', *, *, #138799, .T. ) ;
#39925=DIRECTION ( 'NONE',  ( -0.000000000000000000, -0.1335171055202867274, 0.9910465087640865089 ) ) ;
#39939=AXIS2_PLACEMENT_3D ( 'NONE', #135505, #33911, #113398 ) ;
#39965=EDGE_CURVE ( 'NONE', #75205, #89756, #146535, .T. ) ;
#39971=ORIENTED_EDGE ( 'NONE', *, *, #120981, .T. ) ;
#40010=ORIENTED_EDGE ( 'NONE', *, *, #125412, .F. ) ;
#40024=CARTESIAN_POINT ( 'NONE',  ( -18.79999999999999716, 11.49641995933507843, 1.885425182446133885 ) ) ;
#40078=EDGE_CURVE ( 'NONE', #171414, #83713, #3268, .T. ) ;
#40088=VECTOR ( 'NONE', #3558, 1000.000000000000000 ) ;
#40132=DIRECTION ( 'NONE',  ( 0.000000000000000000, 1.000000000000000000, 0.000000000000000000 ) ) ;
#40143=CARTESIAN_POINT ( 'NONE',  ( -21.00000000000000000, -11.65000000000000036, 0.000000000000000000 ) ) ;
#40161=DIRECTION ( 'NONE',  ( -1.000000000000000000, 0.000000000000000000, 0.000000000000000000 ) ) ;
#40170=AXIS2_PLACEMENT_3D ( 'NONE', #223435, #158380, #39708 ) ;
#40179=CARTESIAN_POINT ( 'NONE',  ( 20.90000000000000213, 0.000000000000000000, 0.000000000000000000 ) ) ;
#40182=EDGE_LOOP ( 'NONE', ( #257637, #88340, #208008, #9748 ) ) ;
#40184=ADVANCED_FACE ( 'NONE', ( #39492 ), #139823, .F. ) ;
#40249=DIRECTION ( 'NONE',  ( 0.000000000000000000, -0.7071067811865472397, -0.7071067811865479058 ) ) ;
#40279=ORIENTED_EDGE ( 'NONE', *, *, #137120, .T. ) ;
#40312=DIRECTION ( 'NONE',  ( 1.000000000000000000, -0.000000000000000000, 0.000000000000000000 ) ) ;
#40324=ADVANCED_FACE ( 'NONE', ( #49722 ), #195035, .F. ) ;
#40362=ORIENTED_EDGE ( 'NONE', *, *, #197254, .T. ) ;
#40397=ORIENTED_EDGE ( 'NONE', *, *, #134654, .F. ) ;
#40409=CARTESIAN_POINT ( 'NONE',  ( -22.94999999999999929, -1.467286812112899463, 33.00000000000000000 ) ) ;
#40419=DIRECTION ( 'NONE',  ( 1.000000000000000000, -0.000000000000000000, -0.000000000000000000 ) ) ;
#40449=VERTEX_POINT ( 'NONE', #130536 ) ;
#40480=CIRCLE ( 'NONE', #186182, 2.600000000000001421 ) ;
#40538=ORIENTED_EDGE ( 'NONE', *, *, #49497, .F. ) ;
#40548=PLANE ( 'NONE',  #47460 ) ;
#40595=ORIENTED_EDGE ( 'NONE', *, *, #165458, .F. ) ;
#40605=DIRECTION ( 'NONE',  ( 1.000000000000000000, 0.000000000000000000, 0.000000000000000000 ) ) ;
#40624=VECTOR ( 'NONE', #86802, 1000.000000000000000 ) ;
#40628=EDGE_LOOP ( 'NONE', ( #75369, #222730, #246077, #5907 ) ) ;
#40638=CARTESIAN_POINT ( 'NONE',  ( 18.69999999999999929, -10.80884033489985363, 6.100000000000002309 ) ) ;
#40639=CARTESIAN_POINT ( 'NONE',  ( 18.59999999999999787, -10.63400887967554986, 6.002871413764276909 ) ) ;
#40687=AXIS2_PLACEMENT_3D ( 'NONE', #98252, #141275, #79985 ) ;
#40698=EDGE_LOOP ( 'NONE', ( #212093, #226320, #11255, #249007 ) ) ;
#40700=DIRECTION ( 'NONE',  ( 1.000000000000000000, 0.000000000000000000, 0.000000000000000000 ) ) ;
#40737=CARTESIAN_POINT ( 'NONE',  ( 19.90000000000000568, 1.250000000000000000, 16.60000000000000142 ) ) ;
#40749=DIRECTION ( 'NONE',  ( -1.000000000000000000, -0.000000000000000000, -0.000000000000000000 ) ) ;
#40757=VECTOR ( 'NONE', #245662, 1000.000000000000000 ) ;
#40856=DIRECTION ( 'NONE',  ( 1.476360405086644309E-16, 1.000000000000000000, 0.000000000000000000 ) ) ;
#40857=EDGE_LOOP ( 'NONE', ( #246100, #4955, #187784, #221685 ) ) ;
#40887=EDGE_CURVE ( 'NONE', #192176, #205125, #214904, .T. ) ;
#40917=DIRECTION ( 'NONE',  ( 1.476360405086644309E-16, 1.000000000000000000, 1.445602896647339410E-16 ) ) ;
#40945=CIRCLE ( 'NONE', #182593, 0.1000000000000002554 ) ;
#40962=DIRECTION ( 'NONE',  ( 0.000000000000000000, 0.000000000000000000, 1.000000000000000000 ) ) ;
#40993=AXIS2_PLACEMENT_3D ( 'NONE', #111685, #15167, #32178 ) ;
#41021=CARTESIAN_POINT ( 'NONE',  ( -0.8999999999999986899, -12.25000000000000355, 26.00000000000000355 ) ) ;
#41023=VECTOR ( 'NONE', #27495, 1000.000000000000000 ) ;
#41053=DIRECTION ( 'NONE',  ( 0.000000000000000000, -0.000000000000000000, 1.000000000000000000 ) ) ;
#41107=VERTEX_POINT ( 'NONE', #102627 ) ;
#41110=CARTESIAN_POINT ( 'NONE',  ( -19.89999999999999858, 1.350000000000000089, 22.00000000000000355 ) ) ;
#41125=ORIENTED_EDGE ( 'NONE', *, *, #11936, .T. ) ;
#41152=ORIENTED_EDGE ( 'NONE', *, *, #144624, .T. ) ;
#41173=CARTESIAN_POINT ( 'NONE',  ( -22.94999999999999929, 0.000000000000000000, 0.000000000000000000 ) ) ;
#41190=CARTESIAN_POINT ( 'NONE',  ( -22.94999999999999929, 11.50977166988710820, -1.786320531569725478 ) ) ;
#41195=PLANE ( 'NONE',  #63104 ) ;
#41215=EDGE_CURVE ( 'NONE', #243832, #106026, #13835, .T. ) ;
#41229=DIRECTION ( 'NONE',  ( 0.000000000000000000, 0.000000000000000000, 1.000000000000000000 ) ) ;
#41292=VERTEX_POINT ( 'NONE', #38534 ) ;
#41455=DIRECTION ( 'NONE',  ( 0.000000000000000000, 0.000000000000000000, -1.000000000000000000 ) ) ;
#41488=DIRECTION ( 'NONE',  ( -0.000000000000000000, 1.000000000000000000, -0.000000000000000000 ) ) ;
#41490=ORIENTED_EDGE ( 'NONE', *, *, #111257, .T. ) ;
#41516=VERTEX_POINT ( 'NONE', #65796 ) ;
#41558=EDGE_LOOP ( 'NONE', ( #96267, #219670, #235115, #129440 ) ) ;
#41601=ORIENTED_EDGE ( 'NONE', *, *, #11976, .F. ) ;
#41604=FACE_OUTER_BOUND ( 'NONE', #166671, .T. ) ;
#41626=ORIENTED_EDGE ( 'NONE', *, *, #257812, .T. ) ;
#41643=ORIENTED_EDGE ( 'NONE', *, *, #87223, .F. ) ;
#41707=AXIS2_PLACEMENT_3D ( 'NONE', #95259, #75712, #52261 ) ;
#41717=ADVANCED_FACE ( 'NONE', ( #179996 ), #43047, .T. ) ;
#41750=CARTESIAN_POINT ( 'NONE',  ( -18.79999999999999716, 0.000000000000000000, 33.00000000000000000 ) ) ;
#41791=DIRECTION ( 'NONE',  ( 0.000000000000000000, 0.000000000000000000, 1.000000000000000000 ) ) ;
#41890=EDGE_CURVE ( 'NONE', #28763, #214793, #173312, .T. ) ;
#41910=AXIS2_PLACEMENT_3D ( 'NONE', #199421, #76873, #58584 ) ;
#41916=EDGE_CURVE ( 'NONE', #144975, #98899, #66184, .T. ) ;
#41992=CYLINDRICAL_SURFACE ( 'NONE', #70320, 2.600000000000001421 ) ;
#42000=DIRECTION ( 'NONE',  ( 0.000000000000000000, 0.000000000000000000, -1.000000000000000000 ) ) ;
#42012=DIRECTION ( 'NONE',  ( 1.000000000000000000, 0.000000000000000000, 0.000000000000000000 ) ) ;
#42016=EDGE_LOOP ( 'NONE', ( #42909, #85309, #91659, #158564 ) ) ;
#42045=ORIENTED_EDGE ( 'NONE', *, *, #123320, .F. ) ;
#42052=CARTESIAN_POINT ( 'NONE',  ( -0.8999999999999993561, -11.75000000000000000, 26.00000000000000355 ) ) ;
#42055=CARTESIAN_POINT ( 'NONE',  ( 22.10000000000000497, -11.65000000000000036, 12.09999999999999609 ) ) ;
#42102=CARTESIAN_POINT ( 'NONE',  ( 20.90000000000000213, 11.49641995933507843, -1.885425182446133885 ) ) ;
#42122=AXIS2_PLACEMENT_3D ( 'NONE', #110213, #208062, #108930 ) ;
#42146=CARTESIAN_POINT ( 'NONE',  ( -22.10000000000000497, 11.99999999999999822, 12.09999999999999964 ) ) ;
#42166=DIRECTION ( 'NONE',  ( 0.000000000000000000, 0.000000000000000000, -1.000000000000000000 ) ) ;
#42179=ADVANCED_FACE ( 'NONE', ( #185867, #170217, #244551, #129748, #5926 ), #31962, .T. ) ;
#42232=ORIENTED_EDGE ( 'NONE', *, *, #199238, .T. ) ;
#42246=ORIENTED_EDGE ( 'NONE', *, *, #96401, .F. ) ;
#42294=PLANE ( 'NONE',  #13853 ) ;
#42295=CYLINDRICAL_SURFACE ( 'NONE', #150579, 0.09999999999999933942 ) ;
#42319=EDGE_CURVE ( 'NONE', #166243, #157545, #52764, .T. ) ;
#42367=CARTESIAN_POINT ( 'NONE',  ( 22.84999999999999787, 0.000000000000000000, -3.900000000000000355 ) ) ;
#42394=VERTEX_POINT ( 'NONE', #54058 ) ;
#42397=ORIENTED_EDGE ( 'NONE', *, *, #60668, .T. ) ;
#42400=AXIS2_PLACEMENT_3D ( 'NONE', #139201, #98775, #40161 ) ;
#42465=CARTESIAN_POINT ( 'NONE',  ( -18.59999999999999787, -10.74999999999999289, 32.89999999999999858 ) ) ;
#42511=AXIS2_PLACEMENT_3D ( 'NONE', #186972, #229925, #107397 ) ;
#42523=CARTESIAN_POINT ( 'NONE',  ( -18.69999999999999929, -8.250000000000005329, 5.900000000000002132 ) ) ;
#42540=DIRECTION ( 'NONE',  ( 1.000000000000000000, 0.000000000000000000, 0.000000000000000000 ) ) ;
#42561=EDGE_CURVE ( 'NONE', #166926, #247506, #7949, .T. ) ;
#42567=CIRCLE ( 'NONE', #188314, 0.09999999999999939493 ) ;
#42699=VECTOR ( 'NONE', #79242, 1000.000000000000000 ) ;
#42710=DIRECTION ( 'NONE',  ( 1.284434275755705296E-16, -0.7071067811865471286, 0.7071067811865479058 ) ) ;
#42752=VECTOR ( 'NONE', #127288, 1000.000000000000114 ) ;
#42798=EDGE_LOOP ( 'NONE', ( #210946, #243300, #119949, #218276 ) ) ;
#42817=EDGE_CURVE ( 'NONE', #21663, #253988, #101519, .T. ) ;
#42822=DIRECTION ( 'NONE',  ( 0.000000000000000000, 0.9910465087640866200, -0.1335171055202867274 ) ) ;
#42856=CARTESIAN_POINT ( 'NONE',  ( -19.99999999999999645, 4.527376849368447864, 21.95857864376269220 ) ) ;
#42876=ORIENTED_EDGE ( 'NONE', *, *, #112527, .T. ) ;
#42909=ORIENTED_EDGE ( 'NONE', *, *, #284, .T. ) ;
#42911=EDGE_LOOP ( 'NONE', ( #37708, #203014, #146495, #101341 ) ) ;
#42945=AXIS2_PLACEMENT_3D ( 'NONE', #85752, #165336, #145750 ) ;
#43015=CARTESIAN_POINT ( 'NONE',  ( 18.79999999999999716, 4.513204987021264714, 22.10000000000000142 ) ) ;
#43023=PLANE ( 'NONE',  #132769 ) ;
#43025=DIRECTION ( 'NONE',  ( 1.000000000000000000, -0.000000000000000000, -0.000000000000000000 ) ) ;
#43047=CYLINDRICAL_SURFACE ( 'NONE', #108282, 0.09999999999999939493 ) ;
#43062=FACE_BOUND ( 'NONE', #173109, .T. ) ;
#43073=DIRECTION ( 'NONE',  ( -1.000000000000000000, 0.000000000000000000, 0.000000000000000000 ) ) ;
#43082=CIRCLE ( 'NONE', #247060, 0.09999999999999939493 ) ;
#43187=DIRECTION ( 'NONE',  ( -1.000000000000000000, 0.000000000000000000, 0.000000000000000000 ) ) ;
#43191=ORIENTED_EDGE ( 'NONE', *, *, #157121, .F. ) ;
#43204=DIRECTION ( 'NONE',  ( 1.000000000000000000, 0.000000000000000000, 0.000000000000000000 ) ) ;
#43214=VECTOR ( 'NONE', #231323, 1000.000000000000114 ) ;
#43229=CIRCLE ( 'NONE', #155685, 0.09999999999999939493 ) ;
#43261=EDGE_CURVE ( 'NONE', #83237, #173524, #224932, .T. ) ;
#43263=CARTESIAN_POINT ( 'NONE',  ( 18.69999999999999929, 1.350000000000000089, 16.39999999999999858 ) ) ;
#43303=( BOUNDED_SURFACE ( )  B_SPLINE_SURFACE ( 3, 2, ( 
 ( #154896, #31105, #194008 ),
 ( #50608, #15372, #130154 ),
 ( #10231, #174484, #234386 ),
 ( #135278, #89739, #37498 ) ),
 .UNSPECIFIED., .F., .F., .F. ) 
 B_SPLINE_SURFACE_WITH_KNOTS ( ( 4, 4 ),
 ( 3, 3 ),
 ( 0.000000000000000000, 1.570796326794896558 ),
 ( 0.000000000000000000, 1.000000000000000000 ),
 .UNSPECIFIED. ) 
 GEOMETRIC_REPRESENTATION_ITEM ( )  RATIONAL_B_SPLINE_SURFACE ( (
 ( 1.000000000000000000, 0.6447402616205117898, 1.000000000000000000),
 ( 1.000000000000000000, 0.6438648806865400198, 1.000000000000000000),
 ( 1.000000000000000000, 0.6753870962079631113, 1.000000000000000000),
 ( 1.000000000000000000, 0.7071067811865505703, 1.000000000000000000) ) ) 
 REPRESENTATION_ITEM ( '' )  SURFACE ( )  );
#43311=ADVANCED_FACE ( 'NONE', ( #226306 ), #120747, .T. ) ;
#43340=( BOUNDED_CURVE ( )  B_SPLINE_CURVE ( 3, ( #58768, #222992, #92, #24837 ),
 .UNSPECIFIED., .F., .F. ) 
 B_SPLINE_CURVE_WITH_KNOTS ( ( 4, 4 ),
 ( 0.000000000000000000, 1.570796326794896558 ),
 .UNSPECIFIED. ) 
 CURVE ( )  GEOMETRIC_REPRESENTATION_ITEM ( )  RATIONAL_B_SPLINE_CURVE ( ( 1.000000000000000000, 0.8047378541243649375, 0.8047378541243649375, 1.000000000000000000 ) ) 
 REPRESENTATION_ITEM ( '' )  );
#43369=CARTESIAN_POINT ( 'NONE',  ( 18.59999999999999787, -8.150000000000007461, -15.00000000000000000 ) ) ;
#43475=DIRECTION ( 'NONE',  ( 1.000000000000000000, -0.000000000000000000, -0.000000000000000000 ) ) ;
#43481=DIRECTION ( 'NONE',  ( 1.472176885922364728E-15, -0.9868171638914230437, 0.1618390714546045217 ) ) ;
#43483=AXIS2_PLACEMENT_3D ( 'NONE', #24251, #107612, #103732 ) ;
#43568=AXIS2_PLACEMENT_3D ( 'NONE', #240962, #62325, #141846 ) ;
#43629=CIRCLE ( 'NONE', #85286, 0.1000000000000028644 ) ;
#43650=AXIS2_PLACEMENT_3D ( 'NONE', #63568, #143099, #146946 ) ;
#43657=DIRECTION ( 'NONE',  ( 0.000000000000000000, 0.000000000000000000, -1.000000000000000000 ) ) ;
#43697=ADVANCED_FACE ( 'NONE', ( #169953 ), #26559, .T. ) ;
#43715=CYLINDRICAL_SURFACE ( 'NONE', #147872, 0.09999999999999939493 ) ;
#43719=EDGE_LOOP ( 'NONE', ( #39971, #203583, #194083, #196701 ) ) ;
#43720=CARTESIAN_POINT ( 'NONE',  ( 20.90000000000000213, 6.726092018229619995, 9.512212474619552438 ) ) ;
#43723=DIRECTION ( 'NONE',  ( -0.000000000000000000, -0.000000000000000000, 1.000000000000000000 ) ) ;
#43756=ORIENTED_EDGE ( 'NONE', *, *, #67311, .F. ) ;
#43769=AXIS2_PLACEMENT_3D ( 'NONE', #252860, #175929, #157666 ) ;
#43774=ORIENTED_EDGE ( 'NONE', *, *, #2924, .F. ) ;
#43797=CARTESIAN_POINT ( 'NONE',  ( -22.94999999999999929, 8.000000000000000000, 1.212568896937007867 ) ) ;
#43831=ORIENTED_EDGE ( 'NONE', *, *, #179370, .T. ) ;
#43833=AXIS2_PLACEMENT_3D ( 'NONE', #188965, #15482, #37609 ) ;
#43899=ORIENTED_EDGE ( 'NONE', *, *, #181764, .F. ) ;
#44015=LINE ( 'NONE', #45303, #152010 ) ;
#44050=LINE ( 'NONE', #165275, #47804 ) ;
#44143=LINE ( 'NONE', #100226, #248932 ) ;
#44161=DIRECTION ( 'NONE',  ( 0.000000000000000000, 1.000000000000000000, 0.000000000000000000 ) ) ;
#44166=DIRECTION ( 'NONE',  ( -1.000000000000000000, 0.000000000000000000, -0.000000000000000000 ) ) ;
#44185=ADVANCED_FACE ( 'NONE', ( #160004 ), #174463, .T. ) ;
#44200=FACE_OUTER_BOUND ( 'NONE', #175874, .T. ) ;
#44202=CARTESIAN_POINT ( 'NONE',  ( 13.40000000000000036, -12.24999999999999822, 15.00000000000000355 ) ) ;
#44211=FACE_OUTER_BOUND ( 'NONE', #54607, .T. ) ;
#44236=DIRECTION ( 'NONE',  ( 0.000000000000000000, 0.000000000000000000, 1.000000000000000000 ) ) ;
#44278=AXIS2_PLACEMENT_3D ( 'NONE', #184414, #202694, #27953 ) ;
#44304=FACE_OUTER_BOUND ( 'NONE', #192833, .T. ) ;
#44316=CARTESIAN_POINT ( 'NONE',  ( 19.95857864376269575, 4.513204987021262937, 22.00000000000000355 ) ) ;
#44492=CYLINDRICAL_SURFACE ( 'NONE', #31237, 0.09999999999999939493 ) ;
#44529=CARTESIAN_POINT ( 'NONE',  ( 21.10000000000000142, -11.65000000000000036, 11.89999999999999680 ) ) ;
#44531=ORIENTED_EDGE ( 'NONE', *, *, #167281, .T. ) ;
#44573=EDGE_CURVE ( 'NONE', #88949, #22117, #34613, .T. ) ;
#44579=CARTESIAN_POINT ( 'NONE',  ( 18.69999999999999929, 11.75000000000000000, 16.39999999999999858 ) ) ;
#44613=ORIENTED_EDGE ( 'NONE', *, *, #217459, .T. ) ;
#44623=ORIENTED_EDGE ( 'NONE', *, *, #205890, .F. ) ;
#44651=CARTESIAN_POINT ( 'NONE',  ( -18.69999999999999929, 11.49641995933507843, 1.885425182446135661 ) ) ;
#44672=ADVANCED_FACE ( 'NONE', ( #222185 ), #83935, .T. ) ;
#44673=EDGE_CURVE ( 'NONE', #171946, #132097, #196451, .T. ) ;
#44694=CARTESIAN_POINT ( 'NONE',  ( -5.900000000000002132, -11.34999999999999964, 13.90000000000000213 ) ) ;
#44698=CARTESIAN_POINT ( 'NONE',  ( -18.79999999999999716, -10.13229168743236031, -1.028467303599445826 ) ) ;
#44719=DIRECTION ( 'NONE',  ( 0.000000000000000000, 0.000000000000000000, -1.000000000000000000 ) ) ;
#44725=EDGE_LOOP ( 'NONE', ( #51780, #164781, #231790, #73583 ) ) ;
#44767=EDGE_CURVE ( 'NONE', #12756, #176282, #175633, .T. ) ;
#44771=ORIENTED_EDGE ( 'NONE', *, *, #37549, .F. ) ;
#44778=EDGE_CURVE ( 'NONE', #223079, #208058, #13311, .T. ) ;
#44788=CARTESIAN_POINT ( 'NONE',  ( -18.69999999999999929, 8.000000000000000000, -1.212568896937008089 ) ) ;
#44815=DIRECTION ( 'NONE',  ( 0.000000000000000000, 0.000000000000000000, -1.000000000000000000 ) ) ;
#44902=VERTEX_POINT ( 'NONE', #117674 ) ;
#44910=ORIENTED_EDGE ( 'NONE', *, *, #54077, .F. ) ;
#44934=AXIS2_PLACEMENT_3D ( 'NONE', #85181, #8268, #44815 ) ;
#44955=ORIENTED_EDGE ( 'NONE', *, *, #121810, .T. ) ;
#45031=EDGE_CURVE ( 'NONE', #70728, #78387, #13504, .T. ) ;
#45035=DIRECTION ( 'NONE',  ( -1.000000000000000000, 0.000000000000000000, 0.000000000000000000 ) ) ;
#45068=VERTEX_POINT ( 'NONE', #2843 ) ;
#45102=ORIENTED_EDGE ( 'NONE', *, *, #141554, .F. ) ;
#45110=EDGE_CURVE ( 'NONE', #163777, #88476, #103225, .T. ) ;
#45123=DIRECTION ( 'NONE',  ( 1.000000000000000000, 0.000000000000000000, 0.000000000000000000 ) ) ;
#45132=CIRCLE ( 'NONE', #65791, 0.09999999999999939493 ) ;
#45142=EDGE_LOOP ( 'NONE', ( #31202, #163868, #210885, #212773 ) ) ;
#45153=AXIS2_PLACEMENT_3D ( 'NONE', #231397, #112724, #137403 ) ;
#45164=LINE ( 'NONE', #127275, #167340 ) ;
#45185=DIRECTION ( 'NONE',  ( 0.000000000000000000, 0.9868171638914228216, 0.1618390714546044939 ) ) ;
#45197=EDGE_CURVE ( 'NONE', #189583, #150585, #117726, .T. ) ;
#45208=DIRECTION ( 'NONE',  ( 0.000000000000000000, 0.9868171638914221555, 0.1618390714546086850 ) ) ;
#45226=EDGE_LOOP ( 'NONE', ( #86052, #146347, #245129, #84604 ) ) ;
#45235=DIRECTION ( 'NONE',  ( -0.000000000000000000, -0.000000000000000000, 1.000000000000000000 ) ) ;
#45240=CARTESIAN_POINT ( 'NONE',  ( -0.8999999999999986899, -8.350000000000004974, 30.04142135623731136 ) ) ;
#45275=ORIENTED_EDGE ( 'NONE', *, *, #233906, .F. ) ;
#45303=CARTESIAN_POINT ( 'NONE',  ( -0.8999999999999993561, -8.250000000000005329, 23.40000000000000568 ) ) ;
#45314=ORIENTED_EDGE ( 'NONE', *, *, #41215, .F. ) ;
#45320=VERTEX_POINT ( 'NONE', #122369 ) ;
#45326=LINE ( 'NONE', #186121, #112826 ) ;
#45386=DIRECTION ( 'NONE',  ( 0.000000000000000000, 0.9910465087640866200, 0.1335171055202867274 ) ) ;
#45391=FACE_OUTER_BOUND ( 'NONE', #109983, .T. ) ;
#45432=SPHERICAL_SURFACE ( 'NONE', #155145, 0.1000000000000000056 ) ;
#45447=DIRECTION ( 'NONE',  ( -0.000000000000000000, 0.1686199900910312910, -0.9856811345164826488 ) ) ;
#45450=DIRECTION ( 'NONE',  ( -0.000000000000000000, -0.000000000000000000, -1.000000000000000000 ) ) ;
#45458=EDGE_LOOP ( 'NONE', ( #234765, #50814, #188657, #212786, #76643, #147217, #244023, #254436, #209778, #126988, #106343, #65862, #93022 ) ) ;
#45463=AXIS2_PLACEMENT_3D ( 'NONE', #222937, #204654, #127713 ) ;
#45478=ORIENTED_EDGE ( 'NONE', *, *, #229119, .F. ) ;
#45492=ORIENTED_EDGE ( 'NONE', *, *, #195482, .F. ) ;
#45551=ORIENTED_EDGE ( 'NONE', *, *, #152843, .F. ) ;
#45562=CYLINDRICAL_SURFACE ( 'NONE', #34453, 0.1000000000000000472 ) ;
#45628=DIRECTION ( 'NONE',  ( 0.000000000000000000, 0.000000000000000000, 1.000000000000000000 ) ) ;
#45630=EDGE_CURVE ( 'NONE', #173345, #105678, #52853, .T. ) ;
#45652=EDGE_LOOP ( 'NONE', ( #198215, #182697, #10483, #25084 ) ) ;
#45674=LINE ( 'NONE', #125217, #209139 ) ;
#45685=ORIENTED_EDGE ( 'NONE', *, *, #219789, .F. ) ;
#45720=CARTESIAN_POINT ( 'NONE',  ( 20.90000000000000213, 6.336640076952988920, 12.03401928653448572 ) ) ;
#45722=EDGE_CURVE ( 'NONE', #211171, #221991, #217837, .T. ) ;
#45734=ORIENTED_EDGE ( 'NONE', *, *, #133590, .F. ) ;
#45754=CARTESIAN_POINT ( 'NONE',  ( -21.00000000000000000, -1.212568896937008089, -8.000000000000000000 ) ) ;
#45763=EDGE_CURVE ( 'NONE', #162415, #14083, #22251, .T. ) ;
#45777=VECTOR ( 'NONE', #8038, 1000.000000000000227 ) ;
#45786=FACE_OUTER_BOUND ( 'NONE', #57732, .T. ) ;
#45802=DIRECTION ( 'NONE',  ( 0.000000000000000000, 4.336808689942044242E-14, 1.000000000000000000 ) ) ;
#45809=ORIENTED_EDGE ( 'NONE', *, *, #200132, .T. ) ;
#45826=CARTESIAN_POINT ( 'NONE',  ( 5.899999999999996803, -11.65000000000000036, 13.90000000000000213 ) ) ;
#45909=CARTESIAN_POINT ( 'NONE',  ( -19.99016485861947601, 4.635725510443826636, 21.97684634237452528 ) ) ;
#45910=ADVANCED_FACE ( 'NONE', ( #103525 ), #42294, .F. ) ;
#45929=ORIENTED_EDGE ( 'NONE', *, *, #59149, .F. ) ;
#45936=VECTOR ( 'NONE', #142600, 1000.000000000000000 ) ;
#45979=DIRECTION ( 'NONE',  ( 1.000000000000000000, 0.000000000000000000, 0.000000000000000000 ) ) ;
#45997=VERTEX_POINT ( 'NONE', #30451 ) ;
#46028=ORIENTED_EDGE ( 'NONE', *, *, #156190, .F. ) ;
#46067=ORIENTED_EDGE ( 'NONE', *, *, #189737, .T. ) ;
#46077=ORIENTED_EDGE ( 'NONE', *, *, #157505, .T. ) ;
#46105=EDGE_CURVE ( 'NONE', #70370, #92927, #176067, .T. ) ;
#46114=ORIENTED_EDGE ( 'NONE', *, *, #214781, .T. ) ;
#46128=FACE_OUTER_BOUND ( 'NONE', #180322, .T. ) ;
#46186=ORIENTED_EDGE ( 'NONE', *, *, #104008, .F. ) ;
#46193=EDGE_CURVE ( 'NONE', #76759, #38945, #134811, .T. ) ;
#46200=ORIENTED_EDGE ( 'NONE', *, *, #16982, .F. ) ;
#46214=LINE ( 'NONE', #127048, #49199 ) ;
#46250=ORIENTED_EDGE ( 'NONE', *, *, #76402, .T. ) ;
#46280=VERTEX_POINT ( 'NONE', #170649 ) ;
#46374=VECTOR ( 'NONE', #4637, 1000.000000000000000 ) ;
#46401=VECTOR ( 'NONE', #210183, 1000.000000000000000 ) ;
#46456=AXIS2_PLACEMENT_3D ( 'NONE', #170906, #15660, #73076 ) ;
#46484=CIRCLE ( 'NONE', #58948, 0.09999999999999990841 ) ;
#46491=FACE_OUTER_BOUND ( 'NONE', #195481, .T. ) ;
#46511=DIRECTION ( 'NONE',  ( 0.000000000000000000, 0.000000000000000000, 1.000000000000000000 ) ) ;
#46592=AXIS2_PLACEMENT_3D ( 'NONE', #72152, #129547, #248206 ) ;
#46601=VERTEX_POINT ( 'NONE', #47746 ) ;
#46607=ADVANCED_FACE ( 'NONE', ( #206844 ), #101265, .T. ) ;
#46684=DIRECTION ( 'NONE',  ( -0.000000000000000000, 0.000000000000000000, -1.000000000000000000 ) ) ;
#46732=DIRECTION ( 'NONE',  ( 0.000000000000000000, 1.000000000000000000, 0.000000000000000000 ) ) ;
#46749=EDGE_CURVE ( 'NONE', #109914, #233154, #114155, .T. ) ;
#46814=FACE_OUTER_BOUND ( 'NONE', #50768, .T. ) ;
#46815=DIRECTION ( 'NONE',  ( 0.000000000000000000, 2.168404344971021884E-15, 1.000000000000000000 ) ) ;
#46838=CARTESIAN_POINT ( 'NONE',  ( 0.000000000000000000, 1.250000000000000000, 0.000000000000000000 ) ) ;
#46854=VECTOR ( 'NONE', #40856, 1000.000000000000000 ) ;
#46867=CARTESIAN_POINT ( 'NONE',  ( -18.79999999999999716, 1.250000000000000000, 21.90000000000000213 ) ) ;
#46885=ADVANCED_FACE ( 'NONE', ( #34649 ), #185093, .T. ) ;
#46911=FACE_OUTER_BOUND ( 'NONE', #222239, .T. ) ;
#46938=EDGE_CURVE ( 'NONE', #3738, #70370, #113785, .T. ) ;
#46972=CARTESIAN_POINT ( 'NONE',  ( -20.90000000000000213, 11.49641995933507843, -1.885425182446133885 ) ) ;
#46986=LINE ( 'NONE', #82247, #41023 ) ;
#47011=DIRECTION ( 'NONE',  ( -1.000000000000000000, 0.000000000000000000, 0.000000000000000000 ) ) ;
#47023=CARTESIAN_POINT ( 'NONE',  ( 20.90000000000000213, 1.899104650876408451, -11.59795743183152972 ) ) ;
#47024=FACE_OUTER_BOUND ( 'NONE', #131296, .T. ) ;
#47029=CIRCLE ( 'NONE', #180324, 0.09999999999999939493 ) ;
#47068=ADVANCED_FACE ( 'NONE', ( #128304 ), #84711, .T. ) ;
#47094=DIRECTION ( 'NONE',  ( 0.000000000000000000, 0.1335171055202901413, -0.9910465087640860649 ) ) ;
#47104=DIRECTION ( 'NONE',  ( 1.000000000000000000, 0.000000000000000000, 0.000000000000000000 ) ) ;
#47106=ORIENTED_EDGE ( 'NONE', *, *, #56128, .F. ) ;
#47140=VERTEX_POINT ( 'NONE', #67035 ) ;
#47259=ORIENTED_EDGE ( 'NONE', *, *, #256556, .F. ) ;
#47310=CARTESIAN_POINT ( 'NONE',  ( -13.40000000000000213, -11.75000000000000000, 12.30000000000000426 ) ) ;
#47323=AXIS2_PLACEMENT_3D ( 'NONE', #61344, #220430, #80887 ) ;
#47355=ORIENTED_EDGE ( 'NONE', *, *, #210423, .F. ) ;
#47359=CARTESIAN_POINT ( 'NONE',  ( 20.10000000000000497, 5.454087299794355914, 16.60000000000000142 ) ) ;
#47370=ORIENTED_EDGE ( 'NONE', *, *, #85271, .T. ) ;
#47380=AXIS2_PLACEMENT_3D ( 'NONE', #118866, #219219, #139668 ) ;
#47386=ADVANCED_FACE ( 'NONE', ( #50984 ), #168189, .F. ) ;
#47402=VECTOR ( 'NONE', #173971, 1000.000000000000000 ) ;
#47412=ORIENTED_EDGE ( 'NONE', *, *, #59997, .T. ) ;
#47460=AXIS2_PLACEMENT_3D ( 'NONE', #176185, #137038, #95343 ) ;
#47478=CARTESIAN_POINT ( 'NONE',  ( -22.10000000000000142, -11.65000000000000036, 12.09999999999999609 ) ) ;
#47514=LINE ( 'NONE', #184465, #223168 ) ;
#47555=FACE_OUTER_BOUND ( 'NONE', #128314, .T. ) ;
#47558=ORIENTED_EDGE ( 'NONE', *, *, #61719, .F. ) ;
#47632=AXIS2_PLACEMENT_3D ( 'NONE', #170772, #106882, #168198 ) ;
#47639=ORIENTED_EDGE ( 'NONE', *, *, #17270, .F. ) ;
#47661=CARTESIAN_POINT ( 'NONE',  ( -22.94999999999999929, 4.898587196589412829E-16, 4.000000000000000000 ) ) ;
#47665=CARTESIAN_POINT ( 'NONE',  ( -18.59999999999999787, -10.84999999999999076, 32.89999999999999858 ) ) ;
#47701=VECTOR ( 'NONE', #112031, 1000.000000000000000 ) ;
#47706=ADVANCED_FACE ( 'NONE', ( #44304 ), #80826, .T. ) ;
#47727=FACE_OUTER_BOUND ( 'NONE', #135397, .T. ) ;
#47731=CARTESIAN_POINT ( 'NONE',  ( -18.69999999999999929, -6.162641848847272286, 0.4936627796039583793 ) ) ;
#47746=CARTESIAN_POINT ( 'NONE',  ( -13.40000000000000036, -9.650000000000005684, 17.60000000000000497 ) ) ;
#47804=VECTOR ( 'NONE', #244803, 1000.000000000000114 ) ;
#47829=ORIENTED_EDGE ( 'NONE', *, *, #284, .F. ) ;
#47853=DIRECTION ( 'NONE',  ( 0.000000000000000000, 1.000000000000000000, 0.000000000000000000 ) ) ;
#47888=DIRECTION ( 'NONE',  ( 1.000000000000000000, 0.000000000000000000, 0.000000000000000000 ) ) ;
#47906=CARTESIAN_POINT ( 'NONE',  ( -11.60000000000000320, -8.250000000000005329, 10.95857864376268864 ) ) ;
#47908=DIRECTION ( 'NONE',  ( -1.000000000000000000, 0.000000000000000000, 0.000000000000000000 ) ) ;
#47956=FACE_OUTER_BOUND ( 'NONE', #91205, .T. ) ;
#47977=SURFACE_SIDE_STYLE ('',( #166686 ) ) ;
#47981=VERTEX_POINT ( 'NONE', #158490 ) ;
#47982=EDGE_CURVE ( 'NONE', #171414, #212664, #234136, .T. ) ;
#47983=ORIENTED_EDGE ( 'NONE', *, *, #39965, .F. ) ;
#48015=DIRECTION ( 'NONE',  ( 0.000000000000000000, -0.1686199900910312910, 0.9856811345164826488 ) ) ;
#48020=CARTESIAN_POINT ( 'NONE',  ( -11.60000000000000320, -11.65000000000000036, 15.00000000000000355 ) ) ;
#48021=CARTESIAN_POINT ( 'NONE',  ( 18.79999999999999716, 11.49641995933507843, -1.885425182446133885 ) ) ;
#48027=ADVANCED_FACE ( 'NONE', ( #61935 ), #67071, .F. ) ;
#48050=CIRCLE ( 'NONE', #43769, 0.09999999999999939493 ) ;
#48069=EDGE_LOOP ( 'NONE', ( #81869, #159733, #135842, #212602 ) ) ;
#48072=ORIENTED_EDGE ( 'NONE', *, *, #212472, .T. ) ;
#48103=CARTESIAN_POINT ( 'NONE',  ( 18.79999999999999716, 11.49641995933507843, 1.885425182446133885 ) ) ;
#48115=VECTOR ( 'NONE', #100812, 1000.000000000000000 ) ;
#48119=DIRECTION ( 'NONE',  ( 0.000000000000000000, 0.000000000000000000, 1.000000000000000000 ) ) ;
#48142=EDGE_CURVE ( 'NONE', #255181, #91499, #121917, .T. ) ;
#48158=EDGE_CURVE ( 'NONE', #144252, #150585, #89381, .T. ) ;
#48180=FACE_OUTER_BOUND ( 'NONE', #243054, .T. ) ;
#48183=CARTESIAN_POINT ( 'NONE',  ( 0.8999999999999993561, -11.65000000000000036, 26.00000000000000355 ) ) ;
#48190=EDGE_CURVE ( 'NONE', #219544, #30076, #101841, .T. ) ;
#48243=VERTEX_POINT ( 'NONE', #57760 ) ;
#48257=ORIENTED_EDGE ( 'NONE', *, *, #256543, .T. ) ;
#48326=DIRECTION ( 'NONE',  ( 0.000000000000000000, -0.9868171638914228216, 0.1618390714546044939 ) ) ;
#48394=DIRECTION ( 'NONE',  ( 2.489438768765008884E-17, -0.1686199900910312910, 0.9856811345164826488 ) ) ;
#48402=CARTESIAN_POINT ( 'NONE',  ( -13.40000000000000213, -8.250000000000007105, 15.00000000000000355 ) ) ;
#48429=ORIENTED_EDGE ( 'NONE', *, *, #96181, .T. ) ;
#48434=ORIENTED_EDGE ( 'NONE', *, *, #9530, .T. ) ;
#48437=DIRECTION ( 'NONE',  ( 0.000000000000000000, 0.9910465087640866200, 0.1335171055202867274 ) ) ;
#48446=EDGE_CURVE ( 'NONE', #57698, #91491, #221953, .T. ) ;
#48492=ORIENTED_EDGE ( 'NONE', *, *, #202665, .F. ) ;
#48504=DIRECTION ( 'NONE',  ( 0.000000000000000000, 0.000000000000000000, -1.000000000000000000 ) ) ;
#48509=CIRCLE ( 'NONE', #2711, 0.09999999999999963085 ) ;
#48537=ORIENTED_EDGE ( 'NONE', *, *, #246868, .T. ) ;
#48608=CYLINDRICAL_SURFACE ( 'NONE', #162299, 11.75000000000000000 ) ;
#48662=CARTESIAN_POINT ( 'NONE',  ( -6.000000000000003553, -11.25000000000000000, 10.00000000000000178 ) ) ;
#48734=CARTESIAN_POINT ( 'NONE',  ( -13.40000000000000036, -11.65000000000000036, 17.60000000000000497 ) ) ;
#48786=PLANE ( 'NONE',  #16026 ) ;
#48792=ADVANCED_FACE ( 'NONE', ( #117460 ), #194444, .T. ) ;
#48795=DIRECTION ( 'NONE',  ( -0.000000000000000000, 0.000000000000000000, -1.000000000000000000 ) ) ;
#48817=AXIS2_PLACEMENT_3D ( 'NONE', #147003, #124901, #50458 ) ;
#48837=CIRCLE ( 'NONE', #144696, 0.09999999999999939493 ) ;
#48842=DIRECTION ( 'NONE',  ( 0.000000000000000000, 0.000000000000000000, 1.000000000000000000 ) ) ;
#48863=VERTEX_POINT ( 'NONE', #219100 ) ;
#48867=ADVANCED_FACE ( 'NONE', ( #144700 ), #163015, .T. ) ;
#48915=ORIENTED_EDGE ( 'NONE', *, *, #112688, .T. ) ;
#48927=DIRECTION ( 'NONE',  ( 0.000000000000000000, -1.000000000000000000, 0.000000000000000000 ) ) ;
#48966=DIRECTION ( 'NONE',  ( 0.000000000000000000, 0.000000000000000000, -1.000000000000000000 ) ) ;
#49008=LINE ( 'NONE', #102867, #198844 ) ;
#49010=CARTESIAN_POINT ( 'NONE',  ( -22.94999999999999929, 5.586869315528661062, 16.41686199900910736 ) ) ;
#49014=DIRECTION ( 'NONE',  ( 0.000000000000000000, 0.000000000000000000, 1.000000000000000000 ) ) ;
#49041=CIRCLE ( 'NONE', #232241, 0.09999999999999939493 ) ;
#49045=ORIENTED_EDGE ( 'NONE', *, *, #202432, .F. ) ;
#49052=VERTEX_POINT ( 'NONE', #202945 ) ;
#49057=AXIS2_PLACEMENT_3D ( 'NONE', #187276, #88121, #202963 ) ;
#49076=EDGE_LOOP ( 'NONE', ( #53155, #134455, #156123, #255881 ) ) ;
#49086=FACE_OUTER_BOUND ( 'NONE', #52711, .T. ) ;
#49114=CARTESIAN_POINT ( 'NONE',  ( -5.900000000000003020, -11.34999999999999964, 10.10000000000000142 ) ) ;
#49131=DIRECTION ( 'NONE',  ( 0.000000000000000000, -0.9856811345164800953, -0.1686199900910462790 ) ) ;
#49140=ORIENTED_EDGE ( 'NONE', *, *, #194516, .T. ) ;
#49170=DIRECTION ( 'NONE',  ( 0.000000000000000000, 0.000000000000000000, 1.000000000000000000 ) ) ;
#49182=VECTOR ( 'NONE', #201057, 1000.000000000000000 ) ;
#49188=DIRECTION ( 'NONE',  ( 0.000000000000000000, -0.9868171638914232657, 0.1618390714546023845 ) ) ;
#49199=VECTOR ( 'NONE', #22836, 1000.000000000000000 ) ;
#49202=FACE_OUTER_BOUND ( 'NONE', #38986, .T. ) ;
#49204=DIRECTION ( 'NONE',  ( 1.000000000000000000, 0.000000000000000000, 0.000000000000000000 ) ) ;
#49227=CARTESIAN_POINT ( 'NONE',  ( -20.01715728752537515, 4.611773100472912112, 22.11686199900910665 ) ) ;
#49324=DIRECTION ( 'NONE',  ( 1.000000000000000000, 0.000000000000000000, -0.000000000000000000 ) ) ;
#49343=DIRECTION ( 'NONE',  ( 0.000000000000000000, 0.000000000000000000, 1.000000000000000000 ) ) ;
#49344=CARTESIAN_POINT ( 'NONE',  ( 11.60000000000000320, -11.75000000000000000, 12.30000000000000426 ) ) ;
#49354=EDGE_CURVE ( 'NONE', #83776, #187034, #36275, .T. ) ;
#49400=DIRECTION ( 'NONE',  ( 0.000000000000000000, 0.000000000000000000, 1.000000000000000000 ) ) ;
#49445=ADVANCED_FACE ( 'NONE', ( #163216 ), #143632, .T. ) ;
#49447=EDGE_CURVE ( 'NONE', #194632, #75205, #182784, .T. ) ;
#49449=DIRECTION ( 'NONE',  ( -0.000000000000000000, 1.000000000000000000, -0.000000000000000000 ) ) ;
#49479=ORIENTED_EDGE ( 'NONE', *, *, #102530, .F. ) ;
#49496=ORIENTED_EDGE ( 'NONE', *, *, #114145, .T. ) ;
#49497=EDGE_CURVE ( 'NONE', #166883, #59365, #203612, .T. ) ;
#49504=ORIENTED_EDGE ( 'NONE', *, *, #246068, .T. ) ;
#49507=VERTEX_POINT ( 'NONE', #43263 ) ;
#49524=TOROIDAL_SURFACE ( 'NONE', #82788, 11.65000000000000036, 0.1000000000000000056 ) ;
#49608=ORIENTED_EDGE ( 'NONE', *, *, #86269, .T. ) ;
#49613=FACE_OUTER_BOUND ( 'NONE', #212026, .T. ) ;
#49629=ORIENTED_EDGE ( 'NONE', *, *, #255596, .F. ) ;
#49675=CARTESIAN_POINT ( 'NONE',  ( -18.59999999999999787, 11.75000000000000000, 5.900000000000001243 ) ) ;
#49696=DIRECTION ( 'NONE',  ( 0.000000000000000000, 0.000000000000000000, 1.000000000000000000 ) ) ;
#49717=LINE ( 'NONE', #148833, #45777 ) ;
#49722=FACE_OUTER_BOUND ( 'NONE', #29964, .T. ) ;
#49760=AXIS2_PLACEMENT_3D ( 'NONE', #93171, #73647, #111458 ) ;
#49791=DIRECTION ( 'NONE',  ( 0.000000000000000000, 0.000000000000000000, -1.000000000000000000 ) ) ;
#49823=VERTEX_POINT ( 'NONE', #78215 ) ;
#49825=EDGE_CURVE ( 'NONE', #110943, #108582, #179911, .T. ) ;
#49827=DIRECTION ( 'NONE',  ( 0.000000000000000000, 0.000000000000000000, -1.000000000000000000 ) ) ;
#49830=ORIENTED_EDGE ( 'NONE', *, *, #17995, .T. ) ;
#49877=ORIENTED_EDGE ( 'NONE', *, *, #45763, .T. ) ;
#49925=ORIENTED_EDGE ( 'NONE', *, *, #146996, .F. ) ;
#49933=AXIS2_PLACEMENT_3D ( 'NONE', #1072, #257939, #118501 ) ;
#50001=CARTESIAN_POINT ( 'NONE',  ( 18.79999999999999716, 1.212568896937007645, -7.900000000000000355 ) ) ;
#50018=EDGE_CURVE ( 'NONE', #179078, #224002, #32407, .T. ) ;
#50052=DIRECTION ( 'NONE',  ( 0.000000000000000000, 0.000000000000000000, -1.000000000000000000 ) ) ;
#50058=VECTOR ( 'NONE', #14159, 1000.000000000000000 ) ;
#50114=EDGE_LOOP ( 'NONE', ( #151505, #125442, #105612, #114920 ) ) ;
#50119=EDGE_LOOP ( 'NONE', ( #203781, #18516, #57789, #247404 ) ) ;
#50164=CARTESIAN_POINT ( 'NONE',  ( 18.79999999999999716, 4.513204987021263825, 22.10000000000000142 ) ) ;
#50208=CARTESIAN_POINT ( 'NONE',  ( -11.60000000000000320, -11.65000000000000036, 15.00000000000000355 ) ) ;
#50231=AXIS2_PLACEMENT_3D ( 'NONE', #48020, #150987, #10202 ) ;
#50241=CARTESIAN_POINT ( 'NONE',  ( -19.99999999999999645, 1.350000000000000089, 21.90000000000000213 ) ) ;
#50268=CARTESIAN_POINT ( 'NONE',  ( -5.900000000000003020, -11.34999999999999964, 10.00000000000000178 ) ) ;
#50277=DIRECTION ( 'NONE',  ( 0.000000000000000000, -0.7071067811865479058, 0.7071067811865472397 ) ) ;
#50287=DIRECTION ( 'NONE',  ( 0.000000000000000000, -0.9910465087640866200, -0.1335171055202867274 ) ) ;
#50289=DIRECTION ( 'NONE',  ( -1.000000000000000000, 0.000000000000000000, 0.000000000000000000 ) ) ;
#50296=ORIENTED_EDGE ( 'NONE', *, *, #173239, .F. ) ;
#50348=SPHERICAL_SURFACE ( 'NONE', #223895, 0.1000000000000000056 ) ;
#50376=ORIENTED_EDGE ( 'NONE', *, *, #49447, .F. ) ;
#50386=CIRCLE ( 'NONE', #246055, 0.09999999999999990841 ) ;
#50392=DIRECTION ( 'NONE',  ( 1.000000000000000000, -1.476360405086644309E-16, 0.000000000000000000 ) ) ;
#50433=FACE_OUTER_BOUND ( 'NONE', #187122, .T. ) ;
#50446=VECTOR ( 'NONE', #216039, 1000.000000000000000 ) ;
#50449=EDGE_CURVE ( 'NONE', #140091, #83237, #178912, .T. ) ;
#50458=DIRECTION ( 'NONE',  ( 0.000000000000000000, 0.000000000000000000, -1.000000000000000000 ) ) ;
#50464=VECTOR ( 'NONE', #41488, 1000.000000000000000 ) ;
#50503=VECTOR ( 'NONE', #48015, 1000.000000000000227 ) ;
#50565=LINE ( 'NONE', #11480, #227960 ) ;
#50575=DIRECTION ( 'NONE',  ( -0.000000000000000000, -0.000000000000000000, 1.000000000000000000 ) ) ;
#50580=VECTOR ( 'NONE', #91145, 1000.000000000000114 ) ;
#50585=AXIS2_PLACEMENT_3D ( 'NONE', #154142, #13312, #111118 ) ;
#50608=CARTESIAN_POINT ( 'NONE',  ( -20.99105743725316842, 6.322468215188231433, 12.11686199560448252 ) ) ;
#50632=DIRECTION ( 'NONE',  ( 2.168404344971008868E-16, -0.000000000000000000, 1.000000000000000000 ) ) ;
#50643=DIRECTION ( 'NONE',  ( 0.000000000000000000, 0.1335171055202901413, -0.9910465087640860649 ) ) ;
#50645=CARTESIAN_POINT ( 'NONE',  ( 19.90000000000000568, 1.350000000000000089, 16.50000000000000000 ) ) ;
#50652=ORIENTED_EDGE ( 'NONE', *, *, #66552, .F. ) ;
#50655=EDGE_CURVE ( 'NONE', #219183, #171414, #49717, .T. ) ;
#50768=EDGE_LOOP ( 'NONE', ( #44613, #125713, #18159, #206046 ) ) ;
#50794=ADVANCED_FACE ( 'NONE', ( #254313 ), #8379, .T. ) ;
#50814=ORIENTED_EDGE ( 'NONE', *, *, #50655, .T. ) ;
#50821=DIRECTION ( 'NONE',  ( 1.000000000000000000, -0.000000000000000000, -0.000000000000000000 ) ) ;
#50836=DIRECTION ( 'NONE',  ( 0.000000000000000000, 0.000000000000000000, -1.000000000000000000 ) ) ;
#50846=CARTESIAN_POINT ( 'NONE',  ( -18.79999999999999716, 4.513204987021263825, 22.10000000000000142 ) ) ;
#50961=CIRCLE ( 'NONE', #17645, 0.09999999999999993616 ) ;
#50984=FACE_OUTER_BOUND ( 'NONE', #82598, .T. ) ;
#51011=AXIS2_PLACEMENT_3D ( 'NONE', #43015, #122559, #164252 ) ;
#51032=DIRECTION ( 'NONE',  ( -1.000000000000000000, 0.000000000000000000, 0.000000000000000000 ) ) ;
#51116=EDGE_CURVE ( 'NONE', #169705, #8702, #250181, .T. ) ;
#51130=DIRECTION ( 'NONE',  ( 0.000000000000000000, 0.000000000000000000, 1.000000000000000000 ) ) ;
#51161=DIRECTION ( 'NONE',  ( 0.000000000000000000, 0.000000000000000000, 1.000000000000000000 ) ) ;
#51169=DIRECTION ( 'NONE',  ( -1.000000000000000000, 0.000000000000000000, 0.000000000000000000 ) ) ;
#51283=ORIENTED_EDGE ( 'NONE', *, *, #67311, .T. ) ;
#51351=AXIS2_PLACEMENT_3D ( 'NONE', #85764, #186198, #224019 ) ;
#51359=CARTESIAN_POINT ( 'NONE',  ( -18.79999999999999716, 11.49641995933507843, -1.885425182446133885 ) ) ;
#51416=EDGE_CURVE ( 'NONE', #38945, #137467, #137695, .T. ) ;
#51440=ORIENTED_EDGE ( 'NONE', *, *, #23683, .F. ) ;
#51460=DIRECTION ( 'NONE',  ( 0.000000000000000000, 0.000000000000000000, -1.000000000000000000 ) ) ;
#51464=ORIENTED_EDGE ( 'NONE', *, *, #146012, .T. ) ;
#51496=AXIS2_PLACEMENT_3D ( 'NONE', #126749, #246685, #148893 ) ;
#51509=CARTESIAN_POINT ( 'NONE',  ( -22.94999999999999929, 0.000000000000000000, 0.000000000000000000 ) ) ;
#51542=DIRECTION ( 'NONE',  ( 0.000000000000000000, -1.000000000000000000, 0.000000000000000000 ) ) ;
#51547=ORIENTED_EDGE ( 'NONE', *, *, #250668, .F. ) ;
#51566=EDGE_CURVE ( 'NONE', #122006, #145044, #225182, .T. ) ;
#51610=CARTESIAN_POINT ( 'NONE',  ( 18.79999999999999716, 1.350000000000000089, 21.90000000000000213 ) ) ;
#51642=DIRECTION ( 'NONE',  ( -1.000000000000000000, 0.000000000000000000, 0.000000000000000000 ) ) ;
#51689=VERTEX_POINT ( 'NONE', #89197 ) ;
#51715=DIRECTION ( 'NONE',  ( 1.000000000000000000, 0.000000000000000000, 0.000000000000000000 ) ) ;
#51741=VECTOR ( 'NONE', #254350, 1000.000000000000000 ) ;
#51780=ORIENTED_EDGE ( 'NONE', *, *, #138812, .T. ) ;
#51888=AXIS2_PLACEMENT_3D ( 'NONE', #116087, #193055, #213887 ) ;
#51897=CIRCLE ( 'NONE', #256430, 0.09999999999999939493 ) ;
#51939=CIRCLE ( 'NONE', #110212, 0.09999999999999982514 ) ;
#51980=CARTESIAN_POINT ( 'NONE',  ( -18.59999999999999787, -9.849999999999994316, 30.09999999999999787 ) ) ;
#51981=ORIENTED_EDGE ( 'NONE', *, *, #200806, .T. ) ;
#51992=CARTESIAN_POINT ( 'NONE',  ( -20.90000000000000213, -1.212568896937008089, -8.000000000000000000 ) ) ;
#52041=DIRECTION ( 'NONE',  ( 1.000000000000000000, -0.000000000000000000, -0.000000000000000000 ) ) ;
#52094=ORIENTED_EDGE ( 'NONE', *, *, #98439, .T. ) ;
#52119=EDGE_CURVE ( 'NONE', #163484, #89234, #102715, .T. ) ;
#52126=LINE ( 'NONE', #67849, #78017 ) ;
#52129=DIRECTION ( 'NONE',  ( 1.000000000000000000, 0.000000000000000000, 0.000000000000000000 ) ) ;
#52210=DIRECTION ( 'NONE',  ( 0.000000000000000000, 0.1335171055202867274, -0.9910465087640866200 ) ) ;
#52219=ORIENTED_EDGE ( 'NONE', *, *, #11538, .F. ) ;
#52256=CARTESIAN_POINT ( 'NONE',  ( -18.79999999999999716, 1.350000000000000089, 21.90000000000000213 ) ) ;
#52261=DIRECTION ( 'NONE',  ( 0.000000000000000000, 0.000000000000000000, 1.000000000000000000 ) ) ;
#52264=DIRECTION ( 'NONE',  ( 0.000000000000000000, 0.000000000000000000, 1.000000000000000000 ) ) ;
#52314=DIRECTION ( 'NONE',  ( 0.000000000000000000, 0.000000000000000000, 1.000000000000000000 ) ) ;
#52347=CYLINDRICAL_SURFACE ( 'NONE', #168788, 0.09999999999999939493 ) ;
#52362=CARTESIAN_POINT ( 'NONE',  ( -5.900000000000002132, -11.34999999999999964, 13.90000000000000213 ) ) ;
#52373=AXIS2_PLACEMENT_3D ( 'NONE', #140904, #121375, #117486 ) ;
#52491=EDGE_LOOP ( 'NONE', ( #30861, #95898, #69931, #83189 ) ) ;
#52505=ORIENTED_EDGE ( 'NONE', *, *, #144570, .F. ) ;
#52572=EDGE_CURVE ( 'NONE', #99532, #175526, #13390, .T. ) ;
#52590=PLANE ( 'NONE',  #110600 ) ;
#52614=VECTOR ( 'NONE', #219893, 1000.000000000000000 ) ;
#52635=CARTESIAN_POINT ( 'NONE',  ( -5.900000000000002132, -11.75000000000000000, 14.10000000000000142 ) ) ;
#52694=FACE_OUTER_BOUND ( 'NONE', #250480, .T. ) ;
#52696=CARTESIAN_POINT ( 'NONE',  ( -20.90000000000000213, 1.786320531569725478, -11.50977166988710820 ) ) ;
#52711=EDGE_LOOP ( 'NONE', ( #48072, #76761, #247853, #257726 ) ) ;
#52713=CARTESIAN_POINT ( 'NONE',  ( 22.10000000000000497, 3.362550747017869490, 28.82623795144604983 ) ) ;
#52726=LINE ( 'NONE', #214380, #184563 ) ;
#52733=CARTESIAN_POINT ( 'NONE',  ( 0.8999999999999993561, -11.65000000000000036, 23.40000000000000568 ) ) ;
#52735=CARTESIAN_POINT ( 'NONE',  ( -13.40000000000000036, -12.25000000000000178, 15.00000000000000355 ) ) ;
#52764=LINE ( 'NONE', #193583, #241175 ) ;
#52766=VERTEX_POINT ( 'NONE', #17788 ) ;
#52778=VECTOR ( 'NONE', #66926, 1000.000000000000000 ) ;
#52789=EDGE_CURVE ( 'NONE', #163445, #136731, #238411, .T. ) ;
#52792=EDGE_CURVE ( 'NONE', #203870, #186764, #157354, .T. ) ;
#52812=ORIENTED_EDGE ( 'NONE', *, *, #111758, .T. ) ;
#52816=ORIENTED_EDGE ( 'NONE', *, *, #132501, .F. ) ;
#52853=LINE ( 'NONE', #49010, #159603 ) ;
#52930=ORIENTED_EDGE ( 'NONE', *, *, #83535, .F. ) ;
#52966=EDGE_LOOP ( 'NONE', ( #250376, #257513, #32523, #69586 ) ) ;
#53003=DIRECTION ( 'NONE',  ( 0.000000000000000000, -0.9856811345164829818, -0.1686199900910294314 ) ) ;
#53013=CARTESIAN_POINT ( 'NONE',  ( -21.00000000000000000, -0.3305886640091971196, 0.04453801223857078301 ) ) ;
#53016=ORIENTED_EDGE ( 'NONE', *, *, #95700, .T. ) ;
#53020=EDGE_CURVE ( 'NONE', #106580, #70167, #146261, .T. ) ;
#53022=CARTESIAN_POINT ( 'NONE',  ( -22.19999999999999929, -11.75000000000000000, 14.10000000000000142 ) ) ;
#53032=ORIENTED_EDGE ( 'NONE', *, *, #13795, .T. ) ;
#53059=EDGE_LOOP ( 'NONE', ( #82953, #82902, #179179, #83300 ) ) ;
#53060=CIRCLE ( 'NONE', #240513, 0.09999999999999939493 ) ;
#53090=DIRECTION ( 'NONE',  ( 0.000000000000000000, 0.000000000000000000, -1.000000000000000000 ) ) ;
#53095=CYLINDRICAL_SURFACE ( 'NONE', #134845, 0.09999999999999997780 ) ;
#53109=DIRECTION ( 'NONE',  ( 1.000000000000000000, -0.000000000000000000, -0.000000000000000000 ) ) ;
#53141=AXIS2_PLACEMENT_3D ( 'NONE', #18910, #137559, #219675 ) ;
#53145=CIRCLE ( 'NONE', #57212, 0.09999999999999990841 ) ;
#53155=ORIENTED_EDGE ( 'NONE', *, *, #83660, .F. ) ;
#53174=CARTESIAN_POINT ( 'NONE',  ( 20.90000000000000213, 1.885425182446133885, -11.49641995933507843 ) ) ;
#53209=ADVANCED_FACE ( 'NONE', ( #154482 ), #214408, .T. ) ;
#53274=EDGE_LOOP ( 'NONE', ( #198089, #78044, #32400, #190722 ) ) ;
#53282=CARTESIAN_POINT ( 'NONE',  ( 18.59999999999999787, -10.84999999999999076, -15.00000000000000000 ) ) ;
#53312=VERTEX_POINT ( 'NONE', #239121 ) ;
#53355=DIRECTION ( 'NONE',  ( 0.000000000000000000, 0.000000000000000000, 1.000000000000000000 ) ) ;
#53368=DIRECTION ( 'NONE',  ( 0.000000000000000000, -1.000000000000000000, 0.000000000000000000 ) ) ;
#53386=DIRECTION ( 'NONE',  ( 0.000000000000000000, -0.000000000000000000, 1.000000000000000000 ) ) ;
#53405=ORIENTED_EDGE ( 'NONE', *, *, #25343, .T. ) ;
#53410=ORIENTED_EDGE ( 'NONE', *, *, #49447, .T. ) ;
#53430=DIRECTION ( 'NONE',  ( 0.000000000000000000, 0.000000000000000000, -1.000000000000000000 ) ) ;
#53549=EDGE_CURVE ( 'NONE', #192176, #120569, #113312, .T. ) ;
#53554=AXIS2_PLACEMENT_3D ( 'NONE', #186797, #207646, #45979 ) ;
#53560=ADVANCED_FACE ( 'NONE', ( #179826 ), #129862, .T. ) ;
#53654=CIRCLE ( 'NONE', #120341, 0.09999999999999939493 ) ;
#53681=EDGE_LOOP ( 'NONE', ( #18967, #113384, #27572, #45929 ) ) ;
#53730=VECTOR ( 'NONE', #5331, 1000.000000000000000 ) ;
#53742=ORIENTED_EDGE ( 'NONE', *, *, #144632, .T. ) ;
#53752=DIRECTION ( 'NONE',  ( 1.000000000000000000, -0.000000000000000000, -0.000000000000000000 ) ) ;
#53754=ORIENTED_EDGE ( 'NONE', *, *, #45722, .F. ) ;
#53774=DIRECTION ( 'NONE',  ( 1.000000000000000000, 0.000000000000000000, 0.000000000000000000 ) ) ;
#53803=CARTESIAN_POINT ( 'NONE',  ( -18.69999999999999929, -8.250000000000005329, 22.10000000000000142 ) ) ;
#53877=CARTESIAN_POINT ( 'NONE',  ( -13.40000000000000213, -11.65000000000000036, 15.00000000000000355 ) ) ;
#53910=ORIENTED_EDGE ( 'NONE', *, *, #100042, .F. ) ;
#53913=EDGE_LOOP ( 'NONE', ( #215632, #220479, #205592, #28792 ) ) ;
#53924=EDGE_LOOP ( 'NONE', ( #247509, #191959, #180193 ) ) ;
#53935=DIRECTION ( 'NONE',  ( -1.000000000000000000, 0.000000000000000000, 0.000000000000000000 ) ) ;
#53979=ADVANCED_FACE ( 'NONE', ( #15309 ), #239478, .T. ) ;
#53990=ORIENTED_EDGE ( 'NONE', *, *, #244008, .T. ) ;
#54002=CARTESIAN_POINT ( 'NONE',  ( 11.60000000000000142, -11.65000000000000036, 12.40000000000000391 ) ) ;
#54051=ORIENTED_EDGE ( 'NONE', *, *, #155840, .T. ) ;
#54058=CARTESIAN_POINT ( 'NONE',  ( -18.69999999999999929, 6.644425182197218227, 9.641788261573355001 ) ) ;
#54065=CIRCLE ( 'NONE', #199852, 2.700000000000001066 ) ;
#54077=EDGE_CURVE ( 'NONE', #141361, #59365, #75904, .T. ) ;
#54087=ORIENTED_EDGE ( 'NONE', *, *, #11570, .T. ) ;
#54133=CARTESIAN_POINT ( 'NONE',  ( 13.40000000000000036, -12.24999999999999822, 15.00000000000000355 ) ) ;
#54156=AXIS2_PLACEMENT_3D ( 'NONE', #232131, #252946, #233420 ) ;
#54313=TOROIDAL_SURFACE ( 'NONE', #149, 0.2000000000000000111, 0.1000000000000000056 ) ;
#54322=DIRECTION ( 'NONE',  ( 0.000000000000000000, 0.000000000000000000, 1.000000000000000000 ) ) ;
#54333=CIRCLE ( 'NONE', #145920, 11.65000000000000036 ) ;
#54356=ORIENTED_EDGE ( 'NONE', *, *, #17995, .F. ) ;
#54374=FACE_OUTER_BOUND ( 'NONE', #169369, .T. ) ;
#54403=VECTOR ( 'NONE', #110516, 1000.000000000000000 ) ;
#54404=ORIENTED_EDGE ( 'NONE', *, *, #94616, .T. ) ;
#54456=CARTESIAN_POINT ( 'NONE',  ( 11.60000000000000320, -8.250000000000003553, 17.60000000000000497 ) ) ;
#54464=CARTESIAN_POINT ( 'NONE',  ( -20.90000000000000213, 3.461118860469513336, 28.84309995045515507 ) ) ;
#54537=DIRECTION ( 'NONE',  ( 0.000000000000000000, 0.1618390714546044939, -0.9868171638914228216 ) ) ;
#54543=ORIENTED_EDGE ( 'NONE', *, *, #158899, .F. ) ;
#54556=DIRECTION ( 'NONE',  ( 0.000000000000000000, 0.000000000000000000, -1.000000000000000000 ) ) ;
#54557=DIRECTION ( 'NONE',  ( 0.000000000000000000, -0.9910465087640865089, 0.1335171055202864221 ) ) ;
#54590=AXIS2_PLACEMENT_3D ( 'NONE', #125878, #146708, #103726 ) ;
#54607=EDGE_LOOP ( 'NONE', ( #139859, #121088, #248205, #75962 ) ) ;
#54610=CYLINDRICAL_SURFACE ( 'NONE', #138937, 0.09999999999999933942 ) ;
#54622=CARTESIAN_POINT ( 'NONE',  ( -20.90000000000000213, 8.000000000000000000, 1.212568896937007867 ) ) ;
#54694=DIRECTION ( 'NONE',  ( 0.000000000000000000, 1.000000000000000000, 0.000000000000000000 ) ) ;
#54695=FACE_OUTER_BOUND ( 'NONE', #225354, .T. ) ;
#54741=DIRECTION ( 'NONE',  ( 0.000000000000000000, 0.000000000000000000, -1.000000000000000000 ) ) ;
#54753=LINE ( 'NONE', #173488, #98924 ) ;
#54757=CIRCLE ( 'NONE', #137942, 0.2000000000000000944 ) ;
#54814=ADVANCED_FACE ( 'NONE', ( #45786 ), #24968, .T. ) ;
#54846=CARTESIAN_POINT ( 'NONE',  ( 21.10000000000000142, -1.720267447010333833E-15, 11.89999999999999858 ) ) ;
#54897=EDGE_CURVE ( 'NONE', #225036, #178041, #241433, .T. ) ;
#54899=DIRECTION ( 'NONE',  ( 1.000000000000000000, -0.000000000000000000, -0.000000000000000000 ) ) ;
#54966=AXIS2_PLACEMENT_3D ( 'NONE', #169430, #132842, #211085 ) ;
#54973=EDGE_CURVE ( 'NONE', #7521, #228920, #206151, .T. ) ;
#55019=AXIS2_PLACEMENT_3D ( 'NONE', #109299, #49343, #83304 ) ;
#55030=DIRECTION ( 'NONE',  ( 0.000000000000000000, 0.000000000000000000, 1.000000000000000000 ) ) ;
#55083=SPHERICAL_SURFACE ( 'NONE', #245272, 0.1000000000000000056 ) ;
#55089=ORIENTED_EDGE ( 'NONE', *, *, #198288, .T. ) ;
#55090=CARTESIAN_POINT ( 'NONE',  ( -18.79999999999999716, -1.410778198689824459, -7.973296578895943121 ) ) ;
#55098=ADVANCED_FACE ( 'NONE', ( #148757 ), #207448, .T. ) ;
#55145=VECTOR ( 'NONE', #99655, 1000.000000000000000 ) ;
#55165=EDGE_LOOP ( 'NONE', ( #197754, #136135, #180766, #81599 ) ) ;
#55170=VECTOR ( 'NONE', #17463, 1000.000000000000000 ) ;
#55217=EDGE_LOOP ( 'NONE', ( #242125, #187996, #28993, #136710, #218626, #90414, #128687, #77529, #129944, #124350, #65399, #158211, #77296, #147073, #139527, #68495, #234985 ) ) ;
#55220=ORIENTED_EDGE ( 'NONE', *, *, #142002, .F. ) ;
#55227=FACE_OUTER_BOUND ( 'NONE', #9860, .T. ) ;
#55279=DIRECTION ( 'NONE',  ( -0.000000000000000000, -0.9910465087640860649, 0.1335171055202901413 ) ) ;
#55288=ORIENTED_EDGE ( 'NONE', *, *, #158884, .T. ) ;
#55291=CARTESIAN_POINT ( 'NONE',  ( -18.59999999999999787, -10.72142460728770352, 6.051435706882140053 ) ) ;
#55320=EDGE_CURVE ( 'NONE', #183834, #190169, #166757, .T. ) ;
#55335=ORIENTED_EDGE ( 'NONE', *, *, #56704, .F. ) ;
#55398=CARTESIAN_POINT ( 'NONE',  ( -21.00000000000000000, 8.058024882095860875, 1.378482379536266178 ) ) ;
#55440=CARTESIAN_POINT ( 'NONE',  ( -22.19999999999999929, -1.467286812112899463, 28.00000000000000000 ) ) ;
#55453=ORIENTED_EDGE ( 'NONE', *, *, #123908, .F. ) ;
#55455=DIRECTION ( 'NONE',  ( 1.000000000000000000, 0.000000000000000000, 0.000000000000000000 ) ) ;
#55468=EDGE_LOOP ( 'NONE', ( #196746, #103837, #218496, #37001 ) ) ;
#55495=FACE_OUTER_BOUND ( 'NONE', #228659, .T. ) ;
#55504=CARTESIAN_POINT ( 'NONE',  ( 18.59999999999999787, -10.80884033489985363, 6.100000000000002309 ) ) ;
#55515=CARTESIAN_POINT ( 'NONE',  ( -13.40000000000000213, -8.250000000000005329, 15.00000000000000355 ) ) ;
#55545=ORIENTED_EDGE ( 'NONE', *, *, #8418, .F. ) ;
#55573=DIRECTION ( 'NONE',  ( -1.000000000000000000, 0.000000000000000000, -0.000000000000000000 ) ) ;
#55651=ORIENTED_EDGE ( 'NONE', *, *, #26721, .F. ) ;
#55686=ORIENTED_EDGE ( 'NONE', *, *, #165111, .T. ) ;
#55728=ORIENTED_EDGE ( 'NONE', *, *, #147704, .T. ) ;
#55767=DIRECTION ( 'NONE',  ( -0.000000000000000000, 1.000000000000000000, -0.000000000000000000 ) ) ;
#55862=VERTEX_POINT ( 'NONE', #215480 ) ;
#55868=LINE ( 'NONE', #135424, #221722 ) ;
#55881=ORIENTED_EDGE ( 'NONE', *, *, #75902, .T. ) ;
#55897=CIRCLE ( 'NONE', #160009, 0.09999999999999939493 ) ;
#55957=DIRECTION ( 'NONE',  ( 1.000000000000000000, 0.000000000000000000, 0.000000000000000000 ) ) ;
#55959=CARTESIAN_POINT ( 'NONE',  ( 18.59999999999999787, -8.250000000000005329, 32.89999999999999858 ) ) ;
#55974=CARTESIAN_POINT ( 'NONE',  ( 0.8999999999999993561, -8.250000000000005329, 26.00000000000000355 ) ) ;
#55979=DIRECTION ( 'NONE',  ( 6.938893903907270030E-14, -0.000000000000000000, 1.000000000000000000 ) ) ;
#56051=CARTESIAN_POINT ( 'NONE',  ( -19.89999999999999858, 1.350000000000000089, 16.60000000000000142 ) ) ;
#56072=FACE_OUTER_BOUND ( 'NONE', #179011, .T. ) ;
#56128=EDGE_CURVE ( 'NONE', #69570, #147074, #70568, .T. ) ;
#56146=ORIENTED_EDGE ( 'NONE', *, *, #70681, .T. ) ;
#56148=CARTESIAN_POINT ( 'NONE',  ( -19.99999999999999645, 5.454087299794355914, 16.60000000000000142 ) ) ;
#56172=DIRECTION ( 'NONE',  ( 0.000000000000000000, 0.000000000000000000, -1.000000000000000000 ) ) ;
#56203=ORIENTED_EDGE ( 'NONE', *, *, #177266, .T. ) ;
#56204=VERTEX_POINT ( 'NONE', #133083 ) ;
#56230=EDGE_LOOP ( 'NONE', ( #210652, #100362, #216049, #197680 ) ) ;
#56319=ORIENTED_EDGE ( 'NONE', *, *, #39965, .T. ) ;
#56344=ORIENTED_EDGE ( 'NONE', *, *, #197187, .F. ) ;
#56384=CIRCLE ( 'NONE', #89714, 0.09999999999999939493 ) ;
#56391=FACE_OUTER_BOUND ( 'NONE', #18143, .T. ) ;
#56435=ADVANCED_FACE ( 'NONE', ( #52694 ), #31255, .T. ) ;
#56458=EDGE_CURVE ( 'NONE', #189583, #144252, #251961, .T. ) ;
#56465=VECTOR ( 'NONE', #197625, 1000.000000000000000 ) ;
#56490=DIRECTION ( 'NONE',  ( 0.000000000000000000, 0.000000000000000000, -1.000000000000000000 ) ) ;
#56509=ORIENTED_EDGE ( 'NONE', *, *, #226988, .T. ) ;
#56511=ORIENTED_EDGE ( 'NONE', *, *, #73226, .T. ) ;
#56541=VERTEX_POINT ( 'NONE', #77389 ) ;
#56565=DIRECTION ( 'NONE',  ( 0.000000000000000000, 1.000000000000000000, 0.000000000000000000 ) ) ;
#56607=EDGE_LOOP ( 'NONE', ( #18734, #52930, #107882, #191933 ) ) ;
#56643=ORIENTED_EDGE ( 'NONE', *, *, #240221, .T. ) ;
#56693=LINE ( 'NONE', #215786, #967 ) ;
#56704=EDGE_CURVE ( 'NONE', #99187, #169705, #227201, .T. ) ;
#56708=DIRECTION ( 'NONE',  ( 0.000000000000000000, 0.000000000000000000, -1.000000000000000000 ) ) ;
#56724=CARTESIAN_POINT ( 'NONE',  ( -22.20000000000000284, 11.75000000000000000, 32.89999999999999858 ) ) ;
#56725=DIRECTION ( 'NONE',  ( -1.000000000000000000, 0.000000000000000000, 0.000000000000000000 ) ) ;
#56732=CIRCLE ( 'NONE', #81856, 0.09999999999999918676 ) ;
#56764=CARTESIAN_POINT ( 'NONE',  ( 18.59999999999999787, -11.75000000000000000, 5.900000000000001243 ) ) ;
#56767=CARTESIAN_POINT ( 'NONE',  ( -22.94999999999999929, -1.212568896937008089, -8.000000000000000000 ) ) ;
#56769=ORIENTED_EDGE ( 'NONE', *, *, #158034, .F. ) ;
#56829=DIRECTION ( 'NONE',  ( 1.000000000000000000, 0.000000000000000000, 0.000000000000000000 ) ) ;
#56859=EDGE_CURVE ( 'NONE', #118769, #28763, #177170, .T. ) ;
#56873=DIRECTION ( 'NONE',  ( -0.000000000000000000, -0.1618390714546045217, 0.9868171638914230437 ) ) ;
#56880=CARTESIAN_POINT ( 'NONE',  ( -13.40000000000000213, -8.250000000000005329, 10.95857864376269042 ) ) ;
#56890=ORIENTED_EDGE ( 'NONE', *, *, #38774, .T. ) ;
#56905=AXIS2_PLACEMENT_3D ( 'NONE', #99326, #81051, #216727 ) ;
#56909=ADVANCED_FACE ( 'NONE', ( #61054 ), #80597, .T. ) ;
#56920=DIRECTION ( 'NONE',  ( 1.000000000000000000, 0.000000000000000000, 0.000000000000000000 ) ) ;
#56931=CARTESIAN_POINT ( 'NONE',  ( 18.79999999999999716, 5.586869315528661062, 16.41686199900910736 ) ) ;
#56937=EDGE_LOOP ( 'NONE', ( #145202, #179397 ) ) ;
#57038=DIRECTION ( 'NONE',  ( 0.000000000000000000, -0.1335171055202901691, 0.9910465087640861759 ) ) ;
#57042=CARTESIAN_POINT ( 'NONE',  ( 18.79999999999999716, 11.49641995933507843, 1.885425182446133441 ) ) ;
#57056=DIRECTION ( 'NONE',  ( -0.000000000000000000, 1.000000000000000000, 1.445602896647339410E-16 ) ) ;
#57066=AXIS2_PLACEMENT_3D ( 'NONE', #177665, #18565, #257114 ) ;
#57087=VERTEX_POINT ( 'NONE', #29670 ) ;
#57101=CARTESIAN_POINT ( 'NONE',  ( -18.79999999999999716, -2.462484827400500453, -15.77971343137458682 ) ) ;
#57131=ORIENTED_EDGE ( 'NONE', *, *, #225381, .F. ) ;
#57163=DIRECTION ( 'NONE',  ( 0.000000000000000000, 0.000000000000000000, 1.000000000000000000 ) ) ;
#57164=VECTOR ( 'NONE', #168302, 1000.000000000000000 ) ;
#57174=FACE_OUTER_BOUND ( 'NONE', #34433, .T. ) ;
#57212=AXIS2_PLACEMENT_3D ( 'NONE', #18617, #28935, #48437 ) ;
#57213=EDGE_LOOP ( 'NONE', ( #236800, #194544, #49479, #117201 ) ) ;
#57240=VECTOR ( 'NONE', #93885, 1000.000000000000000 ) ;
#57247=VERTEX_POINT ( 'NONE', #174336 ) ;
#57258=CARTESIAN_POINT ( 'NONE',  ( -19.89999999999999858, 4.513204987021263825, 22.00000000000000355 ) ) ;
#57261=ORIENTED_EDGE ( 'NONE', *, *, #147704, .F. ) ;
#57290=EDGE_CURVE ( 'NONE', #168032, #187034, #119252, .T. ) ;
#57306=CARTESIAN_POINT ( 'NONE',  ( 18.69999999999999929, 1.250000000000000000, 16.60000000000000142 ) ) ;
#57345=AXIS2_PLACEMENT_3D ( 'NONE', #138678, #171785, #150901 ) ;
#57349=ORIENTED_EDGE ( 'NONE', *, *, #145479, .T. ) ;
#57379=CIRCLE ( 'NONE', #203130, 0.09999999999999990841 ) ;
#57405=EDGE_LOOP ( 'NONE', ( #181267, #115335, #209461, #70136 ) ) ;
#57408=EDGE_LOOP ( 'NONE', ( #249292, #201026, #218870, #246694, #13302, #213857, #45734, #74082, #224916, #179729, #57349, #223633, #124118, #36085, #69944, #90191, #9122, #115714, #178445, #236465, #209402, #74686, #40595, #238656, #78378, #136754, #230305, #24226, #137248 ) ) ;
#57474=ORIENTED_EDGE ( 'NONE', *, *, #113779, .F. ) ;
#57500=ORIENTED_EDGE ( 'NONE', *, *, #182195, .F. ) ;
#57534=ORIENTED_EDGE ( 'NONE', *, *, #46193, .F. ) ;
#57542=CIRCLE ( 'NONE', #20157, 0.1000000000000002554 ) ;
#57590=ADVANCED_FACE ( 'NONE', ( #134821 ), #170178, .F. ) ;
#57613=AXIS2_PLACEMENT_3D ( 'NONE', #104497, #158132, #202344 ) ;
#57618=ADVANCED_FACE ( 'NONE', ( #253502 ), #12364, .T. ) ;
#57669=ADVANCED_FACE ( 'NONE', ( #16216 ), #149305, .T. ) ;
#57698=VERTEX_POINT ( 'NONE', #137406 ) ;
#57729=DIRECTION ( 'NONE',  ( 0.000000000000000000, 0.000000000000000000, -1.000000000000000000 ) ) ;
#57732=EDGE_LOOP ( 'NONE', ( #111295, #135680, #243451, #19735 ) ) ;
#57736=EDGE_CURVE ( 'NONE', #212150, #182680, #81268, .T. ) ;
#57737=AXIS2_PLACEMENT_3D ( 'NONE', #66762, #143715, #25089 ) ;
#57752=CYLINDRICAL_SURFACE ( 'NONE', #171952, 0.1000000000000028644 ) ;
#57760=CARTESIAN_POINT ( 'NONE',  ( -18.79999999999999716, 5.488301202077012775, 16.50000000000000000 ) ) ;
#57766=CARTESIAN_POINT ( 'NONE',  ( 21.00000000000000000, -1.885425182446133885, -11.49641995933507843 ) ) ;
#57789=ORIENTED_EDGE ( 'NONE', *, *, #75902, .F. ) ;
#57800=CARTESIAN_POINT ( 'NONE',  ( -0.8999999999999993561, -9.650000000000003908, 28.60000000000000142 ) ) ;
#57815=CARTESIAN_POINT ( 'NONE',  ( 20.90000000000000213, 6.356682116888462630, 11.91686199900910381 ) ) ;
#57816=DIRECTION ( 'NONE',  ( 0.000000000000000000, 0.000000000000000000, -1.000000000000000000 ) ) ;
#57829=EDGE_LOOP ( 'NONE', ( #75891, #20434, #253818, #11311 ) ) ;
#57842=CARTESIAN_POINT ( 'NONE',  ( 18.69999999999999929, -10.74999999999999289, 32.89999999999999858 ) ) ;
#57851=AXIS2_PLACEMENT_3D ( 'NONE', #27929, #106122, #68314 ) ;
#57907=CIRCLE ( 'NONE', #212067, 0.2000000000000005107 ) ;
#57924=AXIS2_PLACEMENT_3D ( 'NONE', #227318, #186943, #108659 ) ;
#57933=SPHERICAL_SURFACE ( 'NONE', #86931, 0.1000000000000000056 ) ;
#57963=EDGE_CURVE ( 'NONE', #51689, #20074, #91575, .T. ) ;
#58008=ORIENTED_EDGE ( 'NONE', *, *, #16433, .F. ) ;
#58029=CONICAL_SURFACE ( 'NONE', #32983, 4.000000000000000000, 0.7853981633974489451 ) ;
#58032=DIRECTION ( 'NONE',  ( 1.000000000000000000, 0.000000000000000000, 0.000000000000000000 ) ) ;
#58108=CARTESIAN_POINT ( 'NONE',  ( 20.90000000000000213, 7.900000000000000355, 1.212568896937007867 ) ) ;
#58121=LINE ( 'NONE', #709, #207782 ) ;
#58182=CYLINDRICAL_SURFACE ( 'NONE', #186603, 0.09999999999999939493 ) ;
#58216=CARTESIAN_POINT ( 'NONE',  ( 22.10000000000000497, -11.75000000000000000, -15.00000000000000000 ) ) ;
#58219=ORIENTED_EDGE ( 'NONE', *, *, #80637, .T. ) ;
#58235=CARTESIAN_POINT ( 'NONE',  ( -21.10000000000000142, 6.223900101154156594, 12.00000000000000000 ) ) ;
#58261=VERTEX_POINT ( 'NONE', #202235 ) ;
#58269=ORIENTED_EDGE ( 'NONE', *, *, #202572, .F. ) ;
#58294=CIRCLE ( 'NONE', #49933, 0.09999999999999939493 ) ;
#58306=CARTESIAN_POINT ( 'NONE',  ( 22.19999999999999929, -11.75000000000000000, 32.89999999999999858 ) ) ;
#58318=CARTESIAN_POINT ( 'NONE',  ( -13.40000000000000213, -9.650000000000005684, 15.00000000000000355 ) ) ;
#58331=AXIS2_PLACEMENT_3D ( 'NONE', #63341, #183312, #184582 ) ;
#58332=CYLINDRICAL_SURFACE ( 'NONE', #68950, 0.09999999999999939493 ) ;
#58340=DIRECTION ( 'NONE',  ( 0.000000000000000000, 0.000000000000000000, 1.000000000000000000 ) ) ;
#58392=EDGE_CURVE ( 'NONE', #83237, #63710, #76499, .T. ) ;
#58416=CIRCLE ( 'NONE', #204166, 0.09999999999999963085 ) ;
#58433=ORIENTED_EDGE ( 'NONE', *, *, #215935, .T. ) ;
#58443=DIRECTION ( 'NONE',  ( 0.000000000000000000, 0.000000000000000000, 1.000000000000000000 ) ) ;
#58489=( BOUNDED_CURVE ( )  B_SPLINE_CURVE ( 3, ( #161215, #77799, #196472, #58235 ),
 .UNSPECIFIED., .F., .F. ) 
 B_SPLINE_CURVE_WITH_KNOTS ( ( 4, 4 ),
 ( 4.712388980384687009, 6.283185307179586232 ),
 .UNSPECIFIED. ) 
 CURVE ( )  GEOMETRIC_REPRESENTATION_ITEM ( )  RATIONAL_B_SPLINE_CURVE ( ( 1.000000000000000000, 0.8047378541243643824, 0.8047378541243643824, 1.000000000000000000 ) ) 
 REPRESENTATION_ITEM ( '' )  );
#58498=EDGE_CURVE ( 'NONE', #154676, #130397, #157369, .T. ) ;
#58533=DIRECTION ( 'NONE',  ( 0.000000000000000000, 0.000000000000000000, -1.000000000000000000 ) ) ;
#58544=LINE ( 'NONE', #138084, #99389 ) ;
#58584=DIRECTION ( 'NONE',  ( -1.000000000000000000, 0.000000000000000000, 0.000000000000000000 ) ) ;
#58628=ORIENTED_EDGE ( 'NONE', *, *, #205032, .F. ) ;
#58667=CIRCLE ( 'NONE', #204419, 0.1000000000000000472 ) ;
#58688=VERTEX_POINT ( 'NONE', #111480 ) ;
#58691=DIRECTION ( 'NONE',  ( -0.000000000000000000, 1.000000000000000000, 1.445602896647339410E-16 ) ) ;
#58695=LINE ( 'NONE', #255584, #21399 ) ;
#58768=CARTESIAN_POINT ( 'NONE',  ( -21.10000000000000142, 6.322468214605804882, 12.11686199900910310 ) ) ;
#58776=ORIENTED_EDGE ( 'NONE', *, *, #237264, .T. ) ;
#58801=DIRECTION ( 'NONE',  ( 1.000000000000000000, 0.000000000000000000, 0.000000000000000000 ) ) ;
#58803=ORIENTED_EDGE ( 'NONE', *, *, #189526, .T. ) ;
#58865=EDGE_CURVE ( 'NONE', #211037, #76531, #94449, .T. ) ;
#58878=CYLINDRICAL_SURFACE ( 'NONE', #136056, 0.09999999999999939493 ) ;
#58910=CARTESIAN_POINT ( 'NONE',  ( 18.59999999999999787, -10.80884033489985363, 6.100000000000002309 ) ) ;
#58911=CARTESIAN_POINT ( 'NONE',  ( -20.00889983613310008, 5.561941060815491333, 16.56258203121810268 ) ) ;
#58948=AXIS2_PLACEMENT_3D ( 'NONE', #167718, #149431, #50287 ) ;
#58952=CARTESIAN_POINT ( 'NONE',  ( -22.94999999999999929, 11.50977166988710820, 1.786320531569725478 ) ) ;
#59007=DIRECTION ( 'NONE',  ( 0.000000000000000000, 0.1335171055202867274, -0.9910465087640866200 ) ) ;
#59036=TOROIDAL_SURFACE ( 'NONE', #175604, 0.2000000000000000111, 0.1000000000000000056 ) ;
#59092=CIRCLE ( 'NONE', #34222, 0.09999999999999939493 ) ;
#59125=LINE ( 'NONE', #179142, #39277 ) ;
#59131=CARTESIAN_POINT ( 'NONE',  ( 21.00000000000000000, 1.212568896937007645, -8.000000000000000000 ) ) ;
#59149=EDGE_CURVE ( 'NONE', #28188, #27371, #54333, .T. ) ;
#59154=DIRECTION ( 'NONE',  ( -0.000000000000000000, 0.000000000000000000, 1.000000000000000000 ) ) ;
#59174=ORIENTED_EDGE ( 'NONE', *, *, #15881, .F. ) ;
#59267=CIRCLE ( 'NONE', #200786, 0.09999999999999939493 ) ;
#59295=CIRCLE ( 'NONE', #26033, 0.09999999999999939493 ) ;
#59299=AXIS2_PLACEMENT_3D ( 'NONE', #174149, #237922, #99669 ) ;
#59351=ORIENTED_EDGE ( 'NONE', *, *, #243676, .F. ) ;
#59360=EDGE_CURVE ( 'NONE', #189932, #122006, #108346, .T. ) ;
#59365=VERTEX_POINT ( 'NONE', #69210 ) ;
#59375=VERTEX_POINT ( 'NONE', #109578 ) ;
#59393=DIRECTION ( 'NONE',  ( 0.000000000000000000, 0.000000000000000000, -1.000000000000000000 ) ) ;
#59471=AXIS2_PLACEMENT_3D ( 'NONE', #24676, #65052, #67617 ) ;
#59508=VERTEX_POINT ( 'NONE', #96426 ) ;
#59536=CARTESIAN_POINT ( 'NONE',  ( 20.00894256274686001, 5.586869314946281584, 16.41686200241345261 ) ) ;
#59541=FACE_OUTER_BOUND ( 'NONE', #217271, .T. ) ;
#59579=ADVANCED_FACE ( 'NONE', ( #16923 ), #237247, .T. ) ;
#59615=DIRECTION ( 'NONE',  ( 0.000000000000000000, 0.1686199900910312910, -0.9856811345164826488 ) ) ;
#59633=ORIENTED_EDGE ( 'NONE', *, *, #83583, .F. ) ;
#59637=VECTOR ( 'NONE', #234392, 1000.000000000000000 ) ;
#59662=CARTESIAN_POINT ( 'NONE',  ( 18.69999999999999574, -8.262584272387851314, 10.47734830970188824 ) ) ;
#59710=DIRECTION ( 'NONE',  ( -1.000000000000000000, 0.000000000000000000, 4.336808689942017736E-16 ) ) ;
#59720=LINE ( 'NONE', #243512, #50464 ) ;
#59727=ORIENTED_EDGE ( 'NONE', *, *, #83209, .T. ) ;
#59729=CARTESIAN_POINT ( 'NONE',  ( -18.69999999999999929, 7.973296578895943121, -1.410778198689825791 ) ) ;
#59743=VERTEX_POINT ( 'NONE', #204524 ) ;
#59806=EDGE_CURVE ( 'NONE', #244339, #53312, #62737, .T. ) ;
#59814=DIRECTION ( 'NONE',  ( -0.000000000000000000, -0.000000000000000000, 1.000000000000000000 ) ) ;
#59822=EDGE_CURVE ( 'NONE', #71927, #75205, #75222, .T. ) ;
#59848=VECTOR ( 'NONE', #221368, 999.9999999999998863 ) ;
#59880=ORIENTED_EDGE ( 'NONE', *, *, #211407, .T. ) ;
#59890=CARTESIAN_POINT ( 'NONE',  ( -20.90000000000000213, 1.885425182446133885, -11.49641995933507843 ) ) ;
#59912=EDGE_LOOP ( 'NONE', ( #111998, #56203, #125994, #106609 ) ) ;
#59918=CARTESIAN_POINT ( 'NONE',  ( -22.94999999999999929, 0.000000000000000000, 0.000000000000000000 ) ) ;
#59974=ORIENTED_EDGE ( 'NONE', *, *, #75148, .T. ) ;
#59993=EDGE_LOOP ( 'NONE', ( #137477, #54404, #149338 ) ) ;
#59997=EDGE_CURVE ( 'NONE', #158566, #62919, #205335, .T. ) ;
#60004=FACE_OUTER_BOUND ( 'NONE', #138295, .T. ) ;
#60021=ORIENTED_EDGE ( 'NONE', *, *, #11882, .T. ) ;
#60108=CARTESIAN_POINT ( 'NONE',  ( 21.00000000000000000, 0.000000000000000000, 0.000000000000000000 ) ) ;
#60143=CIRCLE ( 'NONE', #155858, 0.2000000000000000944 ) ;
#60162=EDGE_CURVE ( 'NONE', #173202, #98368, #37994, .T. ) ;
#60167=EDGE_LOOP ( 'NONE', ( #189022, #42246, #201154, #24896 ) ) ;
#60178=AXIS2_PLACEMENT_3D ( 'NONE', #84664, #43025, #220383 ) ;
#60346=VERTEX_POINT ( 'NONE', #139145 ) ;
#60403=DIRECTION ( 'NONE',  ( 0.000000000000000000, 0.000000000000000000, -1.000000000000000000 ) ) ;
#60410=ORIENTED_EDGE ( 'NONE', *, *, #107069, .F. ) ;
#60423=ADVANCED_FACE ( 'NONE', ( #242118 ), #63476, .F. ) ;
#60496=AXIS2_PLACEMENT_3D ( 'NONE', #254137, #36419, #235861 ) ;
#60532=AXIS2_PLACEMENT_3D ( 'NONE', #188066, #164656, #244165 ) ;
#60570=ORIENTED_EDGE ( 'NONE', *, *, #6348, .F. ) ;
#60579=AXIS2_PLACEMENT_3D ( 'NONE', #113992, #153175, #192275 ) ;
#60668=EDGE_CURVE ( 'NONE', #195790, #167847, #221466, .T. ) ;
#60689=CARTESIAN_POINT ( 'NONE',  ( -37.88850191057539973, -11.65000000000000036, 29.89999999999999858 ) ) ;
#60759=DIRECTION ( 'NONE',  ( 0.000000000000000000, 0.000000000000000000, -1.000000000000000000 ) ) ;
#60772=FACE_OUTER_BOUND ( 'NONE', #137266, .T. ) ;
#60811=CARTESIAN_POINT ( 'NONE',  ( 5.899999999999995914, -11.34999999999999964, 10.10000000000000142 ) ) ;
#60826=EDGE_CURVE ( 'NONE', #91499, #245021, #229872, .T. ) ;
#60847=SPHERICAL_SURFACE ( 'NONE', #244792, 0.1000000000000000056 ) ;
#60954=VERTEX_POINT ( 'NONE', #9632 ) ;
#60958=CARTESIAN_POINT ( 'NONE',  ( 21.00000000000000000, 7.800000000000000711, 1.212568896937007867 ) ) ;
#60966=AXIS2_PLACEMENT_3D ( 'NONE', #52735, #111437, #250927 ) ;
#60978=AXIS2_PLACEMENT_3D ( 'NONE', #150944, #248766, #173120 ) ;
#60998=AXIS2_PLACEMENT_3D ( 'NONE', #176008, #196816, #254214 ) ;
#61011=CARTESIAN_POINT ( 'NONE',  ( 20.90000000000000213, -1.300000000000000044, -7.800000000000000711 ) ) ;
#61024=DIRECTION ( 'NONE',  ( 0.000000000000000000, 0.000000000000000000, 1.000000000000000000 ) ) ;
#61054=FACE_OUTER_BOUND ( 'NONE', #57408, .T. ) ;
#61109=DIRECTION ( 'NONE',  ( 0.000000000000000000, 0.000000000000000000, 1.000000000000000000 ) ) ;
#61121=DIRECTION ( 'NONE',  ( 0.000000000000000000, 0.000000000000000000, -1.000000000000000000 ) ) ;
#61145=ORIENTED_EDGE ( 'NONE', *, *, #13394, .F. ) ;
#61169=DIRECTION ( 'NONE',  ( 0.000000000000000000, 0.000000000000000000, -1.000000000000000000 ) ) ;
#61180=ADVANCED_FACE ( 'NONE', ( #67689 ), #45562, .T. ) ;
#61205=DIRECTION ( 'NONE',  ( 1.000000000000000000, 0.000000000000000000, 0.000000000000000000 ) ) ;
#61210=CARTESIAN_POINT ( 'NONE',  ( 20.90000000000000213, 11.49641995933507843, 1.885425182446133885 ) ) ;
#61261=DIRECTION ( 'NONE',  ( 1.000000000000000000, 0.000000000000000000, 0.000000000000000000 ) ) ;
#61313=VECTOR ( 'NONE', #21933, 1000.000000000000000 ) ;
#61321=ORIENTED_EDGE ( 'NONE', *, *, #16578, .T. ) ;
#61332=DIRECTION ( 'NONE',  ( 0.000000000000000000, -0.1335171055202867274, -0.9910465087640866200 ) ) ;
#61334=LINE ( 'NONE', #20953, #163601 ) ;
#61344=CARTESIAN_POINT ( 'NONE',  ( 18.79999999999999716, 4.513204987021263825, 22.10000000000000142 ) ) ;
#61355=CYLINDRICAL_SURFACE ( 'NONE', #52373, 0.09999999999999939493 ) ;
#61403=ORIENTED_EDGE ( 'NONE', *, *, #79587, .F. ) ;
#61507=CARTESIAN_POINT ( 'NONE',  ( -18.69999999999999929, -10.84999999999999076, -15.00000000000000000 ) ) ;
#61509=AXIS2_PLACEMENT_3D ( 'NONE', #257626, #158621, #238117 ) ;
#61520=DIRECTION ( 'NONE',  ( 0.000000000000000000, 0.000000000000000000, -1.000000000000000000 ) ) ;
#61624=TOROIDAL_SURFACE ( 'NONE', #240680, 4.900000000000003020, 0.1000000000000000056 ) ;
#61670=DIRECTION ( 'NONE',  ( -0.000000000000000000, -1.000000000000000000, 4.336808689942043611E-14 ) ) ;
#61672=AXIS2_PLACEMENT_3D ( 'NONE', #63612, #47888, #244809 ) ;
#61693=CARTESIAN_POINT ( 'NONE',  ( -22.10000000000000497, 6.223900101154157483, 12.09999999999999787 ) ) ;
#61719=EDGE_CURVE ( 'NONE', #160025, #155708, #152076, .T. ) ;
#61724=AXIS2_PLACEMENT_3D ( 'NONE', #30425, #209047, #211625 ) ;
#61768=CIRCLE ( 'NONE', #207543, 0.09999999999999990841 ) ;
#61810=DIRECTION ( 'NONE',  ( 0.000000000000000000, 1.000000000000000000, 0.000000000000000000 ) ) ;
#61838=CARTESIAN_POINT ( 'NONE',  ( -18.79999999999999716, -11.65000000000000036, 32.89999999999999858 ) ) ;
#61858=LINE ( 'NONE', #157122, #245994 ) ;
#61880=LINE ( 'NONE', #205216, #168275 ) ;
#61899=DIRECTION ( 'NONE',  ( 0.000000000000000000, 0.000000000000000000, -1.000000000000000000 ) ) ;
#61907=ORIENTED_EDGE ( 'NONE', *, *, #186327, .F. ) ;
#61920=FACE_OUTER_BOUND ( 'NONE', #108433, .T. ) ;
#61934=EDGE_CURVE ( 'NONE', #14875, #110943, #202729, .T. ) ;
#61935=FACE_OUTER_BOUND ( 'NONE', #92774, .T. ) ;
#62007=DIRECTION ( 'NONE',  ( 0.000000000000000000, 0.000000000000000000, 1.000000000000000000 ) ) ;
#62024=DIRECTION ( 'NONE',  ( -1.000000000000000000, -0.000000000000000000, 0.000000000000000000 ) ) ;
#62066=EDGE_LOOP ( 'NONE', ( #130141, #46186, #220703, #170892 ) ) ;
#62132=EDGE_LOOP ( 'NONE', ( #189944, #110259, #177218, #246173 ) ) ;
#62169=CARTESIAN_POINT ( 'NONE',  ( 20.90000000000000213, -1.410778198689825347, -7.973296578895943121 ) ) ;
#62213=DIRECTION ( 'NONE',  ( 0.000000000000000000, 0.000000000000000000, 1.000000000000000000 ) ) ;
#62225=ORIENTED_EDGE ( 'NONE', *, *, #207196, .T. ) ;
#62236=EDGE_LOOP ( 'NONE', ( #10394, #77926, #224262, #115489 ) ) ;
#62251=ORIENTED_EDGE ( 'NONE', *, *, #159213, .F. ) ;
#62264=ADVANCED_FACE ( 'NONE', ( #116485 ), #173936, .T. ) ;
#62275=CARTESIAN_POINT ( 'NONE',  ( -13.39999999999999858, -8.279289321881348584, 11.02928932188134503 ) ) ;
#62299=DIRECTION ( 'NONE',  ( -1.000000000000000000, 0.000000000000000000, -0.000000000000000000 ) ) ;
#62322=EDGE_CURVE ( 'NONE', #11158, #214793, #255675, .T. ) ;
#62325=DIRECTION ( 'NONE',  ( 0.000000000000000000, 1.000000000000000000, 0.000000000000000000 ) ) ;
#62343=EDGE_CURVE ( 'NONE', #155708, #215605, #139873, .T. ) ;
#62465=ADVANCED_FACE ( 'NONE', ( #99457 ), #39090, .T. ) ;
#62530=CIRCLE ( 'NONE', #220735, 0.09999999999999939493 ) ;
#62539=ORIENTED_EDGE ( 'NONE', *, *, #90052, .F. ) ;
#62576=CARTESIAN_POINT ( 'NONE',  ( -22.94999999999999929, -1.800000000000000044, -11.61130914238355771 ) ) ;
#62607=DIRECTION ( 'NONE',  ( -1.000000000000000000, -0.000000000000000000, -0.000000000000000000 ) ) ;
#62623=ORIENTED_EDGE ( 'NONE', *, *, #4967, .F. ) ;
#62665=EDGE_CURVE ( 'NONE', #57698, #168032, #238597, .T. ) ;
#62694=CARTESIAN_POINT ( 'NONE',  ( -18.79999999999999716, 11.50977166988710820, -1.786320531569725478 ) ) ;
#62716=LINE ( 'NONE', #241363, #254298 ) ;
#62732=ORIENTED_EDGE ( 'NONE', *, *, #139046, .T. ) ;
#62737=CIRCLE ( 'NONE', #225198, 0.1000000000000002554 ) ;
#62738=EDGE_LOOP ( 'NONE', ( #25584, #246883, #243198 ) ) ;
#62777=ADVANCED_FACE ( 'NONE', ( #1339, #43062, #138279, #20955 ), #163023, .T. ) ;
#62787=VERTEX_POINT ( 'NONE', #159181 ) ;
#62826=DIRECTION ( 'NONE',  ( 0.000000000000000000, -0.9910465087640866200, 0.1335171055202867274 ) ) ;
#62857=CARTESIAN_POINT ( 'NONE',  ( -20.90000000000000213, 6.644425182197215562, 9.641788261573355001 ) ) ;
#62871=ORIENTED_EDGE ( 'NONE', *, *, #112716, .T. ) ;
#62882=DIRECTION ( 'NONE',  ( -3.469446951953635015E-14, 0.000000000000000000, -1.000000000000000000 ) ) ;
#62919=VERTEX_POINT ( 'NONE', #208570 ) ;
#62925=TOROIDAL_SURFACE ( 'NONE', #241973, 0.2000000000000000111, 0.1000000000000000056 ) ;
#62933=EDGE_LOOP ( 'NONE', ( #154132, #183041, #155430, #89523 ) ) ;
#62947=EDGE_LOOP ( 'NONE', ( #24506, #239906, #253658, #26143 ) ) ;
#62948=DIRECTION ( 'NONE',  ( 0.000000000000000000, 1.000000000000000000, 0.000000000000000000 ) ) ;
#62984=CYLINDRICAL_SURFACE ( 'NONE', #38972, 0.1000000000000028644 ) ;
#62996=AXIS2_PLACEMENT_3D ( 'NONE', #14051, #31068, #110561 ) ;
#63029=AXIS2_PLACEMENT_3D ( 'NONE', #72570, #93388, #172977 ) ;
#63052=EDGE_CURVE ( 'NONE', #19574, #118769, #63818, .T. ) ;
#63077=AXIS2_PLACEMENT_3D ( 'NONE', #201714, #163886, #62213 ) ;
#63102=EDGE_LOOP ( 'NONE', ( #123985, #128777, #119138, #242085 ) ) ;
#63104=AXIS2_PLACEMENT_3D ( 'NONE', #15202, #94713, #174312 ) ;
#63192=CARTESIAN_POINT ( 'NONE',  ( -18.79999999999999716, -1.885425182446133885, -11.49641995933507843 ) ) ;
#63226=EDGE_LOOP ( 'NONE', ( #55728, #39495, #150778, #44623 ) ) ;
#63246=ORIENTED_EDGE ( 'NONE', *, *, #59806, .F. ) ;
#63251=DIRECTION ( 'NONE',  ( 0.000000000000000000, -5.204170427930272346E-14, -1.000000000000000000 ) ) ;
#63256=EDGE_CURVE ( 'NONE', #102889, #181190, #129656, .T. ) ;
#63338=ORIENTED_EDGE ( 'NONE', *, *, #124177, .F. ) ;
#63341=CARTESIAN_POINT ( 'NONE',  ( -18.79999999999999716, 1.212568896937007645, -7.800000000000000711 ) ) ;
#63365=EDGE_CURVE ( 'NONE', #103469, #172629, #163949, .T. ) ;
#63379=LINE ( 'NONE', #47661, #99232 ) ;
#63427=EDGE_CURVE ( 'NONE', #141175, #181190, #215599, .T. ) ;
#63429=VERTEX_POINT ( 'NONE', #172686 ) ;
#63458=ADVANCED_FACE ( 'NONE', ( #214331 ), #116522, .T. ) ;
#63476=CYLINDRICAL_SURFACE ( 'NONE', #63077, 0.09999999999999939493 ) ;
#63505=FACE_OUTER_BOUND ( 'NONE', #126185, .T. ) ;
#63518=ORIENTED_EDGE ( 'NONE', *, *, #80296, .T. ) ;
#63541=EDGE_CURVE ( 'NONE', #109914, #47140, #251434, .T. ) ;
#63567=EDGE_CURVE ( 'NONE', #75404, #30076, #181638, .T. ) ;
#63568=CARTESIAN_POINT ( 'NONE',  ( -19.89999999999999858, 1.350000000000000089, 21.90000000000000213 ) ) ;
#63572=ORIENTED_EDGE ( 'NONE', *, *, #133215, .T. ) ;
#63612=CARTESIAN_POINT ( 'NONE',  ( 22.94999999999999929, 0.000000000000000000, 0.000000000000000000 ) ) ;
#63613=CONICAL_SURFACE ( 'NONE', #34600, 4.000000000000000000, 0.7853981633974489451 ) ;
#63621=ADVANCED_FACE ( 'NONE', ( #188052 ), #147630, .F. ) ;
#63624=ORIENTED_EDGE ( 'NONE', *, *, #240200, .F. ) ;
#63677=DIRECTION ( 'NONE',  ( 1.000000000000000000, -0.000000000000000000, -0.000000000000000000 ) ) ;
#63704=FACE_OUTER_BOUND ( 'NONE', #106636, .T. ) ;
#63710=VERTEX_POINT ( 'NONE', #86340 ) ;
#63726=AXIS2_PLACEMENT_3D ( 'NONE', #201919, #63677, #243607 ) ;
#63727=DIRECTION ( 'NONE',  ( 1.000000000000000000, 0.000000000000000000, 0.000000000000000000 ) ) ;
#63738=CARTESIAN_POINT ( 'NONE',  ( 22.10000000000000497, 6.223900101154157483, 12.00000000000000000 ) ) ;
#63792=DIRECTION ( 'NONE',  ( -1.000000000000000000, -0.000000000000000000, -0.000000000000000000 ) ) ;
#63813=CIRCLE ( 'NONE', #205435, 0.09999999999999989453 ) ;
#63815=DIRECTION ( 'NONE',  ( 0.000000000000000000, 0.1686199900910312910, -0.9856811345164826488 ) ) ;
#63818=CIRCLE ( 'NONE', #188698, 0.09999999999999996392 ) ;
#63830=DIRECTION ( 'NONE',  ( 0.000000000000000000, 0.000000000000000000, -1.000000000000000000 ) ) ;
#63867=CARTESIAN_POINT ( 'NONE',  ( 19.90000000000000924, 4.513204987021263825, 22.00000000000000355 ) ) ;
#63875=EDGE_CURVE ( 'NONE', #109914, #256719, #180885, .T. ) ;
#63881=CARTESIAN_POINT ( 'NONE',  ( -21.00000000000000000, 0.000000000000000000, 0.000000000000000000 ) ) ;
#63931=ORIENTED_EDGE ( 'NONE', *, *, #64667, .T. ) ;
#63932=EDGE_LOOP ( 'NONE', ( #231003, #21213, #37116, #46028 ) ) ;
#63941=ORIENTED_EDGE ( 'NONE', *, *, #99081, .T. ) ;
#63944=ORIENTED_EDGE ( 'NONE', *, *, #11529, .T. ) ;
#63951=DIRECTION ( 'NONE',  ( 1.000000000000000000, 0.000000000000000000, 0.000000000000000000 ) ) ;
#63958=CARTESIAN_POINT ( 'NONE',  ( 13.40000000000000036, -9.650000000000002132, 12.40000000000000391 ) ) ;
#63960=ORIENTED_EDGE ( 'NONE', *, *, #191204, .T. ) ;
#63980=CARTESIAN_POINT ( 'NONE',  ( -22.94999999999999929, -1.885425182446134107, -11.49641995933507843 ) ) ;
#64007=ADVANCED_FACE ( 'NONE', ( #38968 ), #36411, .T. ) ;
#64010=DIRECTION ( 'NONE',  ( 0.000000000000000000, -0.8741572761215355980, 0.4856429311786357172 ) ) ;
#64020=DIRECTION ( 'NONE',  ( 1.000000000000000000, -0.000000000000000000, 0.000000000000000000 ) ) ;
#64044=DIRECTION ( 'NONE',  ( 1.000000000000000000, 0.000000000000000000, -0.000000000000000000 ) ) ;
#64132=ORIENTED_EDGE ( 'NONE', *, *, #165993, .F. ) ;
#64163=AXIS2_PLACEMENT_3D ( 'NONE', #213690, #95024, #91182 ) ;
#64170=CARTESIAN_POINT ( 'NONE',  ( -0.8999999999999993561, -8.250000000000005329, 26.00000000000000355 ) ) ;
#64180=DIRECTION ( 'NONE',  ( 0.000000000000000000, 0.1335171055202867274, 0.9910465087640866200 ) ) ;
#64215=DIRECTION ( 'NONE',  ( 1.000000000000000000, -0.000000000000000000, -0.000000000000000000 ) ) ;
#64231=AXIS2_PLACEMENT_3D ( 'NONE', #235582, #56920, #136467 ) ;
#64302=DIRECTION ( 'NONE',  ( 0.000000000000000000, -0.9910465087640860649, -0.1335171055202901413 ) ) ;
#64304=CIRCLE ( 'NONE', #147517, 11.75000000000000000 ) ;
#64337=DIRECTION ( 'NONE',  ( 0.000000000000000000, 0.9856811345164803173, 0.1686199900910455851 ) ) ;
#64339=EDGE_CURVE ( 'NONE', #142179, #22186, #175600, .T. ) ;
#64400=ORIENTED_EDGE ( 'NONE', *, *, #133954, .F. ) ;
#64404=DIRECTION ( 'NONE',  ( 0.000000000000000000, 1.000000000000000000, 1.445602896647339410E-16 ) ) ;
#64433=DIRECTION ( 'NONE',  ( 0.000000000000000000, 0.000000000000000000, -1.000000000000000000 ) ) ;
#64495=ORIENTED_EDGE ( 'NONE', *, *, #176486, .F. ) ;
#64580=VECTOR ( 'NONE', #62024, 1000.000000000000000 ) ;
#64588=CARTESIAN_POINT ( 'NONE',  ( 0.000000000000000000, 1.350000000000000089, 21.90000000000000213 ) ) ;
#64589=EDGE_CURVE ( 'NONE', #975, #98150, #210249, .T. ) ;
#64663=SURFACE_STYLE_USAGE ( .BOTH. , #84169 ) ;
#64667=EDGE_CURVE ( 'NONE', #41516, #57247, #22334, .T. ) ;
#64680=LINE ( 'NONE', #123383, #166023 ) ;
#64707=AXIS2_PLACEMENT_3D ( 'NONE', #132913, #230731, #212453 ) ;
#64795=CYLINDRICAL_SURFACE ( 'NONE', #70906, 0.09999999999999939493 ) ;
#64801=AXIS2_PLACEMENT_3D ( 'NONE', #83799, #82526, #42166 ) ;
#64864=VECTOR ( 'NONE', #234330, 1000.000000000000000 ) ;
#64898=DIRECTION ( 'NONE',  ( 0.000000000000000000, -1.000000000000000000, 0.000000000000000000 ) ) ;
#64938=CARTESIAN_POINT ( 'NONE',  ( 18.79999999999999716, -1.885425182446134107, -11.49641995933507843 ) ) ;
#64971=DIRECTION ( 'NONE',  ( 1.000000000000000000, 0.000000000000000000, -0.000000000000000000 ) ) ;
#64977=( BOUNDED_SURFACE ( )  B_SPLINE_SURFACE ( 3, 2, ( 
 ( #249206, #150119, #210082 ),
 ( #96203, #250468, #31466 ),
 ( #110967, #175777, #255233 ),
 ( #190533, #97467, #256505 ) ),
 .UNSPECIFIED., .F., .F., .T. ) 
 B_SPLINE_SURFACE_WITH_KNOTS ( ( 4, 4 ),
 ( 3, 3 ),
 ( 1.570796326794896558, 3.141592653589793116 ),
 ( 0.000000000000000000, 1.000000000000000000 ),
 .UNSPECIFIED. ) 
 GEOMETRIC_REPRESENTATION_ITEM ( )  RATIONAL_B_SPLINE_SURFACE ( (
 ( 1.000000000000000000, 0.7071067811865505703, 1.000000000000000000),
 ( 1.000000000000000000, 0.6753870962079620011, 1.000000000000000000),
 ( 1.000000000000000000, 0.6438648806865411300, 1.000000000000000000),
 ( 1.000000000000000000, 0.6447402616205117898, 1.000000000000000000) ) ) 
 REPRESENTATION_ITEM ( '' )  SURFACE ( )  );
#64983=CARTESIAN_POINT ( 'NONE',  ( 18.59999999999999787, -9.849999999999994316, 30.00000000000000000 ) ) ;
#64993=ORIENTED_EDGE ( 'NONE', *, *, #200081, .F. ) ;
#65010=ORIENTED_EDGE ( 'NONE', *, *, #10148, .F. ) ;
#65049=CIRCLE ( 'NONE', #210792, 0.1000000000000000472 ) ;
#65052=DIRECTION ( 'NONE',  ( -0.000000000000000000, 1.000000000000000000, -0.000000000000000000 ) ) ;
#65073=DIRECTION ( 'NONE',  ( 1.284434275755705789E-16, -0.7071067811865472397, 0.7071067811865479058 ) ) ;
#65091=TOROIDAL_SURFACE ( 'NONE', #215293, 11.65000000000000036, 0.1000000000000000056 ) ;
#65140=CIRCLE ( 'NONE', #98416, 0.09999999999999939493 ) ;
#65187=VECTOR ( 'NONE', #64302, 1000.000000000000114 ) ;
#65191=MECHANICAL_DESIGN_GEOMETRIC_PRESENTATION_REPRESENTATION('',(#11027),#210944);
#65209=ORIENTED_EDGE ( 'NONE', *, *, #128994, .T. ) ;
#65256=EDGE_LOOP ( 'NONE', ( #207937, #160906, #51981, #151032, #99885, #37082, #188035 ) ) ;
#65257=FACE_OUTER_BOUND ( 'NONE', #38871, .T. ) ;
#65268=CIRCLE ( 'NONE', #131908, 0.1000000000000000472 ) ;
#65297=VECTOR ( 'NONE', #98763, 1000.000000000000000 ) ;
#65318=CARTESIAN_POINT ( 'NONE',  ( -21.00000000000000000, 5.021051876504148371E-16, -4.100000000000000533 ) ) ;
#65340=TOROIDAL_SURFACE ( 'NONE', #219438, 0.2000000000000000111, 0.1000000000000000056 ) ;
#65399=ORIENTED_EDGE ( 'NONE', *, *, #229667, .T. ) ;
#65406=AXIS2_PLACEMENT_3D ( 'NONE', #5834, #26731, #65826 ) ;
#65437=DIRECTION ( 'NONE',  ( -1.000000000000000000, -0.000000000000000000, 0.000000000000000000 ) ) ;
#65467=CARTESIAN_POINT ( 'NONE',  ( -19.99999999999999645, 4.547418889303921574, 21.90000000000000213 ) ) ;
#65491=ORIENTED_EDGE ( 'NONE', *, *, #196890, .F. ) ;
#65493=ORIENTED_EDGE ( 'NONE', *, *, #225939, .F. ) ;
#65560=EDGE_LOOP ( 'NONE', ( #106860, #20857, #113733, #32327 ) ) ;
#65582=LINE ( 'NONE', #163412, #65187 ) ;
#65718=AXIS2_PLACEMENT_3D ( 'NONE', #231879, #233164, #16676 ) ;
#65780=DIRECTION ( 'NONE',  ( -4.336808689942017736E-16, 0.000000000000000000, -1.000000000000000000 ) ) ;
#65791=AXIS2_PLACEMENT_3D ( 'NONE', #2561, #179944, #101639 ) ;
#65796=CARTESIAN_POINT ( 'NONE',  ( 18.79999999999999716, 7.986648289447971116, -1.311673547813416718 ) ) ;
#65817=ORIENTED_EDGE ( 'NONE', *, *, #146470, .T. ) ;
#65826=DIRECTION ( 'NONE',  ( 0.000000000000000000, 0.000000000000000000, 1.000000000000000000 ) ) ;
#65828=ORIENTED_EDGE ( 'NONE', *, *, #1267, .T. ) ;
#65847=CIRCLE ( 'NONE', #11712, 0.1000000000000001443 ) ;
#65862=ORIENTED_EDGE ( 'NONE', *, *, #187979, .T. ) ;
#65886=EDGE_CURVE ( 'NONE', #193899, #82204, #213157, .T. ) ;
#65906=VERTEX_POINT ( 'NONE', #143888 ) ;
#65928=ORIENTED_EDGE ( 'NONE', *, *, #128534, .F. ) ;
#66014=DIRECTION ( 'NONE',  ( -0.000000000000000000, 0.000000000000000000, 1.000000000000000000 ) ) ;
#66027=SPHERICAL_SURFACE ( 'NONE', #113487, 0.1000000000000000056 ) ;
#66082=ADVANCED_FACE ( 'NONE', ( #250693 ), #9513, .F. ) ;
#66085=CARTESIAN_POINT ( 'NONE',  ( 18.79999999999999716, -1.212568896937008089, -7.800000000000000711 ) ) ;
#66088=EDGE_CURVE ( 'NONE', #128297, #102889, #151634, .T. ) ;
#66123=VERTEX_POINT ( 'NONE', #95474 ) ;
#66184=CIRCLE ( 'NONE', #166752, 0.09999999999999939493 ) ;
#66192=CYLINDRICAL_SURFACE ( 'NONE', #201166, 0.09999999999999939493 ) ;
#66193=ORIENTED_EDGE ( 'NONE', *, *, #207196, .F. ) ;
#66213=ORIENTED_EDGE ( 'NONE', *, *, #175695, .F. ) ;
#66260=DIRECTION ( 'NONE',  ( 0.000000000000000000, 1.000000000000000000, 0.000000000000000000 ) ) ;
#66301=CIRCLE ( 'NONE', #16243, 0.2000000000000000944 ) ;
#66303=EDGE_LOOP ( 'NONE', ( #171856, #225836, #252669, #28105 ) ) ;
#66309=DIRECTION ( 'NONE',  ( 0.000000000000000000, -0.4856429311786307212, -0.8741572761215384846 ) ) ;
#66381=CARTESIAN_POINT ( 'NONE',  ( 22.19999999999999929, -1.467286812112899463, 32.89999999999999858 ) ) ;
#66390=ADVANCED_FACE ( 'NONE', ( #165414 ), #244935, .F. ) ;
#66395=VERTEX_POINT ( 'NONE', #27212 ) ;
#66482=VERTEX_POINT ( 'NONE', #113134 ) ;
#66505=CARTESIAN_POINT ( 'NONE',  ( 20.90000000000000213, 7.886648289447972360, 1.399104650876408451 ) ) ;
#66534=EDGE_CURVE ( 'NONE', #130825, #150252, #50565, .T. ) ;
#66552=EDGE_CURVE ( 'NONE', #125866, #3738, #148862, .T. ) ;
#66639=ORIENTED_EDGE ( 'NONE', *, *, #90004, .F. ) ;
#66659=CARTESIAN_POINT ( 'NONE',  ( 5.899999999999995914, -11.75000000000000000, 10.10000000000000142 ) ) ;
#66662=DIRECTION ( 'NONE',  ( 0.000000000000000000, 0.000000000000000000, 1.000000000000000000 ) ) ;
#66727=ORIENTED_EDGE ( 'NONE', *, *, #219564, .F. ) ;
#66737=DIRECTION ( 'NONE',  ( 0.000000000000000000, 0.000000000000000000, 1.000000000000000000 ) ) ;
#66762=CARTESIAN_POINT ( 'NONE',  ( -0.8999999999999993561, -11.65000000000000036, 26.00000000000000355 ) ) ;
#66767=DIRECTION ( 'NONE',  ( -0.000000000000000000, 0.1335171055202901413, -0.9910465087640860649 ) ) ;
#66774=DIRECTION ( 'NONE',  ( 0.000000000000000000, 0.000000000000000000, 1.000000000000000000 ) ) ;
#66836=CYLINDRICAL_SURFACE ( 'NONE', #218938, 0.09999999999999939493 ) ;
#66878=DIRECTION ( 'NONE',  ( 0.000000000000000000, -1.000000000000000000, 0.000000000000000000 ) ) ;
#66926=DIRECTION ( 'NONE',  ( 1.000000000000000000, 0.000000000000000000, 0.000000000000000000 ) ) ;
#66961=VERTEX_POINT ( 'NONE', #98341 ) ;
#67035=CARTESIAN_POINT ( 'NONE',  ( -6.000000000000002665, -11.34999999999999964, 13.90000000000000213 ) ) ;
#67056=ADVANCED_FACE ( 'NONE', ( #5679 ), #200065, .T. ) ;
#67059=VERTEX_POINT ( 'NONE', #186944 ) ;
#67071=CYLINDRICAL_SURFACE ( 'NONE', #210035, 0.1000000000000002554 ) ;
#67096=AXIS2_PLACEMENT_3D ( 'NONE', #192159, #13511, #50052 ) ;
#67112=CARTESIAN_POINT ( 'NONE',  ( -22.94999999999999929, 0.000000000000000000, 3.900000000000000355 ) ) ;
#67205=CARTESIAN_POINT ( 'NONE',  ( -22.94999999999999929, 8.000000000000000000, -1.212568896937008089 ) ) ;
#67214=FACE_OUTER_BOUND ( 'NONE', #167492, .T. ) ;
#67246=DIRECTION ( 'NONE',  ( 0.000000000000000000, 0.000000000000000000, 1.000000000000000000 ) ) ;
#67260=CARTESIAN_POINT ( 'NONE',  ( 20.90000000000000213, 1.212568896937007645, -7.800000000000000711 ) ) ;
#67263=VECTOR ( 'NONE', #203308, 1000.000000000000000 ) ;
#67267=ORIENTED_EDGE ( 'NONE', *, *, #227709, .T. ) ;
#67290=DIRECTION ( 'NONE',  ( 1.000000000000000000, -0.000000000000000000, 0.000000000000000000 ) ) ;
#67301=DIRECTION ( 'NONE',  ( -1.000000000000000000, 0.000000000000000000, 0.000000000000000000 ) ) ;
#67311=EDGE_CURVE ( 'NONE', #98899, #164655, #90936, .T. ) ;
#67366=AXIS2_PLACEMENT_3D ( 'NONE', #3206, #243116, #237971 ) ;
#67424=CARTESIAN_POINT ( 'NONE',  ( 18.79999999999999716, -11.65000000000000036, 0.000000000000000000 ) ) ;
#67433=CARTESIAN_POINT ( 'NONE',  ( -37.88850191057539973, -14.35849056603774976, -0.4952830188679671064 ) ) ;
#67457=VECTOR ( 'NONE', #114116, 1000.000000000000227 ) ;
#67512=DIRECTION ( 'NONE',  ( 0.000000000000000000, 0.1335171055202867274, -0.9910465087640865089 ) ) ;
#67517=DIRECTION ( 'NONE',  ( 0.000000000000000000, 0.000000000000000000, 1.000000000000000000 ) ) ;
#67545=FACE_OUTER_BOUND ( 'NONE', #59912, .T. ) ;
#67588=CARTESIAN_POINT ( 'NONE',  ( -18.69999999999999929, 10.31653824539118069, -11.82383137372478110 ) ) ;
#67600=DIRECTION ( 'NONE',  ( 0.000000000000000000, 0.000000000000000000, 1.000000000000000000 ) ) ;
#67617=DIRECTION ( 'NONE',  ( 0.000000000000000000, 0.000000000000000000, 1.000000000000000000 ) ) ;
#67631=AXIS2_PLACEMENT_3D ( 'NONE', #3613, #204379, #27071 ) ;
#67689=FACE_OUTER_BOUND ( 'NONE', #89785, .T. ) ;
#67691=CYLINDRICAL_SURFACE ( 'NONE', #191274, 0.09999999999999939493 ) ;
#67724=AXIS2_PLACEMENT_3D ( 'NONE', #125681, #200091, #21470 ) ;
#67773=DIRECTION ( 'NONE',  ( -1.000000000000000000, 0.000000000000000000, 0.000000000000000000 ) ) ;
#67794=AXIS2_PLACEMENT_3D ( 'NONE', #959, #160097, #80497 ) ;
#67838=LINE ( 'NONE', #147381, #998 ) ;
#67849=CARTESIAN_POINT ( 'NONE',  ( 21.00000000000000000, 0.000000000000000000, -7.800000000000000711 ) ) ;
#67858=VERTEX_POINT ( 'NONE', #195987 ) ;
#67939=EDGE_CURVE ( 'NONE', #97490, #131374, #99411, .T. ) ;
#67954=CYLINDRICAL_SURFACE ( 'NONE', #7635, 0.1000000000000002554 ) ;
#67992=EDGE_CURVE ( 'NONE', #173202, #184295, #53145, .T. ) ;
#67997=DIRECTION ( 'NONE',  ( 1.000000000000000000, 0.000000000000000000, 0.000000000000000000 ) ) ;
#68037=CARTESIAN_POINT ( 'NONE',  ( -20.00894256274684224, 4.611773101055291590, 22.11686199560476140 ) ) ;
#68043=FACE_OUTER_BOUND ( 'NONE', #172534, .T. ) ;
#68087=ORIENTED_EDGE ( 'NONE', *, *, #114524, .F. ) ;
#68088=EDGE_CURVE ( 'NONE', #248699, #217909, #84970, .T. ) ;
#68136=ORIENTED_EDGE ( 'NONE', *, *, #102329, .F. ) ;
#68146=EDGE_CURVE ( 'NONE', #25360, #172629, #49041, .T. ) ;
#68151=ORIENTED_EDGE ( 'NONE', *, *, #242015, .T. ) ;
#68160=AXIS2_PLACEMENT_3D ( 'NONE', #23808, #81160, #223240 ) ;
#68165=EDGE_CURVE ( 'NONE', #103588, #30076, #82335, .T. ) ;
#68226=AXIS2_PLACEMENT_3D ( 'NONE', #254013, #157537, #54537 ) ;
#68261=ORIENTED_EDGE ( 'NONE', *, *, #133631, .F. ) ;
#68278=ORIENTED_EDGE ( 'NONE', *, *, #170387, .F. ) ;
#68292=ORIENTED_EDGE ( 'NONE', *, *, #26730, .F. ) ;
#68301=ADVANCED_FACE ( 'NONE', ( #1290 ), #78264, .T. ) ;
#68314=DIRECTION ( 'NONE',  ( 1.000000000000000000, 0.000000000000000000, 0.000000000000000000 ) ) ;
#68383=DIRECTION ( 'NONE',  ( 0.000000000000000000, -1.000000000000000000, 0.000000000000000000 ) ) ;
#68464=CARTESIAN_POINT ( 'NONE',  ( 22.94999999999999929, 4.837354856632045057E-16, 3.900000000000000355 ) ) ;
#68470=CARTESIAN_POINT ( 'NONE',  ( -5.900000000000003020, -11.65000000000000036, 10.00000000000000178 ) ) ;
#68495=ORIENTED_EDGE ( 'NONE', *, *, #106225, .F. ) ;
#68501=DIRECTION ( 'NONE',  ( 1.000000000000000000, 0.000000000000000000, -0.000000000000000000 ) ) ;
#68520=ORIENTED_EDGE ( 'NONE', *, *, #233015, .T. ) ;
#68530=ORIENTED_EDGE ( 'NONE', *, *, #254250, .F. ) ;
#68594=CARTESIAN_POINT ( 'NONE',  ( 18.79999999999999716, 4.513204987021263825, 22.00000000000000355 ) ) ;
#68605=AXIS2_PLACEMENT_3D ( 'NONE', #219745, #18977, #176800 ) ;
#68618=ADVANCED_FACE ( 'NONE', ( #93681 ), #187283, .T. ) ;
#68624=CARTESIAN_POINT ( 'NONE',  ( -22.19999999999999929, -11.65000000000000036, -15.00000000000000000 ) ) ;
#68657=VECTOR ( 'NONE', #215359, 1000.000000000000000 ) ;
#68694=CIRCLE ( 'NONE', #110372, 0.2000000000000000944 ) ;
#68704=ORIENTED_EDGE ( 'NONE', *, *, #84864, .F. ) ;
#68729=CIRCLE ( 'NONE', #114515, 0.09999999999999939493 ) ;
#68749=CARTESIAN_POINT ( 'NONE',  ( -18.79999999999999716, 1.885425182446133885, -11.49641995933507843 ) ) ;
#68784=AXIS2_PLACEMENT_3D ( 'NONE', #233413, #195566, #191726 ) ;
#68840=EDGE_CURVE ( 'NONE', #212150, #16688, #105780, .T. ) ;
#68855=( NAMED_UNIT ( * ) SI_UNIT ( $, .STERADIAN. ) SOLID_ANGLE_UNIT ( ) );
#68861=CARTESIAN_POINT ( 'NONE',  ( -13.40000000000000036, -8.250000000000007105, 12.40000000000000391 ) ) ;
#68864=CYLINDRICAL_SURFACE ( 'NONE', #73812, 4.000000000000000000 ) ;
#68881=CIRCLE ( 'NONE', #131394, 2.600000000000001421 ) ;
#68909=COLOUR_RGB ( '', 0.72549020, 0.75294118, 0.79215686) ;
#68927=VECTOR ( 'NONE', #35001, 1000.000000000000000 ) ;
#68932=CARTESIAN_POINT ( 'NONE',  ( 18.79999999999999716, -11.75000000000000178, 0.000000000000000000 ) ) ;
#68950=AXIS2_PLACEMENT_3D ( 'NONE', #118347, #154925, #157498 ) ;
#68957=FACE_OUTER_BOUND ( 'NONE', #134748, .T. ) ;
#68971=EDGE_CURVE ( 'NONE', #82535, #195496, #208203, .T. ) ;
#69056=CARTESIAN_POINT ( 'NONE',  ( 11.60000000000000142, -8.250000000000005329, 15.00000000000000355 ) ) ;
#69058=CARTESIAN_POINT ( 'NONE',  ( -18.79999999999999716, 1.410778198689825347, -7.973296578895943121 ) ) ;
#69064=CARTESIAN_POINT ( 'NONE',  ( 20.90000000000000213, 11.49641995933507843, 1.885425182446133885 ) ) ;
#69069=DIRECTION ( 'NONE',  ( 0.000000000000000000, 0.000000000000000000, -1.000000000000000000 ) ) ;
#69091=ORIENTED_EDGE ( 'NONE', *, *, #96767, .T. ) ;
#69098=CARTESIAN_POINT ( 'NONE',  ( 18.59999999999999787, 11.75000000000000000, 6.000000000000001776 ) ) ;
#69200=EDGE_LOOP ( 'NONE', ( #73294, #80917, #43899, #105525 ) ) ;
#69208=EDGE_LOOP ( 'NONE', ( #228431, #195043, #130396, #8316, #233271, #40362, #105056, #105214, #60410, #189327, #89773, #210410, #109340, #15652, #40397, #218545 ) ) ;
#69210=CARTESIAN_POINT ( 'NONE',  ( 18.69999999999999929, -1.212568896937008089, -7.800000000000000711 ) ) ;
#69216=CARTESIAN_POINT ( 'NONE',  ( 19.90000000000000924, 4.611773100472912112, 22.11686199900910665 ) ) ;
#69263=CIRCLE ( 'NONE', #165106, 0.09999999999999939493 ) ;
#69268=CARTESIAN_POINT ( 'NONE',  ( -22.10000000000000497, 3.461118860469513336, 28.84309995045515507 ) ) ;
#69276=DIRECTION ( 'NONE',  ( 1.000000000000000000, -0.000000000000000000, 0.000000000000000000 ) ) ;
#69293=EDGE_CURVE ( 'NONE', #227995, #28763, #164090, .T. ) ;
#69299=LINE ( 'NONE', #246624, #234638 ) ;
#69309=ORIENTED_EDGE ( 'NONE', *, *, #49354, .F. ) ;
#69359=EDGE_CURVE ( 'NONE', #242362, #17438, #34945, .T. ) ;
#69389=ADVANCED_FACE ( 'NONE', ( #190587 ), #233559, .T. ) ;
#69407=AXIS2_PLACEMENT_3D ( 'NONE', #180008, #202126, #1333 ) ;
#69426=ORIENTED_EDGE ( 'NONE', *, *, #240656, .T. ) ;
#69445=ORIENTED_EDGE ( 'NONE', *, *, #219405, .T. ) ;
#69468=VERTEX_POINT ( 'NONE', #78305 ) ;
#69492=DIRECTION ( 'NONE',  ( 0.000000000000000000, -1.000000000000000000, 0.000000000000000000 ) ) ;
#69549=CARTESIAN_POINT ( 'NONE',  ( -22.94999999999999929, 6.841561409100513025, 9.675512259591560138 ) ) ;
#69570=VERTEX_POINT ( 'NONE', #80867 ) ;
#69586=ORIENTED_EDGE ( 'NONE', *, *, #181630, .F. ) ;
#69588=ORIENTED_EDGE ( 'NONE', *, *, #234361, .T. ) ;
#69600=DIRECTION ( 'NONE',  ( 0.000000000000000000, 0.000000000000000000, -1.000000000000000000 ) ) ;
#69625=EDGE_CURVE ( 'NONE', #36331, #190169, #22638, .T. ) ;
#69634=PRODUCT_DEFINITION_FORMATION_WITH_SPECIFIED_SOURCE ( 'ANY', '', #70236, .NOT_KNOWN. ) ;
#69670=DIRECTION ( 'NONE',  ( -0.000000000000000000, 1.000000000000000000, -0.000000000000000000 ) ) ;
#69686=DIRECTION ( 'NONE',  ( 1.000000000000000000, 0.000000000000000000, -0.000000000000000000 ) ) ;
#69699=CIRCLE ( 'NONE', #115462, 0.1000000000000002554 ) ;
#69734=LINE ( 'NONE', #209220, #231384 ) ;
#69823=ADVANCED_FACE ( 'NONE', ( #31232 ), #153759, .F. ) ;
#69858=AXIS2_PLACEMENT_3D ( 'NONE', #247121, #59814, #140657 ) ;
#69908=EDGE_CURVE ( 'NONE', #37087, #5080, #156104, .T. ) ;
#69923=ORIENTED_EDGE ( 'NONE', *, *, #20655, .T. ) ;
#69931=ORIENTED_EDGE ( 'NONE', *, *, #217302, .T. ) ;
#69944=ORIENTED_EDGE ( 'NONE', *, *, #142423, .F. ) ;
#69982=EDGE_CURVE ( 'NONE', #254397, #163777, #218786, .T. ) ;
#70003=EDGE_CURVE ( 'NONE', #154676, #163656, #147893, .T. ) ;
#70051=ORIENTED_EDGE ( 'NONE', *, *, #183764, .T. ) ;
#70052=DIRECTION ( 'NONE',  ( 0.000000000000000000, 0.000000000000000000, -1.000000000000000000 ) ) ;
#70054=EDGE_CURVE ( 'NONE', #192900, #7521, #44015, .T. ) ;
#70070=CIRCLE ( 'NONE', #136670, 0.09999999999999963085 ) ;
#70077=CIRCLE ( 'NONE', #186779, 0.09999999999999990841 ) ;
#70084=DIRECTION ( 'NONE',  ( 0.000000000000000000, 0.000000000000000000, 1.000000000000000000 ) ) ;
#70136=ORIENTED_EDGE ( 'NONE', *, *, #6400, .F. ) ;
#70167=VERTEX_POINT ( 'NONE', #10024 ) ;
#70178=ORIENTED_EDGE ( 'NONE', *, *, #129936, .F. ) ;
#70186=DIRECTION ( 'NONE',  ( 0.000000000000000000, 0.000000000000000000, -1.000000000000000000 ) ) ;
#70236=PRODUCT ( 'Fixed End Mounting Bracket', 'Fixed End Mounting Bracket', '', ( #100313 ) ) ;
#70271=ORIENTED_EDGE ( 'NONE', *, *, #11876, .F. ) ;
#70290=DIRECTION ( 'NONE',  ( -0.000000000000000000, 1.000000000000000000, -0.000000000000000000 ) ) ;
#70307=DIRECTION ( 'NONE',  ( 0.000000000000000000, -0.000000000000000000, 1.000000000000000000 ) ) ;
#70317=AXIS2_PLACEMENT_3D ( 'NONE', #185536, #207680, #51130 ) ;
#70320=AXIS2_PLACEMENT_3D ( 'NONE', #6690, #84912, #223161 ) ;
#70370=VERTEX_POINT ( 'NONE', #58108 ) ;
#70395=CARTESIAN_POINT ( 'NONE',  ( 18.59999999999999787, -9.849999999999994316, 30.09999999999999076 ) ) ;
#70445=ORIENTED_EDGE ( 'NONE', *, *, #236743, .F. ) ;
#70456=CARTESIAN_POINT ( 'NONE',  ( -0.000000000000000000, -11.25000000000000000, 10.10000000000000142 ) ) ;
#70470=CARTESIAN_POINT ( 'NONE',  ( -21.10000000000000142, -11.64999999999999858, 11.89999999999999680 ) ) ;
#70481=FACE_OUTER_BOUND ( 'NONE', #215145, .T. ) ;
#70520=AXIS2_PLACEMENT_3D ( 'NONE', #20791, #83277, #199428 ) ;
#70542=ORIENTED_EDGE ( 'NONE', *, *, #182490, .F. ) ;
#70568=LINE ( 'NONE', #127946, #143450 ) ;
#70588=CIRCLE ( 'NONE', #78892, 0.1000000000000000749 ) ;
#70594=EDGE_CURVE ( 'NONE', #149638, #28763, #202238, .T. ) ;
#70640=ADVANCED_FACE ( 'NONE', ( #55227 ), #237749, .T. ) ;
#70651=ORIENTED_EDGE ( 'NONE', *, *, #122964, .F. ) ;
#70681=EDGE_CURVE ( 'NONE', #129072, #246378, #139855, .T. ) ;
#70694=AXIS2_PLACEMENT_3D ( 'NONE', #242372, #105403, #183703 ) ;
#70728=VERTEX_POINT ( 'NONE', #25146 ) ;
#70732=FACE_OUTER_BOUND ( 'NONE', #201248, .T. ) ;
#70746=SPHERICAL_SURFACE ( 'NONE', #25386, 0.1000000000000000056 ) ;
#70763=AXIS2_PLACEMENT_3D ( 'NONE', #20446, #99931, #94820 ) ;
#70802=CARTESIAN_POINT ( 'NONE',  ( 18.79999999999999005, 8.000000000000000000, 1.212568896937007867 ) ) ;
#70896=DIRECTION ( 'NONE',  ( 0.000000000000000000, 0.000000000000000000, 1.000000000000000000 ) ) ;
#70899=ORIENTED_EDGE ( 'NONE', *, *, #57963, .T. ) ;
#70906=AXIS2_PLACEMENT_3D ( 'NONE', #45240, #222569, #204297 ) ;
#70939=ORIENTED_EDGE ( 'NONE', *, *, #51116, .F. ) ;
#70979=DIRECTION ( 'NONE',  ( 0.000000000000000000, 1.000000000000000000, 0.000000000000000000 ) ) ;
#70994=SPHERICAL_SURFACE ( 'NONE', #239844, 0.1000000000000000056 ) ;
#71006=CIRCLE ( 'NONE', #191820, 0.1000000000000002554 ) ;
#71027=ORIENTED_EDGE ( 'NONE', *, *, #14664, .T. ) ;
#71040=VECTOR ( 'NONE', #243374, 1000.000000000000000 ) ;
#71096=CIRCLE ( 'NONE', #16935, 0.09999999999999939493 ) ;
#71160=PLANE ( 'NONE',  #188437 ) ;
#71198=VERTEX_POINT ( 'NONE', #186110 ) ;
#71238=ADVANCED_FACE ( 'NONE', ( #229092 ), #133830, .T. ) ;
#71247=UNCERTAINTY_MEASURE_WITH_UNIT (LENGTH_MEASURE( 1.000000000000000082E-05 ), #148376, 'distance_accuracy_value', 'NONE');
#71301=DIRECTION ( 'NONE',  ( 1.000000000000000000, 0.000000000000000000, 0.000000000000000000 ) ) ;
#71339=CARTESIAN_POINT ( 'NONE',  ( -18.59999999999999787, -10.80884033489985363, 5.900000000000001243 ) ) ;
#71397=EDGE_LOOP ( 'NONE', ( #183946, #249693, #104069, #49045 ) ) ;
#71398=EDGE_CURVE ( 'NONE', #34286, #79153, #119391, .T. ) ;
#71403=AXIS2_PLACEMENT_3D ( 'NONE', #177009, #238223, #15354 ) ;
#71415=ORIENTED_EDGE ( 'NONE', *, *, #90035, .F. ) ;
#71424=( LENGTH_UNIT ( ) NAMED_UNIT ( * ) SI_UNIT ( .MILLI., .METRE. ) );
#71467=ORIENTED_EDGE ( 'NONE', *, *, #90739, .F. ) ;
#71509=DIRECTION ( 'NONE',  ( 1.000000000000000000, 0.000000000000000000, 0.000000000000000000 ) ) ;
#71538=( BOUNDED_CURVE ( )  B_SPLINE_CURVE ( 3, ( #246154, #209594, #49227, #29702 ),
 .UNSPECIFIED., .F., .F. ) 
 B_SPLINE_CURVE_WITH_KNOTS ( ( 4, 4 ),
 ( 1.570796326794896558, 3.141592653589793116 ),
 .UNSPECIFIED. ) 
 CURVE ( )  GEOMETRIC_REPRESENTATION_ITEM ( )  RATIONAL_B_SPLINE_CURVE ( ( 1.000000000000000000, 0.8047378541243649375, 0.8047378541243649375, 1.000000000000000000 ) ) 
 REPRESENTATION_ITEM ( '' )  );
#71564=CARTESIAN_POINT ( 'NONE',  ( 18.59999999999999787, -9.749999999999996447, 31.50000000000000000 ) ) ;
#71599=EDGE_CURVE ( 'NONE', #209282, #253747, #244270, .T. ) ;
#71635=DIRECTION ( 'NONE',  ( 0.000000000000000000, -0.9856811345164829818, -0.1686199900910294314 ) ) ;
#71645=CARTESIAN_POINT ( 'NONE',  ( -37.88850191057539973, -10.64999999999999325, 31.50000000000000000 ) ) ;
#71654=ORIENTED_EDGE ( 'NONE', *, *, #86685, .F. ) ;
#71700=CARTESIAN_POINT ( 'NONE',  ( -19.99999999999999645, 1.249999999999999334, 21.90000000000000213 ) ) ;
#71727=DIRECTION ( 'NONE',  ( -0.000000000000000000, -1.000000000000000000, 0.000000000000000000 ) ) ;
#71796=DIRECTION ( 'NONE',  ( 0.000000000000000000, 0.000000000000000000, -1.000000000000000000 ) ) ;
#71813=AXIS2_PLACEMENT_3D ( 'NONE', #190645, #195785, #254419 ) ;
#71816=VECTOR ( 'NONE', #115835, 1000.000000000000000 ) ;
#71828=AXIS2_PLACEMENT_3D ( 'NONE', #73846, #153395, #232913 ) ;
#71900=DIRECTION ( 'NONE',  ( 0.000000000000000000, 0.000000000000000000, 1.000000000000000000 ) ) ;
#71927=VERTEX_POINT ( 'NONE', #79939 ) ;
#71941=AXIS2_PLACEMENT_3D ( 'NONE', #96016, #158600, #218518 ) ;
#71969=ORIENTED_EDGE ( 'NONE', *, *, #62322, .T. ) ;
#72002=LINE ( 'NONE', #133248, #89877 ) ;
#72008=ORIENTED_EDGE ( 'NONE', *, *, #190236, .T. ) ;
#72043=ORIENTED_EDGE ( 'NONE', *, *, #206297, .F. ) ;
#72083=DIRECTION ( 'NONE',  ( 0.000000000000000000, 0.000000000000000000, -1.000000000000000000 ) ) ;
#72152=CARTESIAN_POINT ( 'NONE',  ( 20.90000000000000213, -1.885425182446133885, -11.49641995933507843 ) ) ;
#72155=DIRECTION ( 'NONE',  ( 0.000000000000000000, -1.000000000000000000, 6.938893903907270030E-14 ) ) ;
#72184=EDGE_LOOP ( 'NONE', ( #222760, #149009, #199551, #61403 ) ) ;
#72201=AXIS2_PLACEMENT_3D ( 'NONE', #108822, #149267, #110114 ) ;
#72264=ORIENTED_EDGE ( 'NONE', *, *, #77889, .T. ) ;
#72281=ADVANCED_FACE ( 'NONE', ( #187450 ), #145723, .T. ) ;
#72293=ORIENTED_EDGE ( 'NONE', *, *, #246868, .F. ) ;
#72312=CIRCLE ( 'NONE', #47323, 0.09999999999999939493 ) ;
#72315=VECTOR ( 'NONE', #119950, 1000.000000000000000 ) ;
#72337=CIRCLE ( 'NONE', #172329, 0.09999999999999939493 ) ;
#72385=FACE_OUTER_BOUND ( 'NONE', #91259, .T. ) ;
#72409=DIRECTION ( 'NONE',  ( 0.000000000000000000, -0.000000000000000000, 1.000000000000000000 ) ) ;
#72438=CIRCLE ( 'NONE', #93256, 0.09999999999999939493 ) ;
#72453=CARTESIAN_POINT ( 'NONE',  ( 18.59999999999999787, -8.350000000000004974, 10.52591260281975138 ) ) ;
#72464=VECTOR ( 'NONE', #42710, 1000.000000000000000 ) ;
#72479=CARTESIAN_POINT ( 'NONE',  ( -13.40000000000000213, -8.350000000000004974, 19.04142135623731491 ) ) ;
#72523=CYLINDRICAL_SURFACE ( 'NONE', #92032, 0.09999999999999939493 ) ;
#72552=CARTESIAN_POINT ( 'NONE',  ( -19.89999999999999858, 1.350000000000000089, 16.60000000000000142 ) ) ;
#72561=DIRECTION ( 'NONE',  ( 0.000000000000000000, -0.1686199900910313187, 0.9856811345164828708 ) ) ;
#72570=CARTESIAN_POINT ( 'NONE',  ( -20.90000000000000213, 8.000000000000000000, -1.212568896937008089 ) ) ;
#72593=CARTESIAN_POINT ( 'NONE',  ( 18.59999999999999787, -14.35849056603774976, -0.4952830188679671064 ) ) ;
#72669=EDGE_LOOP ( 'NONE', ( #46250, #101909, #234838, #231925 ) ) ;
#72673=EDGE_CURVE ( 'NONE', #26640, #73948, #187152, .T. ) ;
#72676=PLANE ( 'NONE',  #57345 ) ;
#72694=VERTEX_POINT ( 'NONE', #24221 ) ;
#72716=FILL_AREA_STYLE ('',( #171825 ) ) ;
#72738=DIRECTION ( 'NONE',  ( 0.000000000000000000, -0.9856811345164832039, -0.1686199900910280158 ) ) ;
#72798=LINE ( 'NONE', #152332, #59637 ) ;
#72807=ORIENTED_EDGE ( 'NONE', *, *, #76890, .F. ) ;
#72918=ORIENTED_EDGE ( 'NONE', *, *, #195040, .F. ) ;
#72939=AXIS2_PLACEMENT_3D ( 'NONE', #132244, #211793, #129673 ) ;
#72983=ORIENTED_EDGE ( 'NONE', *, *, #165912, .F. ) ;
#73010=ADVANCED_FACE ( 'NONE', ( #121735 ), #99656, .T. ) ;
#73017=DIRECTION ( 'NONE',  ( 1.000000000000000000, 0.000000000000000000, 0.000000000000000000 ) ) ;
#73021=VERTEX_POINT ( 'NONE', #125563 ) ;
#73036=CARTESIAN_POINT ( 'NONE',  ( 18.69999999999999929, -10.80884033489985363, 5.900000000000001243 ) ) ;
#73044=ADVANCED_FACE ( 'NONE', ( #203813 ), #199980, .T. ) ;
#73076=DIRECTION ( 'NONE',  ( 0.000000000000000000, 0.000000000000000000, 1.000000000000000000 ) ) ;
#73088=CARTESIAN_POINT ( 'NONE',  ( -18.79999999999999716, 0.000000000000000000, 0.000000000000000000 ) ) ;
#73096=CARTESIAN_POINT ( 'NONE',  ( 21.00000000000000000, 6.238071963501339745, 11.95857864376269042 ) ) ;
#73113=FACE_OUTER_BOUND ( 'NONE', #102049, .T. ) ;
#73160=ORIENTED_EDGE ( 'NONE', *, *, #16767, .T. ) ;
#73185=EDGE_LOOP ( 'NONE', ( #169174, #70651, #229012, #145686 ) ) ;
#73226=EDGE_CURVE ( 'NONE', #211171, #205125, #107259, .T. ) ;
#73228=CIRCLE ( 'NONE', #19008, 0.09999999999999990841 ) ;
#73240=CYLINDRICAL_SURFACE ( 'NONE', #76923, 5.000000000000004441 ) ;
#73294=ORIENTED_EDGE ( 'NONE', *, *, #229644, .T. ) ;
#73306=VERTEX_POINT ( 'NONE', #221766 ) ;
#73308=EDGE_LOOP ( 'NONE', ( #12824, #67267, #159169, #80672 ) ) ;
#73339=ORIENTED_EDGE ( 'NONE', *, *, #4967, .T. ) ;
#73352=FACE_OUTER_BOUND ( 'NONE', #194796, .T. ) ;
#73354=EDGE_LOOP ( 'NONE', ( #86464, #113260, #52812 ) ) ;
#73371=DIRECTION ( 'NONE',  ( 1.000000000000000000, -0.000000000000000000, -0.000000000000000000 ) ) ;
#73398=DIRECTION ( 'NONE',  ( 0.000000000000000000, -0.000000000000000000, -1.000000000000000000 ) ) ;
#73401=VECTOR ( 'NONE', #17037, 1000.000000000000000 ) ;
#73550=TOROIDAL_SURFACE ( 'NONE', #160844, 0.2000000000000000111, 0.1000000000000000056 ) ;
#73567=DIRECTION ( 'NONE',  ( 0.000000000000000000, 1.000000000000000000, 0.000000000000000000 ) ) ;
#73583=ORIENTED_EDGE ( 'NONE', *, *, #230229, .T. ) ;
#73615=ORIENTED_EDGE ( 'NONE', *, *, #79383, .F. ) ;
#73635=TOROIDAL_SURFACE ( 'NONE', #211160, 0.2000000000000000111, 0.1000000000000000056 ) ;
#73647=DIRECTION ( 'NONE',  ( 0.000000000000000000, 0.000000000000000000, 1.000000000000000000 ) ) ;
#73672=DIRECTION ( 'NONE',  ( 0.000000000000000000, 0.000000000000000000, -1.000000000000000000 ) ) ;
#73680=EDGE_CURVE ( 'NONE', #37930, #56204, #44143, .T. ) ;
#73692=EDGE_LOOP ( 'NONE', ( #168265, #12945, #736, #66213 ) ) ;
#73752=CARTESIAN_POINT ( 'NONE',  ( 18.79999999999999716, 5.488301202077012775, 16.50000000000000000 ) ) ;
#73764=( BOUNDED_SURFACE ( )  B_SPLINE_SURFACE ( 3, 2, ( 
 ( #176987, #218629, #79113 ),
 ( #2150, #158706, #238198 ),
 ( #59536, #82948, #225040 ),
 ( #205490, #102512, #84209 ) ),
 .UNSPECIFIED., .F., .F., .F. ) 
 B_SPLINE_SURFACE_WITH_KNOTS ( ( 4, 4 ),
 ( 3, 3 ),
 ( 4.712388980384689674, 6.283185307179586232 ),
 ( 0.000000000000000000, 1.000000000000000000 ),
 .UNSPECIFIED. ) 
 GEOMETRIC_REPRESENTATION_ITEM ( )  RATIONAL_B_SPLINE_SURFACE ( (
 ( 1.000000000000000000, 0.7071067811865444641, 1.000000000000000000),
 ( 1.000000000000000000, 0.7389971855006018941, 1.000000000000000000),
 ( 1.000000000000000000, 0.7651312202474049862, 1.000000000000000000),
 ( 1.000000000000000000, 0.7644017236018784134, 1.000000000000000000) ) ) 
 REPRESENTATION_ITEM ( '' )  SURFACE ( )  );
#73792=CARTESIAN_POINT ( 'NONE',  ( -18.69999999999999929, -11.65000000000000036, -15.00000000000000000 ) ) ;
#73809=CARTESIAN_POINT ( 'NONE',  ( 18.79999999999999716, 7.900000000000000355, -1.212568896937008089 ) ) ;
#73812=AXIS2_PLACEMENT_3D ( 'NONE', #25884, #148387, #105362 ) ;
#73833=DIRECTION ( 'NONE',  ( 2.895190717381441586E-16, -0.1335171055202867274, 0.9910465087640865089 ) ) ;
#73836=CARTESIAN_POINT ( 'NONE',  ( 18.69999999999999929, -14.27107483842559432, -0.5438473119858313609 ) ) ;
#73846=CARTESIAN_POINT ( 'NONE',  ( 18.79999999999999716, 1.212568896937007645, -8.000000000000000000 ) ) ;
#73865=DIRECTION ( 'NONE',  ( -3.469446951953635015E-14, 1.000000000000000000, 0.000000000000000000 ) ) ;
#73883=ORIENTED_EDGE ( 'NONE', *, *, #95749, .T. ) ;
#73888=ORIENTED_EDGE ( 'NONE', *, *, #139886, .T. ) ;
#73901=LINE ( 'NONE', #232965, #105377 ) ;
#73948=VERTEX_POINT ( 'NONE', #159607 ) ;
#74003=AXIS2_PLACEMENT_3D ( 'NONE', #255341, #214981, #117180 ) ;
#74023=LINE ( 'NONE', #137788, #64864 ) ;
#74075=ORIENTED_EDGE ( 'NONE', *, *, #151681, .F. ) ;
#74082=ORIENTED_EDGE ( 'NONE', *, *, #48142, .T. ) ;
#74102=DIRECTION ( 'NONE',  ( 0.000000000000000000, 0.000000000000000000, -1.000000000000000000 ) ) ;
#74114=DIRECTION ( 'NONE',  ( 0.000000000000000000, 0.000000000000000000, -1.000000000000000000 ) ) ;
#74126=FACE_OUTER_BOUND ( 'NONE', #118827, .T. ) ;
#74135=DIRECTION ( 'NONE',  ( 2.168404344971008868E-16, 0.000000000000000000, 1.000000000000000000 ) ) ;
#74139=EDGE_CURVE ( 'NONE', #72694, #184776, #107619, .T. ) ;
#74142=LINE ( 'NONE', #115803, #20859 ) ;
#74159=CLOSED_SHELL ( 'NONE', ( #94218, #62465, #47386, #99100, #213142, #254130, #117392, #86339, #49445, #46607, #146865, #111811, #248673, #92957, #87688, #38455, #56909, #20475, #248974, #42179, #238951, #251575, #239058, #57618, #87054, #124520, #147134, #10876, #178103, #187078, #53979, #180277, #81436, #8671, #15480, #117195, #203207, #19609, #47706, #206529, #62777, #211083, #11497, #245189, #8680, #103172, #159580, #155666, #241050, #223531, #107720, #252718, #243128, #19801, #188620, #66082, #76722, #41, #1654, #34112, #43697, #68301, #84406, #30154, #84419, #111716, #53209, #165302, #33829, #257919, #90752, #197376, #90397, #5188, #122658, #224102, #128441, #106426, #38299, #143878, #175190, #115957, #31171, #241697, #57590, #18078, #36959, #94571, #214026, #16443, #179700, #206314, #45910, #123519, #219630, #200550, #136581, #43311, #217156, #202370, #211654, #166819, #183, #62264, #190506, #68618, #109026, #37256, #141285, #250334, #154704, #96617, #171761, #20002, #159192, #21656, #148560, #31178, #13160, #220755, #170083, #253042, #207171, #154268, #211053, #174047, #257600, #179895, #216507, #164476, #80796, #193836, #1461, #252965, #22928, #234852, #171957, #55098, #155773, #89987, #209077, #244291, #173408, #88454, #240625, #46885, #219067, #200978, #251026, #237764, #100790, #9119, #32935, #48792, #245145, #123813, #253806, #195979, #101160, #4370, #234431, #102105, #84654, #255607, #113887, #226508, #1778, #207399, #135297, #77996, #40184, #88982, #193446, #89173, #206546, #246249, #241885, #256052, #230326, #228145, #142634, #93782, #124069, #253958, #111605, #9751, #88994, #186969, #233690, #63621, #22573, #30340, #144904, #18756, #116753, #186250, #236294, #79149, #222503, #119852, #85301, #73010, #70640, #16353, #152295, #195344, #242804, #237845, #38514, #106971, #218210, #131771, #67056, #72281, #25719, #144010, #212266, #172633, #197925, #54814, #186819, #25823, #133667, #57669, #218286, #236616, #147449, #47068, #41717, #227342, #151141, #64007, #66390, #122446, #175180, #339, #80567, #166673, #76529, #114324, #25525, #53560, #173757, #145933, #63458, #84017, #69389, #192058, #81747, #196469, #91341, #150968, #149574, #18539, #26190, #50794, #92326, #232793, #125541, #44672, #214374, #148622, #2114, #143285, #190090, #218395, #126833, #200403, #151770, #196371, #129970, #113263, #56435, #141168, #140562, #99243, #202389, #206494, #73044, #155921, #103825, #249541, #236848, #61180, #132073, #1051, #16155, #138651, #30865, #230690, #139926, #38200, #232754, #255294, #69823, #78321, #17116, #18783, #91340, #143208, #32268, #121435, #211134, #197850, #196817, #212696, #36416, #71238, #97290, #189812, #156181, #21894, #99254, #166061, #40324, #124734, #108633, #92428, #143960, #163225, #162801, #254985, #36532, #193683, #119040, #239316, #120377, #83105, #30239, #44185, #122485, #178403, #35231, #163001, #213091, #59579, #122114, #10267, #22514, #77563, #141583, #225177, #174703, #176625, #60423, #48027, #4080, #144506, #132413, #187231, #116301, #13321, #1346, #12676, #123523, #86947, #218777, #48867, #155553, #225649, #239244 ) ) ;
#74238=DIRECTION ( 'NONE',  ( -1.000000000000000000, 0.000000000000000000, 0.000000000000000000 ) ) ;
#74299=CARTESIAN_POINT ( 'NONE',  ( 18.69999999999999929, 1.212568896937007645, -7.800000000000000711 ) ) ;
#74306=ORIENTED_EDGE ( 'NONE', *, *, #38623, .T. ) ;
#74334=DIRECTION ( 'NONE',  ( -0.000000000000000000, 0.000000000000000000, -1.000000000000000000 ) ) ;
#74359=DIRECTION ( 'NONE',  ( 1.000000000000000000, 0.000000000000000000, -0.000000000000000000 ) ) ;
#74418=CIRCLE ( 'NONE', #70317, 0.09999999999999939493 ) ;
#74431=EDGE_CURVE ( 'NONE', #83776, #245477, #211882, .T. ) ;
#74508=CARTESIAN_POINT ( 'NONE',  ( 11.60000000000000142, -11.65000000000000036, 17.60000000000000497 ) ) ;
#74539=FACE_OUTER_BOUND ( 'NONE', #226683, .T. ) ;
#74542=EDGE_CURVE ( 'NONE', #208877, #7521, #111932, .T. ) ;
#74551=DIRECTION ( 'NONE',  ( 0.000000000000000000, 0.000000000000000000, 1.000000000000000000 ) ) ;
#74562=DIRECTION ( 'NONE',  ( 0.000000000000000000, 0.000000000000000000, -1.000000000000000000 ) ) ;
#74603=AXIS2_PLACEMENT_3D ( 'NONE', #131700, #108294, #88692 ) ;
#74654=ORIENTED_EDGE ( 'NONE', *, *, #52119, .F. ) ;
#74656=CARTESIAN_POINT ( 'NONE',  ( -22.84999999999999787, 0.000000000000000000, 0.000000000000000000 ) ) ;
#74672=DIRECTION ( 'NONE',  ( -1.000000000000000000, 0.000000000000000000, -0.000000000000000000 ) ) ;
#74686=ORIENTED_EDGE ( 'NONE', *, *, #11538, .T. ) ;
#74744=CARTESIAN_POINT ( 'NONE',  ( 0.000000000000000000, 1.350000000000000089, 16.60000000000000142 ) ) ;
#74790=PLANE ( 'NONE',  #223499 ) ;
#74836=CARTESIAN_POINT ( 'NONE',  ( 18.69999999999999929, 4.513204987021264714, 22.10000000000000142 ) ) ;
#74889=ORIENTED_EDGE ( 'NONE', *, *, #114145, .F. ) ;
#74901=CIRCLE ( 'NONE', #241472, 0.09999999999999939493 ) ;
#74907=AXIS2_PLACEMENT_3D ( 'NONE', #116710, #175431, #155865 ) ;
#74920=ORIENTED_EDGE ( 'NONE', *, *, #20023, .F. ) ;
#74921=EDGE_CURVE ( 'NONE', #150529, #60954, #249659, .T. ) ;
#74968=VERTEX_POINT ( 'NONE', #226793 ) ;
#74973=ORIENTED_EDGE ( 'NONE', *, *, #117758, .F. ) ;
#74986=DIRECTION ( 'NONE',  ( 0.000000000000000000, 0.000000000000000000, 1.000000000000000000 ) ) ;
#74988=CARTESIAN_POINT ( 'NONE',  ( -22.94999999999999929, 6.223900101154157483, 12.09999999999999964 ) ) ;
#75005=EDGE_LOOP ( 'NONE', ( #188142, #36581, #29742, #255969 ) ) ;
#75031=EDGE_CURVE ( 'NONE', #78593, #20074, #87143, .T. ) ;
#75066=CARTESIAN_POINT ( 'NONE',  ( -18.79999999999999716, 7.799999999999999822, -15.00000000000000000 ) ) ;
#75141=FACE_OUTER_BOUND ( 'NONE', #16508, .T. ) ;
#75148=EDGE_CURVE ( 'NONE', #217909, #106580, #95697, .T. ) ;
#75200=VECTOR ( 'NONE', #206163, 1000.000000000000000 ) ;
#75205=VERTEX_POINT ( 'NONE', #19304 ) ;
#75222=CIRCLE ( 'NONE', #50231, 2.600000000000000089 ) ;
#75242=CARTESIAN_POINT ( 'NONE',  ( -18.79999999999999716, 6.644425182197214674, 9.641788261573355001 ) ) ;
#75310=EDGE_CURVE ( 'NONE', #211037, #18932, #27037, .T. ) ;
#75317=DIRECTION ( 'NONE',  ( 1.000000000000000000, 0.000000000000000000, 0.000000000000000000 ) ) ;
#75320=CARTESIAN_POINT ( 'NONE',  ( 20.90000000000000213, 7.973296578895943121, 1.410778198689825347 ) ) ;
#75369=ORIENTED_EDGE ( 'NONE', *, *, #14671, .F. ) ;
#75404=VERTEX_POINT ( 'NONE', #94345 ) ;
#75428=CARTESIAN_POINT ( 'NONE',  ( -18.69999999999999929, -8.250000000000005329, 16.39999999999999858 ) ) ;
#75429=CARTESIAN_POINT ( 'NONE',  ( 22.19999999999999929, -1.467286812112899463, 28.00000000000000000 ) ) ;
#75451=VERTEX_POINT ( 'NONE', #74836 ) ;
#75476=CARTESIAN_POINT ( 'NONE',  ( -19.89999999999999858, 1.350000000000000089, 21.90000000000000213 ) ) ;
#75504=DIRECTION ( 'NONE',  ( 0.000000000000000000, 0.000000000000000000, 1.000000000000000000 ) ) ;
#75607=EDGE_CURVE ( 'NONE', #248699, #89072, #112477, .T. ) ;
#75610=EDGE_LOOP ( 'NONE', ( #24572, #115232, #139383, #165844 ) ) ;
#75644=DIRECTION ( 'NONE',  ( -1.000000000000000000, 0.000000000000000000, 0.000000000000000000 ) ) ;
#75657=ORIENTED_EDGE ( 'NONE', *, *, #10294, .F. ) ;
#75673=ORIENTED_EDGE ( 'NONE', *, *, #68146, .T. ) ;
#75712=DIRECTION ( 'NONE',  ( -1.000000000000000000, 0.000000000000000000, 0.000000000000000000 ) ) ;
#75786=DIRECTION ( 'NONE',  ( -1.000000000000000000, 0.000000000000000000, 0.000000000000000000 ) ) ;
#75809=VERTEX_POINT ( 'NONE', #114912 ) ;
#75855=CARTESIAN_POINT ( 'NONE',  ( 18.79999999999999716, 7.900000000000000355, 1.212568896937007867 ) ) ;
#75865=DIRECTION ( 'NONE',  ( -0.000000000000000000, 1.000000000000000000, -0.000000000000000000 ) ) ;
#75891=ORIENTED_EDGE ( 'NONE', *, *, #42817, .T. ) ;
#75902=EDGE_CURVE ( 'NONE', #92448, #101761, #137743, .T. ) ;
#75904=CIRCLE ( 'NONE', #230015, 0.1999999999999996503 ) ;
#75948=CARTESIAN_POINT ( 'NONE',  ( 0.000000000000000000, 0.000000000000000000, 33.00000000000000000 ) ) ;
#75962=ORIENTED_EDGE ( 'NONE', *, *, #52119, .T. ) ;
#76000=CIRCLE ( 'NONE', #51011, 0.09999999999999963085 ) ;
#76012=ORIENTED_EDGE ( 'NONE', *, *, #216199, .F. ) ;
#76024=ORIENTED_EDGE ( 'NONE', *, *, #23802, .F. ) ;
#76066=EDGE_CURVE ( 'NONE', #186207, #245477, #208, .T. ) ;
#76067=VECTOR ( 'NONE', #173197, 1000.000000000000000 ) ;
#76102=CARTESIAN_POINT ( 'NONE',  ( -18.79999999999999716, 0.000000000000000000, 32.89999999999999858 ) ) ;
#76191=CARTESIAN_POINT ( 'NONE',  ( -20.90000000000000213, 6.841561409100513025, 9.675512259591560138 ) ) ;
#76259=VECTOR ( 'NONE', #55573, 1000.000000000000000 ) ;
#76261=FACE_OUTER_BOUND ( 'NONE', #41558, .T. ) ;
#76298=AXIS2_PLACEMENT_3D ( 'NONE', #198835, #119310, #137560 ) ;
#76334=CARTESIAN_POINT ( 'NONE',  ( -18.59999999999999787, -9.749999999999996447, 31.39999999999999858 ) ) ;
#76341=DIRECTION ( 'NONE',  ( 0.000000000000000000, 0.000000000000000000, -1.000000000000000000 ) ) ;
#76402=EDGE_CURVE ( 'NONE', #92927, #249092, #45326, .T. ) ;
#76419=ORIENTED_EDGE ( 'NONE', *, *, #18943, .T. ) ;
#76447=TOROIDAL_SURFACE ( 'NONE', #230600, 11.65000000000000036, 0.1000000000000000056 ) ;
#76457=PLANE ( 'NONE',  #71941 ) ;
#76465=ORIENTED_EDGE ( 'NONE', *, *, #76066, .T. ) ;
#76499=LINE ( 'NONE', #88675, #77331 ) ;
#76505=DIRECTION ( 'NONE',  ( -1.000000000000000000, -0.000000000000000000, 0.000000000000000000 ) ) ;
#76529=ADVANCED_FACE ( 'NONE', ( #50433 ), #230380, .T. ) ;
#76531=VERTEX_POINT ( 'NONE', #191288 ) ;
#76573=AXIS2_PLACEMENT_3D ( 'NONE', #242415, #63792, #122496 ) ;
#76607=DIRECTION ( 'NONE',  ( -1.000000000000000000, -0.000000000000000000, -0.000000000000000000 ) ) ;
#76620=DIRECTION ( 'NONE',  ( 0.000000000000000000, 0.000000000000000000, 1.000000000000000000 ) ) ;
#76623=DIRECTION ( 'NONE',  ( -0.000000000000000000, 0.000000000000000000, 1.000000000000000000 ) ) ;
#76643=ORIENTED_EDGE ( 'NONE', *, *, #17750, .T. ) ;
#76665=DIRECTION ( 'NONE',  ( -1.000000000000000000, 8.673617379884087537E-15, 0.000000000000000000 ) ) ;
#76668=ORIENTED_EDGE ( 'NONE', *, *, #209794, .T. ) ;
#76671=DIRECTION ( 'NONE',  ( -0.000000000000000000, 0.000000000000000000, -1.000000000000000000 ) ) ;
#76706=ORIENTED_EDGE ( 'NONE', *, *, #72673, .T. ) ;
#76722=ADVANCED_FACE ( 'NONE', ( #219793 ), #41195, .T. ) ;
#76726=VECTOR ( 'NONE', #74672, 1000.000000000000000 ) ;
#76759=VERTEX_POINT ( 'NONE', #245794 ) ;
#76761=ORIENTED_EDGE ( 'NONE', *, *, #205370, .T. ) ;
#76773=AXIS2_PLACEMENT_3D ( 'NONE', #129904, #30847, #46511 ) ;
#76798=ORIENTED_EDGE ( 'NONE', *, *, #23246, .F. ) ;
#76850=PLANE ( 'NONE',  #78137 ) ;
#76869=CARTESIAN_POINT ( 'NONE',  ( -18.59999999999999787, -9.849999999999994316, 30.00000000000000000 ) ) ;
#76870=DIRECTION ( 'NONE',  ( 0.000000000000000000, 0.000000000000000000, -1.000000000000000000 ) ) ;
#76873=DIRECTION ( 'NONE',  ( -4.336808689942017736E-16, 0.000000000000000000, -1.000000000000000000 ) ) ;
#76883=AXIS2_PLACEMENT_3D ( 'NONE', #51610, #132472, #210723 ) ;
#76890=EDGE_CURVE ( 'NONE', #62919, #212664, #192148, .T. ) ;
#76894=VECTOR ( 'NONE', #14197, 1000.000000000000000 ) ;
#76913=DIRECTION ( 'NONE',  ( 0.000000000000000000, 0.9868171638914230437, 0.1618390714546045217 ) ) ;
#76923=AXIS2_PLACEMENT_3D ( 'NONE', #251833, #155343, #152774 ) ;
#76994=CARTESIAN_POINT ( 'NONE',  ( 20.90000000000000213, 0.000000000000000000, 0.000000000000000000 ) ) ;
#76998=CARTESIAN_POINT ( 'NONE',  ( 18.79999999999999716, 11.49641995933507843, -1.885425182446135661 ) ) ;
#77037=DIRECTION ( 'NONE',  ( -1.462545276649423285E-15, 0.1686199900910279881, -0.9856811345164833149 ) ) ;
#77051=ORIENTED_EDGE ( 'NONE', *, *, #138812, .F. ) ;
#77088=VERTEX_POINT ( 'NONE', #168240 ) ;
#77093=DIRECTION ( 'NONE',  ( 1.000000000000000000, 0.000000000000000000, 0.000000000000000000 ) ) ;
#77100=CIRCLE ( 'NONE', #227122, 0.1999999999999987899 ) ;
#77112=ORIENTED_EDGE ( 'NONE', *, *, #5812, .T. ) ;
#77125=EDGE_LOOP ( 'NONE', ( #23852, #70271, #65491, #105217 ) ) ;
#77177=CARTESIAN_POINT ( 'NONE',  ( -19.89999999999999858, 11.61130914238355771, 21.90000000000000213 ) ) ;
#77186=CARTESIAN_POINT ( 'NONE',  ( -20.90000000000000213, -11.75000000000000178, 0.000000000000000000 ) ) ;
#77213=DIRECTION ( 'NONE',  ( 0.000000000000000000, -0.000000000000000000, 1.000000000000000000 ) ) ;
#77296=ORIENTED_EDGE ( 'NONE', *, *, #14663, .T. ) ;
#77320=ORIENTED_EDGE ( 'NONE', *, *, #249884, .T. ) ;
#77331=VECTOR ( 'NONE', #127842, 1000.000000000000227 ) ;
#77344=EDGE_CURVE ( 'NONE', #249092, #41516, #121229, .T. ) ;
#77355=CIRCLE ( 'NONE', #10746, 0.09999999999999939493 ) ;
#77389=CARTESIAN_POINT ( 'NONE',  ( -22.84999999999999787, 0.000000000000000000, -4.000000000000000000 ) ) ;
#77416=DIRECTION ( 'NONE',  ( 2.489438768765008884E-17, 0.1686199900910312910, -0.9856811345164826488 ) ) ;
#77431=CIRCLE ( 'NONE', #185786, 3.970710678118657189 ) ;
#77526=DIRECTION ( 'NONE',  ( 1.000000000000000000, 0.000000000000000000, 0.000000000000000000 ) ) ;
#77529=ORIENTED_EDGE ( 'NONE', *, *, #231013, .T. ) ;
#77534=CARTESIAN_POINT ( 'NONE',  ( -0.8999999999999994671, -8.350000000000004974, 30.04142135623731136 ) ) ;
#77554=CARTESIAN_POINT ( 'NONE',  ( 6.100000000000000533, -11.75000000000000000, 13.90000000000000213 ) ) ;
#77563=ADVANCED_FACE ( 'NONE', ( #145740 ), #62925, .T. ) ;
#77678=CARTESIAN_POINT ( 'NONE',  ( -18.69999999999999929, -10.84999999999999076, 31.59999999999999787 ) ) ;
#77693=DIRECTION ( 'NONE',  ( 0.000000000000000000, -1.000000000000000000, 0.000000000000000000 ) ) ;
#77701=AXIS2_PLACEMENT_3D ( 'NONE', #120759, #256316, #136404 ) ;
#77782=AXIS2_PLACEMENT_3D ( 'NONE', #155115, #138065, #61109 ) ;
#77799=CARTESIAN_POINT ( 'NONE',  ( -21.00000000000000000, 6.238071963501339745, 11.95857864376269575 ) ) ;
#77845=PLANE ( 'NONE',  #5299 ) ;
#77869=CARTESIAN_POINT ( 'NONE',  ( -18.79999999999999716, 11.61130914238355771, 22.00000000000000355 ) ) ;
#77878=FACE_OUTER_BOUND ( 'NONE', #85668, .T. ) ;
#77884=CARTESIAN_POINT ( 'NONE',  ( 21.00000000000000000, -1.212568896937008089, -7.800000000000000711 ) ) ;
#77889=EDGE_CURVE ( 'NONE', #247436, #139556, #38632, .T. ) ;
#77898=DIRECTION ( 'NONE',  ( -0.000000000000000000, 1.000000000000000000, -0.000000000000000000 ) ) ;
#77926=ORIENTED_EDGE ( 'NONE', *, *, #114824, .F. ) ;
#77950=ORIENTED_EDGE ( 'NONE', *, *, #91517, .T. ) ;
#77996=ADVANCED_FACE ( 'NONE', ( #236402 ), #57752, .F. ) ;
#78001=CARTESIAN_POINT ( 'NONE',  ( -21.10000000000000142, 0.000000000000000000, 0.000000000000000000 ) ) ;
#78017=VECTOR ( 'NONE', #31335, 1000.000000000000000 ) ;
#78034=DIRECTION ( 'NONE',  ( 0.000000000000000000, 0.000000000000000000, -1.000000000000000000 ) ) ;
#78044=ORIENTED_EDGE ( 'NONE', *, *, #249589, .T. ) ;
#78061=DIRECTION ( 'NONE',  ( 1.000000000000000000, -0.000000000000000000, 0.000000000000000000 ) ) ;
#78066=DIRECTION ( 'NONE',  ( 1.000000000000000000, 0.000000000000000000, -0.000000000000000000 ) ) ;
#78080=DIRECTION ( 'NONE',  ( 1.000000000000000000, -0.000000000000000000, -0.000000000000000000 ) ) ;
#78117=EDGE_LOOP ( 'NONE', ( #115224, #110717, #201823 ) ) ;
#78121=CARTESIAN_POINT ( 'NONE',  ( -18.79999999999999716, 5.488301202077012775, 16.40000000000000213 ) ) ;
#78130=EDGE_CURVE ( 'NONE', #94336, #105678, #189578, .T. ) ;
#78137=AXIS2_PLACEMENT_3D ( 'NONE', #118574, #74334, #234650 ) ;
#78208=ORIENTED_EDGE ( 'NONE', *, *, #225642, .T. ) ;
#78211=CARTESIAN_POINT ( 'NONE',  ( 5.899999999999996803, -11.34999999999999964, 13.90000000000000213 ) ) ;
#78215=CARTESIAN_POINT ( 'NONE',  ( -21.00000000000000000, 7.800000000000000711, 1.212568896937007867 ) ) ;
#78229=AXIS2_PLACEMENT_3D ( 'NONE', #59131, #158310, #138668 ) ;
#78243=CIRCLE ( 'NONE', #119985, 0.1000000000000028644 ) ;
#78264=PLANE ( 'NONE',  #120006 ) ;
#78271=ORIENTED_EDGE ( 'NONE', *, *, #122979, .F. ) ;
#78275=VECTOR ( 'NONE', #174476, 1000.000000000000227 ) ;
#78305=CARTESIAN_POINT ( 'NONE',  ( -18.79999999999999716, -11.75000000000000178, 0.000000000000000000 ) ) ;
#78321=ADVANCED_FACE ( 'NONE', ( #129447 ), #30362, .T. ) ;
#78326=DIRECTION ( 'NONE',  ( 0.000000000000000000, 0.000000000000000000, 1.000000000000000000 ) ) ;
#78355=ORIENTED_EDGE ( 'NONE', *, *, #215515, .T. ) ;
#78378=ORIENTED_EDGE ( 'NONE', *, *, #106959, .T. ) ;
#78387=VERTEX_POINT ( 'NONE', #169908 ) ;
#78391=DIRECTION ( 'NONE',  ( 0.000000000000000000, 0.000000000000000000, -1.000000000000000000 ) ) ;
#78394=VERTEX_POINT ( 'NONE', #234976 ) ;
#78413=VECTOR ( 'NONE', #248086, 1000.000000000000000 ) ;
#78424=AXIS2_PLACEMENT_3D ( 'NONE', #191759, #10528, #208737 ) ;
#78436=DIRECTION ( 'NONE',  ( -0.000000000000000000, 0.1686199900910312910, -0.9856811345164826488 ) ) ;
#78486=ORIENTED_EDGE ( 'NONE', *, *, #194309, .T. ) ;
#78489=PLANE ( 'NONE',  #56905 ) ;
#78492=DIRECTION ( 'NONE',  ( 0.000000000000000000, 1.000000000000000000, -0.000000000000000000 ) ) ;
#78501=ORIENTED_EDGE ( 'NONE', *, *, #94090, .F. ) ;
#78557=VECTOR ( 'NONE', #245227, 1000.000000000000000 ) ;
#78593=VERTEX_POINT ( 'NONE', #100555 ) ;
#78635=ORIENTED_EDGE ( 'NONE', *, *, #202166, .T. ) ;
#78741=LINE ( 'NONE', #158336, #186845 ) ;
#78816=PLANE ( 'NONE',  #179396 ) ;
#78830=ORIENTED_EDGE ( 'NONE', *, *, #49497, .T. ) ;
#78862=CARTESIAN_POINT ( 'NONE',  ( 18.79999999999999716, -1.885425182446133885, -11.49641995933507843 ) ) ;
#78877=AXIS2_PLACEMENT_3D ( 'NONE', #25050, #8040, #147538 ) ;
#78892=AXIS2_PLACEMENT_3D ( 'NONE', #136146, #16265, #39681 ) ;
#78894=ORIENTED_EDGE ( 'NONE', *, *, #70054, .F. ) ;
#78951=ORIENTED_EDGE ( 'NONE', *, *, #11315, .T. ) ;
#79030=CARTESIAN_POINT ( 'NONE',  ( -20.90000000000000213, 7.973296578895943121, -1.410778198689825347 ) ) ;
#79039=ORIENTED_EDGE ( 'NONE', *, *, #165458, .T. ) ;
#79049=ORIENTED_EDGE ( 'NONE', *, *, #21163, .T. ) ;
#79074=LINE ( 'NONE', #16582, #52614 ) ;
#79081=EDGE_LOOP ( 'NONE', ( #128986, #210330, #131356, #45809, #249954, #84407, #228503 ) ) ;
#79088=DIRECTION ( 'NONE',  ( 0.000000000000000000, 0.000000000000000000, 1.000000000000000000 ) ) ;
#79113=CARTESIAN_POINT ( 'NONE',  ( 20.00000000000000355, 5.454087299794354138, 16.60000000000000142 ) ) ;
#79145=LINE ( 'NONE', #38764, #114837 ) ;
#79149=ADVANCED_FACE ( 'NONE', ( #205464 ), #102460, .T. ) ;
#79153=VERTEX_POINT ( 'NONE', #146754 ) ;
#79154=DIRECTION ( 'NONE',  ( 1.000000000000000000, 0.000000000000000000, 0.000000000000000000 ) ) ;
#79242=DIRECTION ( 'NONE',  ( 1.000000000000000000, -0.000000000000000000, -0.000000000000000000 ) ) ;
#79243=AXIS2_PLACEMENT_3D ( 'NONE', #97159, #94633, #76341 ) ;
#79286=VERTEX_POINT ( 'NONE', #81334 ) ;
#79289=DIRECTION ( 'NONE',  ( 0.000000000000000000, 0.000000000000000000, 1.000000000000000000 ) ) ;
#79294=LINE ( 'NONE', #121043, #59848 ) ;
#79339=ORIENTED_EDGE ( 'NONE', *, *, #224630, .F. ) ;
#79364=CARTESIAN_POINT ( 'NONE',  ( -18.79999999999999716, -1.885425182446133885, -11.49641995933507843 ) ) ;
#79378=ORIENTED_EDGE ( 'NONE', *, *, #76890, .T. ) ;
#79383=EDGE_CURVE ( 'NONE', #5568, #63710, #252506, .T. ) ;
#79393=DIRECTION ( 'NONE',  ( -0.000000000000000000, -0.1686199900910312910, 0.9856811345164826488 ) ) ;
#79419=ORIENTED_EDGE ( 'NONE', *, *, #110202, .F. ) ;
#79429=DIRECTION ( 'NONE',  ( 1.000000000000000000, 0.000000000000000000, 0.000000000000000000 ) ) ;
#79475=EDGE_CURVE ( 'NONE', #94336, #16688, #48509, .T. ) ;
#79512=DIRECTION ( 'NONE',  ( -1.000000000000000000, 0.000000000000000000, 0.000000000000000000 ) ) ;
#79574=CARTESIAN_POINT ( 'NONE',  ( 18.59999999999999787, -10.74999999999999289, 31.59999999999999787 ) ) ;
#79587=EDGE_CURVE ( 'NONE', #58261, #245971, #254536, .T. ) ;
#79594=ORIENTED_EDGE ( 'NONE', *, *, #236214, .F. ) ;
#79700=EDGE_LOOP ( 'NONE', ( #114026, #179268, #79594 ) ) ;
#79713=CARTESIAN_POINT ( 'NONE',  ( 20.00000000000000355, 4.547418889303922462, 21.90000000000000213 ) ) ;
#79788=CARTESIAN_POINT ( 'NONE',  ( 18.79999999999999716, 0.000000000000000000, 32.89999999999999858 ) ) ;
#79797=CYLINDRICAL_SURFACE ( 'NONE', #219663, 0.09999999999999939493 ) ;
#79817=CARTESIAN_POINT ( 'NONE',  ( -22.19999999999999929, -11.75000000000000000, 32.89999999999999858 ) ) ;
#79820=DIRECTION ( 'NONE',  ( 0.000000000000000000, -1.000000000000000000, 0.000000000000000000 ) ) ;
#79822=ORIENTED_EDGE ( 'NONE', *, *, #103394, .F. ) ;
#79856=DIRECTION ( 'NONE',  ( 0.000000000000000000, 0.000000000000000000, -1.000000000000000000 ) ) ;
#79870=AXIS2_PLACEMENT_3D ( 'NONE', #129443, #196788, #194265 ) ;
#79874=ORIENTED_EDGE ( 'NONE', *, *, #202378, .F. ) ;
#79892=DIRECTION ( 'NONE',  ( 1.000000000000000000, 0.000000000000000000, 0.000000000000000000 ) ) ;
#79909=DIRECTION ( 'NONE',  ( 0.000000000000000000, 4.336808689942044242E-14, 1.000000000000000000 ) ) ;
#79910=ORIENTED_EDGE ( 'NONE', *, *, #63567, .F. ) ;
#79939=CARTESIAN_POINT ( 'NONE',  ( -11.60000000000000320, -11.65000000000000036, 12.40000000000000391 ) ) ;
#79944=VERTEX_POINT ( 'NONE', #254242 ) ;
#79974=FACE_OUTER_BOUND ( 'NONE', #215229, .T. ) ;
#79985=DIRECTION ( 'NONE',  ( -1.000000000000000000, 0.000000000000000000, 0.000000000000000000 ) ) ;
#80019=DIRECTION ( 'NONE',  ( 0.000000000000000000, 0.000000000000000000, 1.000000000000000000 ) ) ;
#80042=DIRECTION ( 'NONE',  ( 0.000000000000000000, 0.000000000000000000, 1.000000000000000000 ) ) ;
#80043=DIRECTION ( 'NONE',  ( 1.000000000000000000, 0.000000000000000000, 0.000000000000000000 ) ) ;
#80094=FACE_OUTER_BOUND ( 'NONE', #36527, .T. ) ;
#80101=FACE_OUTER_BOUND ( 'NONE', #243251, .T. ) ;
#80118=CIRCLE ( 'NONE', #121872, 0.09999999999999939493 ) ;
#80150=CARTESIAN_POINT ( 'NONE',  ( 5.899999999999996803, -11.75000000000000000, 14.10000000000000142 ) ) ;
#80200=ORIENTED_EDGE ( 'NONE', *, *, #218609, .F. ) ;
#80206=CYLINDRICAL_SURFACE ( 'NONE', #68605, 0.09999999999999939493 ) ;
#80207=CIRCLE ( 'NONE', #117837, 2.700000000000001066 ) ;
#80216=EDGE_LOOP ( 'NONE', ( #49140, #201756, #194485, #234925 ) ) ;
#80228=FACE_OUTER_BOUND ( 'NONE', #56937, .T. ) ;
#80245=ORIENTED_EDGE ( 'NONE', *, *, #42319, .F. ) ;
#80274=DIRECTION ( 'NONE',  ( 0.000000000000000000, 0.000000000000000000, 1.000000000000000000 ) ) ;
#80290=VECTOR ( 'NONE', #189972, 1000.000000000000114 ) ;
#80296=EDGE_CURVE ( 'NONE', #190676, #176903, #34947, .T. ) ;
#80304=ORIENTED_EDGE ( 'NONE', *, *, #58392, .F. ) ;
#80306=ORIENTED_EDGE ( 'NONE', *, *, #191204, .F. ) ;
#80325=CARTESIAN_POINT ( 'NONE',  ( -19.99999999999999645, 1.350000000000000089, 16.50000000000000000 ) ) ;
#80368=ORIENTED_EDGE ( 'NONE', *, *, #60162, .F. ) ;
#80386=FACE_OUTER_BOUND ( 'NONE', #53924, .T. ) ;
#80485=DIRECTION ( 'NONE',  ( 8.673617379884087537E-15, 1.000000000000000000, 0.000000000000000000 ) ) ;
#80497=DIRECTION ( 'NONE',  ( 0.000000000000000000, 0.000000000000000000, 1.000000000000000000 ) ) ;
#80545=PLANE ( 'NONE',  #171184 ) ;
#80550=FACE_OUTER_BOUND ( 'NONE', #203261, .T. ) ;
#80567=ADVANCED_FACE ( 'NONE', ( #47727 ), #28220, .T. ) ;
#80569=FACE_OUTER_BOUND ( 'NONE', #241421, .T. ) ;
#80597=PLANE ( 'NONE',  #227386 ) ;
#80603=DIRECTION ( 'NONE',  ( -1.000000000000000000, 0.000000000000000000, 0.000000000000000000 ) ) ;
#80609=VECTOR ( 'NONE', #189011, 1000.000000000000000 ) ;
#80637=EDGE_CURVE ( 'NONE', #169297, #169606, #249174, .T. ) ;
#80656=VERTEX_POINT ( 'NONE', #233781 ) ;
#80672=ORIENTED_EDGE ( 'NONE', *, *, #224630, .T. ) ;
#80701=CIRCLE ( 'NONE', #1596, 0.09999999999999939493 ) ;
#80703=CARTESIAN_POINT ( 'NONE',  ( 21.00000000000000000, 6.644425182197215562, 9.641788261573355001 ) ) ;
#80737=AXIS2_PLACEMENT_3D ( 'NONE', #42102, #121638, #221964 ) ;
#80796=ADVANCED_FACE ( 'NONE', ( #198489 ), #25019, .T. ) ;
#80826=PLANE ( 'NONE',  #130715 ) ;
#80867=CARTESIAN_POINT ( 'NONE',  ( -20.90000000000000213, 1.311673547813416718, -7.986648289447971116 ) ) ;
#80875=AXIS2_PLACEMENT_3D ( 'NONE', #53877, #154308, #69600 ) ;
#80887=DIRECTION ( 'NONE',  ( 0.000000000000000000, 0.000000000000000000, 1.000000000000000000 ) ) ;
#80917=ORIENTED_EDGE ( 'NONE', *, *, #169577, .T. ) ;
#80939=DIRECTION ( 'NONE',  ( 1.000000000000000000, -0.000000000000000000, -0.000000000000000000 ) ) ;
#80955=ORIENTED_EDGE ( 'NONE', *, *, #142423, .T. ) ;
#80977=CARTESIAN_POINT ( 'NONE',  ( 20.90000000000000213, 6.356682116888462630, 11.91686199900910381 ) ) ;
#81036=AXIS2_PLACEMENT_3D ( 'NONE', #81177, #160772, #180304 ) ;
#81051=DIRECTION ( 'NONE',  ( 0.000000000000000000, 0.000000000000000000, -1.000000000000000000 ) ) ;
#81058=AXIS2_PLACEMENT_3D ( 'NONE', #130531, #232230, #107118 ) ;
#81065=ORIENTED_EDGE ( 'NONE', *, *, #172699, .F. ) ;
#81160=DIRECTION ( 'NONE',  ( 0.000000000000000000, 1.000000000000000000, 0.000000000000000000 ) ) ;
#81177=CARTESIAN_POINT ( 'NONE',  ( -18.79999999999999716, -8.250000000000005329, 22.10000000000000142 ) ) ;
#81211=CIRCLE ( 'NONE', #168782, 0.09999999999999939493 ) ;
#81234=AXIS2_PLACEMENT_3D ( 'NONE', #74656, #154197, #51161 ) ;
#81243=DIRECTION ( 'NONE',  ( 0.000000000000000000, 0.000000000000000000, -1.000000000000000000 ) ) ;
#81254=LINE ( 'NONE', #57842, #185445 ) ;
#81268=LINE ( 'NONE', #219510, #48115 ) ;
#81292=CARTESIAN_POINT ( 'NONE',  ( 20.10000000000000853, 5.552655413246003313, 16.61686199900910310 ) ) ;
#81300=DIRECTION ( 'NONE',  ( 0.000000000000000000, 0.000000000000000000, 1.000000000000000000 ) ) ;
#81309=DIRECTION ( 'NONE',  ( 0.000000000000000000, -0.1335171055202901691, -0.9910465087640861759 ) ) ;
#81334=CARTESIAN_POINT ( 'NONE',  ( 11.60000000000000320, -9.650000000000002132, 12.40000000000000391 ) ) ;
#81368=DIRECTION ( 'NONE',  ( 0.000000000000000000, 0.7071067811865472397, -0.7071067811865479058 ) ) ;
#81436=ADVANCED_FACE ( 'NONE', ( #115772 ), #94912, .T. ) ;
#81537=CARTESIAN_POINT ( 'NONE',  ( -11.60000000000000320, -8.279289321881350361, 18.97071067811866030 ) ) ;
#81555=EDGE_CURVE ( 'NONE', #216154, #45320, #203738, .T. ) ;
#81599=ORIENTED_EDGE ( 'NONE', *, *, #243676, .T. ) ;
#81612=CARTESIAN_POINT ( 'NONE',  ( -13.40000000000000213, -8.250000000000005329, 19.04142135623731491 ) ) ;
#81715=COLOUR_RGB ( '', 0.72549020, 0.75294118, 0.79215686) ;
#81733=VECTOR ( 'NONE', #201545, 1000.000000000000000 ) ;
#81740=CARTESIAN_POINT ( 'NONE',  ( 20.90000000000000213, 3.461118860469513336, 28.84309995045515507 ) ) ;
#81747=ADVANCED_FACE ( 'NONE', ( #247237 ), #223819, .F. ) ;
#81824=VERTEX_POINT ( 'NONE', #228982 ) ;
#81853=EDGE_LOOP ( 'NONE', ( #256872, #140046, #4828, #215321 ) ) ;
#81856=AXIS2_PLACEMENT_3D ( 'NONE', #172746, #116579, #35778 ) ;
#81869=ORIENTED_EDGE ( 'NONE', *, *, #221857, .T. ) ;
#81894=CIRCLE ( 'NONE', #119365, 3.970710678118657189 ) ;
#81958=ORIENTED_EDGE ( 'NONE', *, *, #243645, .F. ) ;
#81976=ORIENTED_EDGE ( 'NONE', *, *, #66088, .F. ) ;
#82031=EDGE_LOOP ( 'NONE', ( #175471, #210508, #232708, #195799 ) ) ;
#82064=DIRECTION ( 'NONE',  ( 0.000000000000000000, 0.9910465087640860649, -0.1335171055202901413 ) ) ;
#82072=AXIS2_PLACEMENT_3D ( 'NONE', #173666, #154092, #254395 ) ;
#82078=( BOUNDED_CURVE ( )  B_SPLINE_CURVE ( 3, ( #251689, #73096, #152625, #189152 ),
 .UNSPECIFIED., .F., .F. ) 
 B_SPLINE_CURVE_WITH_KNOTS ( ( 4, 4 ),
 ( 1.570796326794896558, 3.141592653589793116 ),
 .UNSPECIFIED. ) 
 CURVE ( )  GEOMETRIC_REPRESENTATION_ITEM ( )  RATIONAL_B_SPLINE_CURVE ( ( 1.000000000000000000, 0.8047378541243649375, 0.8047378541243649375, 1.000000000000000000 ) ) 
 REPRESENTATION_ITEM ( '' )  );
#82092=ORIENTED_EDGE ( 'NONE', *, *, #40887, .F. ) ;
#82095=VERTEX_POINT ( 'NONE', #124451 ) ;
#82102=CYLINDRICAL_SURFACE ( 'NONE', #163661, 0.09999999999999939493 ) ;
#82108=DIRECTION ( 'NONE',  ( 1.000000000000000000, 0.000000000000000000, -0.000000000000000000 ) ) ;
#82134=ORIENTED_EDGE ( 'NONE', *, *, #252839, .F. ) ;
#82204=VERTEX_POINT ( 'NONE', #82704 ) ;
#82209=ORIENTED_EDGE ( 'NONE', *, *, #86269, .F. ) ;
#82247=CARTESIAN_POINT ( 'NONE',  ( -6.000000000000002665, -11.75000000000000000, 13.90000000000000213 ) ) ;
#82267=ORIENTED_EDGE ( 'NONE', *, *, #43261, .F. ) ;
#82289=CARTESIAN_POINT ( 'NONE',  ( 5.899999999999995914, -11.25000000000000000, 10.10000000000000142 ) ) ;
#82322=EDGE_LOOP ( 'NONE', ( #203532, #3551, #78894, #113857 ) ) ;
#82335=CIRCLE ( 'NONE', #119803, 0.1000000000000028644 ) ;
#82398=DIRECTION ( 'NONE',  ( 0.000000000000000000, 1.156482317317873105E-15, -1.000000000000000000 ) ) ;
#82449=ORIENTED_EDGE ( 'NONE', *, *, #16433, .T. ) ;
#82453=DIRECTION ( 'NONE',  ( 0.000000000000000000, 0.000000000000000000, -1.000000000000000000 ) ) ;
#82477=CARTESIAN_POINT ( 'NONE',  ( 20.90000000000000213, 11.49641995933507843, 1.885425182446133885 ) ) ;
#82486=EDGE_CURVE ( 'NONE', #2147, #172709, #54065, .T. ) ;
#82505=FACE_OUTER_BOUND ( 'NONE', #33990, .T. ) ;
#82512=VERTEX_POINT ( 'NONE', #104538 ) ;
#82526=DIRECTION ( 'NONE',  ( -1.000000000000000000, -0.000000000000000000, -0.000000000000000000 ) ) ;
#82535=VERTEX_POINT ( 'NONE', #25065 ) ;
#82537=DIRECTION ( 'NONE',  ( 0.000000000000000000, 0.000000000000000000, 1.000000000000000000 ) ) ;
#82552=CARTESIAN_POINT ( 'NONE',  ( -20.90000000000000213, 7.900000000000000355, -1.212568896937008089 ) ) ;
#82598=EDGE_LOOP ( 'NONE', ( #60570, #4636, #71467, #55545 ) ) ;
#82672=AXIS2_PLACEMENT_3D ( 'NONE', #59890, #67290, #23390 ) ;
#82704=CARTESIAN_POINT ( 'NONE',  ( -18.69999999999999929, -8.150000000000005684, 32.89999999999999858 ) ) ;
#82734=ORIENTED_EDGE ( 'NONE', *, *, #171755, .T. ) ;
#82788=AXIS2_PLACEMENT_3D ( 'NONE', #231449, #232735, #225313 ) ;
#82902=ORIENTED_EDGE ( 'NONE', *, *, #177266, .F. ) ;
#82948=CARTESIAN_POINT ( 'NONE',  ( 19.96434256916586847, 5.572646937746800866, 16.50000000334722472 ) ) ;
#82953=ORIENTED_EDGE ( 'NONE', *, *, #52572, .T. ) ;
#83036=DIRECTION ( 'NONE',  ( 1.000000000000000000, 0.000000000000000000, 0.000000000000000000 ) ) ;
#83105=ADVANCED_FACE ( 'NONE', ( #90766 ), #72523, .T. ) ;
#83187=EDGE_CURVE ( 'NONE', #6496, #171633, #21337, .T. ) ;
#83189=ORIENTED_EDGE ( 'NONE', *, *, #241156, .T. ) ;
#83209=EDGE_CURVE ( 'NONE', #23059, #37930, #222256, .T. ) ;
#83235=ORIENTED_EDGE ( 'NONE', *, *, #198958, .T. ) ;
#83237=VERTEX_POINT ( 'NONE', #127042 ) ;
#83277=DIRECTION ( 'NONE',  ( 1.000000000000000000, 0.000000000000000000, 0.000000000000000000 ) ) ;
#83300=ORIENTED_EDGE ( 'NONE', *, *, #202166, .F. ) ;
#83304=DIRECTION ( 'NONE',  ( 1.000000000000000000, 0.000000000000000000, 0.000000000000000000 ) ) ;
#83339=LINE ( 'NONE', #199493, #221349 ) ;
#83442=ORIENTED_EDGE ( 'NONE', *, *, #106544, .T. ) ;
#83457=CARTESIAN_POINT ( 'NONE',  ( 18.69999999999999929, -1.410778198689825569, -7.973296578895943121 ) ) ;
#83469=ORIENTED_EDGE ( 'NONE', *, *, #74921, .T. ) ;
#83535=EDGE_CURVE ( 'NONE', #119824, #69468, #149941, .T. ) ;
#83569=CARTESIAN_POINT ( 'NONE',  ( -0.8999999999999980238, -11.65000000000000036, 28.60000000000000142 ) ) ;
#83572=CARTESIAN_POINT ( 'NONE',  ( -18.79999999999999716, 6.726092018229619995, 9.512212474619552438 ) ) ;
#83583=EDGE_CURVE ( 'NONE', #6496, #152492, #206282, .T. ) ;
#83611=CARTESIAN_POINT ( 'NONE',  ( 20.99999999999998934, -1.311673547813416718, -7.986648289447971116 ) ) ;
#83660=EDGE_CURVE ( 'NONE', #26765, #204919, #237415, .T. ) ;
#83691=CARTESIAN_POINT ( 'NONE',  ( 20.90000000000000213, 11.49641995933507843, -1.885425182446133885 ) ) ;
#83701=DIRECTION ( 'NONE',  ( -0.000000000000000000, 0.000000000000000000, 1.000000000000000000 ) ) ;
#83712=AXIS2_PLACEMENT_3D ( 'NONE', #26259, #256118, #185320 ) ;
#83713=VERTEX_POINT ( 'NONE', #186735 ) ;
#83716=VECTOR ( 'NONE', #181950, 1000.000000000000227 ) ;
#83733=DIRECTION ( 'NONE',  ( 0.000000000000000000, 8.673617379884087537E-15, 1.000000000000000000 ) ) ;
#83776=VERTEX_POINT ( 'NONE', #94022 ) ;
#83799=CARTESIAN_POINT ( 'NONE',  ( 18.59999999999999787, -8.350000000000004974, 32.89999999999999858 ) ) ;
#83814=CARTESIAN_POINT ( 'NONE',  ( -5.900000000000002132, -11.65000000000000036, 13.90000000000000213 ) ) ;
#83885=LINE ( 'NONE', #163472, #45936 ) ;
#83906=DIRECTION ( 'NONE',  ( -0.000000000000000000, 0.9910465087640860649, -0.1335171055202901413 ) ) ;
#83919=CARTESIAN_POINT ( 'NONE',  ( -21.00000000000000000, 7.986648289447971116, 1.311673547813416718 ) ) ;
#83921=DIRECTION ( 'NONE',  ( -0.000000000000000000, -0.9910465087640860649, 0.1335171055202901413 ) ) ;
#83931=CARTESIAN_POINT ( 'NONE',  ( 0.8999999999999980238, -8.250000000000005329, 21.95857864376268864 ) ) ;
#83935=CYLINDRICAL_SURFACE ( 'NONE', #183997, 0.09999999999999933942 ) ;
#84017=ADVANCED_FACE ( 'NONE', ( #105551 ), #2624, .T. ) ;
#84023=ORIENTED_EDGE ( 'NONE', *, *, #69625, .F. ) ;
#84072=CARTESIAN_POINT ( 'NONE',  ( -18.79999999999999716, -1.300000000000000044, -7.900000000000000355 ) ) ;
#84078=AXIS2_PLACEMENT_3D ( 'NONE', #247115, #68501, #227562 ) ;
#84128=VECTOR ( 'NONE', #187453, 1000.000000000000000 ) ;
#84150=CIRCLE ( 'NONE', #54966, 0.09999999999999939493 ) ;
#84159=PLANE ( 'NONE',  #214113 ) ;
#84163=ORIENTED_EDGE ( 'NONE', *, *, #217423, .F. ) ;
#84169=SURFACE_SIDE_STYLE ('',( #125911 ) ) ;
#84188=EDGE_LOOP ( 'NONE', ( #148065, #252608, #87924, #190763 ) ) ;
#84195=DIRECTION ( 'NONE',  ( 0.000000000000000000, -1.000000000000000000, -0.000000000000000000 ) ) ;
#84209=CARTESIAN_POINT ( 'NONE',  ( 19.90000000000000568, 5.488301202077012775, 16.50000000000000000 ) ) ;
#84235=DIRECTION ( 'NONE',  ( 0.000000000000000000, 0.000000000000000000, 1.000000000000000000 ) ) ;
#84248=CARTESIAN_POINT ( 'NONE',  ( 20.99999999999998934, 1.212568896937007645, -7.900000000000000355 ) ) ;
#84250=EDGE_CURVE ( 'NONE', #79944, #248319, #158700, .T. ) ;
#84265=VECTOR ( 'NONE', #195947, 1000.000000000000000 ) ;
#84361=CARTESIAN_POINT ( 'NONE',  ( -22.94999999999999929, 11.61130914238355771, -1.800000000000000044 ) ) ;
#84374=DIRECTION ( 'NONE',  ( 0.000000000000000000, 0.000000000000000000, -1.000000000000000000 ) ) ;
#84406=ADVANCED_FACE ( 'NONE', ( #101371 ), #140536, .T. ) ;
#84407=ORIENTED_EDGE ( 'NONE', *, *, #223611, .T. ) ;
#84419=ADVANCED_FACE ( 'NONE', ( #3600 ), #80545, .T. ) ;
#84422=ORIENTED_EDGE ( 'NONE', *, *, #98194, .F. ) ;
#84434=LINE ( 'NONE', #106592, #218177 ) ;
#84453=ORIENTED_EDGE ( 'NONE', *, *, #98074, .F. ) ;
#84503=DIRECTION ( 'NONE',  ( -1.000000000000000000, 0.000000000000000000, 0.000000000000000000 ) ) ;
#84532=DIRECTION ( 'NONE',  ( 0.000000000000000000, 0.000000000000000000, 1.000000000000000000 ) ) ;
#84550=CYLINDRICAL_SURFACE ( 'NONE', #220921, 0.1000000000000028644 ) ;
#84604=ORIENTED_EDGE ( 'NONE', *, *, #36075, .F. ) ;
#84633=DIRECTION ( 'NONE',  ( 0.000000000000000000, 1.000000000000000000, -0.000000000000000000 ) ) ;
#84647=ORIENTED_EDGE ( 'NONE', *, *, #145128, .F. ) ;
#84654=ADVANCED_FACE ( 'NONE', ( #198603 ), #19994, .T. ) ;
#84664=CARTESIAN_POINT ( 'NONE',  ( -22.94999999999999929, 0.000000000000000000, 0.000000000000000000 ) ) ;
#84667=CARTESIAN_POINT ( 'NONE',  ( 0.8999999999999992450, -8.279289321881350361, 29.97071067811866030 ) ) ;
#84711=TOROIDAL_SURFACE ( 'NONE', #251335, 11.65000000000000036, 0.1000000000000000056 ) ;
#84718=VERTEX_POINT ( 'NONE', #18688 ) ;
#84755=AXIS2_PLACEMENT_3D ( 'NONE', #52256, #251761, #232224 ) ;
#84782=DIRECTION ( 'NONE',  ( 1.000000000000000000, 0.000000000000000000, 0.000000000000000000 ) ) ;
#84785=DIRECTION ( 'NONE',  ( 0.000000000000000000, 0.000000000000000000, -1.000000000000000000 ) ) ;
#84823=VERTEX_POINT ( 'NONE', #130626 ) ;
#84843=DIRECTION ( 'NONE',  ( 0.000000000000000000, 0.1335171055202901413, -0.9910465087640860649 ) ) ;
#84857=CARTESIAN_POINT ( 'NONE',  ( 20.01715728752538936, 4.611773100472912112, 22.11686199900910665 ) ) ;
#84864=EDGE_CURVE ( 'NONE', #22402, #144975, #212747, .T. ) ;
#84891=CARTESIAN_POINT ( 'NONE',  ( 5.999999999999995559, -11.65000000000000036, 10.10000000000000142 ) ) ;
#84912=DIRECTION ( 'NONE',  ( -0.000000000000000000, 1.000000000000000000, -0.000000000000000000 ) ) ;
#84924=CARTESIAN_POINT ( 'NONE',  ( -18.70000000000000284, 1.212568896937007645, -7.900000000000000355 ) ) ;
#84965=ORIENTED_EDGE ( 'NONE', *, *, #7332, .T. ) ;
#84970=LINE ( 'NONE', #189251, #240588 ) ;
#84971=EDGE_CURVE ( 'NONE', #166706, #73306, #222856, .T. ) ;
#85033=DIRECTION ( 'NONE',  ( 0.000000000000000000, -1.000000000000000000, 0.000000000000000000 ) ) ;
#85129=TOROIDAL_SURFACE ( 'NONE', #80875, 2.699999999999999734, 0.1000000000000000056 ) ;
#85133=CARTESIAN_POINT ( 'NONE',  ( 18.79999999999999716, 1.901609089591594470, -11.59510167572422112 ) ) ;
#85146=DIRECTION ( 'NONE',  ( 0.000000000000000000, 0.000000000000000000, -1.000000000000000000 ) ) ;
#85181=CARTESIAN_POINT ( 'NONE',  ( -18.59999999999999787, -10.64999999999999325, 31.59999999999999787 ) ) ;
#85199=LINE ( 'NONE', #206473, #112430 ) ;
#85205=DIRECTION ( 'NONE',  ( 0.000000000000000000, 1.445602896647339410E-16, -1.000000000000000000 ) ) ;
#85221=VECTOR ( 'NONE', #37452, 1000.000000000000114 ) ;
#85252=DIRECTION ( 'NONE',  ( -1.000000000000000000, 0.000000000000000000, 0.000000000000000000 ) ) ;
#85270=ORIENTED_EDGE ( 'NONE', *, *, #210495, .F. ) ;
#85271=EDGE_CURVE ( 'NONE', #22402, #46601, #117342, .T. ) ;
#85281=ORIENTED_EDGE ( 'NONE', *, *, #225939, .T. ) ;
#85286=AXIS2_PLACEMENT_3D ( 'NONE', #178392, #132834, #192804 ) ;
#85301=ADVANCED_FACE ( 'NONE', ( #177040 ), #59036, .T. ) ;
#85309=ORIENTED_EDGE ( 'NONE', *, *, #26937, .T. ) ;
#85336=CARTESIAN_POINT ( 'NONE',  ( 11.60000000000000142, -8.250000000000005329, 10.95857864376269575 ) ) ;
#85353=ORIENTED_EDGE ( 'NONE', *, *, #216028, .F. ) ;
#85382=VECTOR ( 'NONE', #92156, 1000.000000000000000 ) ;
#85503=EDGE_CURVE ( 'NONE', #228920, #109505, #107895, .T. ) ;
#85507=DIRECTION ( 'NONE',  ( -1.000000000000000000, 0.000000000000000000, 0.000000000000000000 ) ) ;
#85637=DIRECTION ( 'NONE',  ( -0.000000000000000000, 1.000000000000000000, -0.000000000000000000 ) ) ;
#85668=EDGE_LOOP ( 'NONE', ( #103041, #74973, #52505, #142387 ) ) ;
#85671=CARTESIAN_POINT ( 'NONE',  ( -19.99999999999999645, 11.61130914238355771, 22.00000000000000355 ) ) ;
#85677=UNCERTAINTY_MEASURE_WITH_UNIT (LENGTH_MEASURE( 1.000000000000000082E-05 ), #111500, 'distance_accuracy_value', 'NONE');
#85692=LINE ( 'NONE', #161443, #123620 ) ;
#85694=DIRECTION ( 'NONE',  ( -1.000000000000000000, 0.000000000000000000, -0.000000000000000000 ) ) ;
#85723=AXIS2_PLACEMENT_3D ( 'NONE', #163444, #146420, #85146 ) ;
#85752=CARTESIAN_POINT ( 'NONE',  ( 21.00000000000000000, 0.000000000000000000, 0.000000000000000000 ) ) ;
#85764=CARTESIAN_POINT ( 'NONE',  ( -18.79999999999999716, 1.885425182446133885, -11.49641995933507843 ) ) ;
#85772=CIRCLE ( 'NONE', #231568, 0.1000000000000002554 ) ;
#85820=LINE ( 'NONE', #204509, #254761 ) ;
#85837=SPHERICAL_SURFACE ( 'NONE', #16759, 0.1000000000000000056 ) ;
#85957=FACE_OUTER_BOUND ( 'NONE', #62933, .T. ) ;
#86052=ORIENTED_EDGE ( 'NONE', *, *, #3449, .T. ) ;
#86103=AXIS2_PLACEMENT_3D ( 'NONE', #69549, #149087, #30420 ) ;
#86110=CIRCLE ( 'NONE', #223673, 0.09999999999999990841 ) ;
#86158=EDGE_CURVE ( 'NONE', #41292, #103483, #185545, .T. ) ;
#86173=CIRCLE ( 'NONE', #115417, 0.09999999999999939493 ) ;
#86187=CARTESIAN_POINT ( 'NONE',  ( -22.84999999999999787, 4.898587196589412829E-16, 4.000000000000000000 ) ) ;
#86210=CARTESIAN_POINT ( 'NONE',  ( 21.00000000000000000, 0.000000000000000000, -4.100000000000000533 ) ) ;
#86227=ORIENTED_EDGE ( 'NONE', *, *, #68165, .F. ) ;
#86236=VERTEX_POINT ( 'NONE', #82552 ) ;
#86266=ORIENTED_EDGE ( 'NONE', *, *, #2358, .T. ) ;
#86268=CARTESIAN_POINT ( 'NONE',  ( -19.89999999999999858, 1.350000000000000089, 0.000000000000000000 ) ) ;
#86269=EDGE_CURVE ( 'NONE', #181190, #77088, #36450, .T. ) ;
#86291=CARTESIAN_POINT ( 'NONE',  ( -19.89999999999999858, 4.513204987021262937, 22.00000000000000355 ) ) ;
#86293=VERTEX_POINT ( 'NONE', #251616 ) ;
#86333=ORIENTED_EDGE ( 'NONE', *, *, #209548, .F. ) ;
#86339=ADVANCED_FACE ( 'NONE', ( #136790 ), #97647, .T. ) ;
#86340=CARTESIAN_POINT ( 'NONE',  ( -22.20000000000000284, 6.223900101154157483, 12.09999999999999787 ) ) ;
#86343=ORIENTED_EDGE ( 'NONE', *, *, #184384, .F. ) ;
#86365=CARTESIAN_POINT ( 'NONE',  ( 0.8999999999999993561, -11.65000000000000036, 26.00000000000000355 ) ) ;
#86373=EDGE_CURVE ( 'NONE', #172709, #208877, #88630, .T. ) ;
#86464=ORIENTED_EDGE ( 'NONE', *, *, #164334, .F. ) ;
#86541=TOROIDAL_SURFACE ( 'NONE', #103122, 0.2000000000000000111, 0.1000000000000000056 ) ;
#86547=VECTOR ( 'NONE', #109113, 999.9999999999998863 ) ;
#86550=DIRECTION ( 'NONE',  ( 1.000000000000000000, 0.000000000000000000, 0.000000000000000000 ) ) ;
#86661=DIRECTION ( 'NONE',  ( 0.000000000000000000, 0.000000000000000000, 1.000000000000000000 ) ) ;
#86675=ORIENTED_EDGE ( 'NONE', *, *, #201292, .T. ) ;
#86682=ORIENTED_EDGE ( 'NONE', *, *, #194129, .F. ) ;
#86685=EDGE_CURVE ( 'NONE', #125866, #83776, #175637, .T. ) ;
#86768=AXIS2_PLACEMENT_3D ( 'NONE', #30045, #52129, #53430 ) ;
#86802=DIRECTION ( 'NONE',  ( -1.000000000000000000, -0.000000000000000000, -0.000000000000000000 ) ) ;
#86804=ORIENTED_EDGE ( 'NONE', *, *, #8418, .T. ) ;
#86825=TOROIDAL_SURFACE ( 'NONE', #45153, 0.2000000000000000111, 0.1000000000000000056 ) ;
#86847=EDGE_CURVE ( 'NONE', #171323, #59375, #19107, .T. ) ;
#86910=CARTESIAN_POINT ( 'NONE',  ( 22.10000000000000142, -11.65000000000000036, 32.89999999999999858 ) ) ;
#86931=AXIS2_PLACEMENT_3D ( 'NONE', #17525, #61810, #80043 ) ;
#86947=ADVANCED_FACE ( 'NONE', ( #157376 ), #217289, .T. ) ;
#87019=LINE ( 'NONE', #47906, #19177 ) ;
#87047=ORIENTED_EDGE ( 'NONE', *, *, #234542, .F. ) ;
#87054=ADVANCED_FACE ( 'NONE', ( #89336 ), #84159, .T. ) ;
#87070=VECTOR ( 'NONE', #180232, 1000.000000000000000 ) ;
#87074=CIRCLE ( 'NONE', #57851, 0.09999999999999939493 ) ;
#87078=DIRECTION ( 'NONE',  ( 0.000000000000000000, 0.000000000000000000, -1.000000000000000000 ) ) ;
#87093=( NAMED_UNIT ( * ) SI_UNIT ( $, .STERADIAN. ) SOLID_ANGLE_UNIT ( ) );
#87143=CIRCLE ( 'NONE', #183024, 0.09999999999999939493 ) ;
#87160=CARTESIAN_POINT ( 'NONE',  ( -18.69999999999999929, -9.849999999999996092, 31.39999999999999858 ) ) ;
#87189=DIRECTION ( 'NONE',  ( 1.000000000000000000, 0.000000000000000000, 0.000000000000000000 ) ) ;
#87211=VERTEX_POINT ( 'NONE', #254792 ) ;
#87223=EDGE_CURVE ( 'NONE', #204755, #84823, #1792, .T. ) ;
#87235=DIRECTION ( 'NONE',  ( 0.000000000000000000, -0.9856811345164803173, -0.1686199900910455851 ) ) ;
#87275=DIRECTION ( 'NONE',  ( 1.000000000000000000, 0.000000000000000000, 0.000000000000000000 ) ) ;
#87298=DIRECTION ( 'NONE',  ( 1.000000000000000000, 0.000000000000000000, 0.000000000000000000 ) ) ;
#87308=CIRCLE ( 'NONE', #37271, 0.1000000000000001860 ) ;
#87315=FACE_OUTER_BOUND ( 'NONE', #165049, .T. ) ;
#87439=CIRCLE ( 'NONE', #170900, 0.1999999999999996503 ) ;
#87441=EDGE_CURVE ( 'NONE', #209609, #691, #171211, .T. ) ;
#87443=LINE ( 'NONE', #228264, #6844 ) ;
#87543=EDGE_CURVE ( 'NONE', #161554, #21663, #210300, .T. ) ;
#87584=ORIENTED_EDGE ( 'NONE', *, *, #116209, .F. ) ;
#87622=AXIS2_PLACEMENT_3D ( 'NONE', #89466, #248550, #127328 ) ;
#87625=EDGE_CURVE ( 'NONE', #72694, #89956, #251707, .T. ) ;
#87634=ORIENTED_EDGE ( 'NONE', *, *, #94478, .T. ) ;
#87649=AXIS2_PLACEMENT_3D ( 'NONE', #62169, #36202, #195281 ) ;
#87688=ADVANCED_FACE ( 'NONE', ( #221815, #241418 ), #2777, .T. ) ;
#87738=ORIENTED_EDGE ( 'NONE', *, *, #127080, .F. ) ;
#87759=LINE ( 'NONE', #232450, #206838 ) ;
#87827=AXIS2_PLACEMENT_3D ( 'NONE', #128031, #172334, #251814 ) ;
#87857=DIRECTION ( 'NONE',  ( 0.000000000000000000, -1.000000000000000000, 0.000000000000000000 ) ) ;
#87910=DIRECTION ( 'NONE',  ( -1.000000000000000000, -0.000000000000000000, -0.000000000000000000 ) ) ;
#87924=ORIENTED_EDGE ( 'NONE', *, *, #174992, .T. ) ;
#88008=VERTEX_POINT ( 'NONE', #135566 ) ;
#88058=ORIENTED_EDGE ( 'NONE', *, *, #46749, .F. ) ;
#88074=CARTESIAN_POINT ( 'NONE',  ( -19.99999999999999645, 1.350000000000000089, 22.00000000000000355 ) ) ;
#88120=LINE ( 'NONE', #166443, #34006 ) ;
#88121=DIRECTION ( 'NONE',  ( 0.000000000000000000, 0.1335171055202901691, 0.9910465087640861759 ) ) ;
#88191=DIRECTION ( 'NONE',  ( 1.000000000000000000, -0.000000000000000000, -0.000000000000000000 ) ) ;
#88200=FACE_OUTER_BOUND ( 'NONE', #168497, .T. ) ;
#88254=DIRECTION ( 'NONE',  ( 0.000000000000000000, -0.4856429311786307212, -0.8741572761215384846 ) ) ;
#88340=ORIENTED_EDGE ( 'NONE', *, *, #154758, .F. ) ;
#88407=DIRECTION ( 'NONE',  ( -1.000000000000000000, 0.000000000000000000, 0.000000000000000000 ) ) ;
#88422=DIRECTION ( 'NONE',  ( 0.000000000000000000, 0.000000000000000000, 1.000000000000000000 ) ) ;
#88438=VECTOR ( 'NONE', #144512, 1000.000000000000000 ) ;
#88439=DIRECTION ( 'NONE',  ( -1.000000000000000000, -0.000000000000000000, -0.000000000000000000 ) ) ;
#88441=FACE_OUTER_BOUND ( 'NONE', #18940, .T. ) ;
#88454=ADVANCED_FACE ( 'NONE', ( #5674 ), #168684, .F. ) ;
#88463=DIRECTION ( 'NONE',  ( -2.489438768765009500E-17, -0.1686199900910313187, 0.9856811345164828708 ) ) ;
#88476=VERTEX_POINT ( 'NONE', #143921 ) ;
#88501=LINE ( 'NONE', #190211, #253508 ) ;
#88506=FACE_OUTER_BOUND ( 'NONE', #233101, .T. ) ;
#88597=CARTESIAN_POINT ( 'NONE',  ( 0.9000000000000014655, -11.75000000000000000, 28.70000000000000284 ) ) ;
#88630=CIRCLE ( 'NONE', #172088, 0.09999999999999939493 ) ;
#88675=CARTESIAN_POINT ( 'NONE',  ( -22.20000000000000284, 10.88519226655716565, -15.14794223642649840 ) ) ;
#88679=AXIS2_PLACEMENT_3D ( 'NONE', #10787, #242958, #64337 ) ;
#88692=DIRECTION ( 'NONE',  ( 0.000000000000000000, 0.000000000000000000, -1.000000000000000000 ) ) ;
#88694=AXIS2_PLACEMENT_3D ( 'NONE', #237898, #175395, #45802 ) ;
#88713=DIRECTION ( 'NONE',  ( 0.000000000000000000, 0.000000000000000000, 1.000000000000000000 ) ) ;
#88718=FACE_OUTER_BOUND ( 'NONE', #246789, .T. ) ;
#88746=CARTESIAN_POINT ( 'NONE',  ( 0.8999999999999993561, -11.65000000000000036, 23.40000000000000568 ) ) ;
#88812=EDGE_LOOP ( 'NONE', ( #117073, #28413, #131568, #186568 ) ) ;
#88886=CARTESIAN_POINT ( 'NONE',  ( 22.19999999999999929, -11.75000000000000355, 12.09999999999999609 ) ) ;
#88922=ORIENTED_EDGE ( 'NONE', *, *, #218301, .T. ) ;
#88932=EDGE_LOOP ( 'NONE', ( #168250, #148982, #119362, #31600 ) ) ;
#88946=ORIENTED_EDGE ( 'NONE', *, *, #155913, .F. ) ;
#88949=VERTEX_POINT ( 'NONE', #178479 ) ;
#88982=ADVANCED_FACE ( 'NONE', ( #217554 ), #38955, .F. ) ;
#88985=DIRECTION ( 'NONE',  ( 0.000000000000000000, 0.000000000000000000, -1.000000000000000000 ) ) ;
#88993=AXIS2_PLACEMENT_3D ( 'NONE', #166914, #67773, #229425 ) ;
#88994=ADVANCED_FACE ( 'NONE', ( #239715 ), #102733, .F. ) ;
#89023=DIRECTION ( 'NONE',  ( -0.000000000000000000, -0.000000000000000000, 1.000000000000000000 ) ) ;
#89072=VERTEX_POINT ( 'NONE', #1234 ) ;
#89163=FACE_OUTER_BOUND ( 'NONE', #186800, .T. ) ;
#89173=ADVANCED_FACE ( 'NONE', ( #68957 ), #169360, .T. ) ;
#89178=CARTESIAN_POINT ( 'NONE',  ( 20.90000000000000213, 1.885425182446133885, -11.59641995933507808 ) ) ;
#89197=CARTESIAN_POINT ( 'NONE',  ( 19.90000000000000568, 1.250000000000000000, 21.90000000000000213 ) ) ;
#89225=VERTEX_POINT ( 'NONE', #250142 ) ;
#89234=VERTEX_POINT ( 'NONE', #6387 ) ;
#89280=DIRECTION ( 'NONE',  ( -1.000000000000000000, 0.000000000000000000, 0.000000000000000000 ) ) ;
#89336=FACE_OUTER_BOUND ( 'NONE', #174908, .T. ) ;
#89342=CARTESIAN_POINT ( 'NONE',  ( 18.79999999999999716, 5.488301202077012775, 16.40000000000000213 ) ) ;
#89347=( NAMED_UNIT ( * ) SI_UNIT ( $, .STERADIAN. ) SOLID_ANGLE_UNIT ( ) );
#89349=AXIS2_PLACEMENT_3D ( 'NONE', #108140, #49449, #27362 ) ;
#89368=ORIENTED_EDGE ( 'NONE', *, *, #90551, .F. ) ;
#89381=CIRCLE ( 'NONE', #147661, 0.09999999999999939493 ) ;
#89403=DIRECTION ( 'NONE',  ( 0.000000000000000000, 0.000000000000000000, 1.000000000000000000 ) ) ;
#89450=DIRECTION ( 'NONE',  ( 0.000000000000000000, 0.000000000000000000, 1.000000000000000000 ) ) ;
#89466=CARTESIAN_POINT ( 'NONE',  ( -37.88850191057539973, 11.75000000000000000, 31.50000000000000000 ) ) ;
#89487=DIRECTION ( 'NONE',  ( 0.000000000000000000, 0.000000000000000000, -1.000000000000000000 ) ) ;
#89507=AXIS2_PLACEMENT_3D ( 'NONE', #134731, #179052, #18658 ) ;
#89523=ORIENTED_EDGE ( 'NONE', *, *, #122964, .T. ) ;
#89578=DIRECTION ( 'NONE',  ( 1.000000000000000000, 0.000000000000000000, 0.000000000000000000 ) ) ;
#89611=VERTEX_POINT ( 'NONE', #184709 ) ;
#89658=LINE ( 'NONE', #169254, #54403 ) ;
#89704=LINE ( 'NONE', #10199, #15519 ) ;
#89714=AXIS2_PLACEMENT_3D ( 'NONE', #49114, #111662, #247313 ) ;
#89717=AXIS2_PLACEMENT_3D ( 'NONE', #155516, #254545, #5040 ) ;
#89737=ORIENTED_EDGE ( 'NONE', *, *, #164334, .T. ) ;
#89739=CARTESIAN_POINT ( 'NONE',  ( -21.00000000000000000, 6.356682116888462630, 11.91686199900910381 ) ) ;
#89740=LINE ( 'NONE', #49344, #230895 ) ;
#89756=VERTEX_POINT ( 'NONE', #11223 ) ;
#89758=CIRCLE ( 'NONE', #235508, 0.1000000000000000056 ) ;
#89773=ORIENTED_EDGE ( 'NONE', *, *, #154758, .T. ) ;
#89777=DIRECTION ( 'NONE',  ( -0.000000000000000000, 1.000000000000000000, -0.000000000000000000 ) ) ;
#89778=PLANE ( 'NONE',  #121454 ) ;
#89785=EDGE_LOOP ( 'NONE', ( #10454, #232298, #32901, #155887 ) ) ;
#89794=ORIENTED_EDGE ( 'NONE', *, *, #98194, .T. ) ;
#89867=DIRECTION ( 'NONE',  ( 0.000000000000000000, 0.000000000000000000, 1.000000000000000000 ) ) ;
#89877=VECTOR ( 'NONE', #190683, 1000.000000000000000 ) ;
#89956=VERTEX_POINT ( 'NONE', #126690 ) ;
#89987=ADVANCED_FACE ( 'NONE', ( #148834 ), #30178, .T. ) ;
#90004=EDGE_CURVE ( 'NONE', #41107, #130397, #201307, .T. ) ;
#90023=CARTESIAN_POINT ( 'NONE',  ( 20.10000000000000853, 4.645987002755569861, 21.91686199900910736 ) ) ;
#90035=EDGE_CURVE ( 'NONE', #217909, #70167, #197221, .T. ) ;
#90052=EDGE_CURVE ( 'NONE', #45320, #139155, #69299, .T. ) ;
#90062=ORIENTED_EDGE ( 'NONE', *, *, #167827, .T. ) ;
#90108=CARTESIAN_POINT ( 'NONE',  ( 20.89999999999999858, -11.65000000000000036, -15.00000000000000000 ) ) ;
#90115=CARTESIAN_POINT ( 'NONE',  ( 18.69999999999999929, 1.149999999999999911, 21.90000000000000213 ) ) ;
#90127=EDGE_LOOP ( 'NONE', ( #98234, #251138, #175848, #22866 ) ) ;
#90188=FACE_OUTER_BOUND ( 'NONE', #151942, .T. ) ;
#90191=ORIENTED_EDGE ( 'NONE', *, *, #233408, .T. ) ;
#90235=EDGE_LOOP ( 'NONE', ( #153448, #111027, #76419, #208319 ) ) ;
#90258=CARTESIAN_POINT ( 'NONE',  ( 5.899999999999995914, -11.34999999999999964, 10.10000000000000142 ) ) ;
#90299=LINE ( 'NONE', #8225, #116387 ) ;
#90316=EDGE_CURVE ( 'NONE', #198523, #136731, #72337, .T. ) ;
#90322=CARTESIAN_POINT ( 'NONE',  ( 5.899999999999995914, -11.25000000000000000, 10.00000000000000178 ) ) ;
#90331=ORIENTED_EDGE ( 'NONE', *, *, #14271, .T. ) ;
#90346=DIRECTION ( 'NONE',  ( -0.000000000000000000, -0.1686199900910463068, 0.9856811345164802063 ) ) ;
#90397=ADVANCED_FACE ( 'NONE', ( #88506 ), #147222, .F. ) ;
#90414=ORIENTED_EDGE ( 'NONE', *, *, #37189, .T. ) ;
#90421=CARTESIAN_POINT ( 'NONE',  ( -18.79999999999999716, 0.000000000000000000, 0.000000000000000000 ) ) ;
#90485=CARTESIAN_POINT ( 'NONE',  ( 18.59999999999999787, -10.84999999999999076, 32.89999999999999858 ) ) ;
#90536=EDGE_CURVE ( 'NONE', #189932, #176334, #180652, .T. ) ;
#90551=EDGE_CURVE ( 'NONE', #58688, #172629, #17969, .T. ) ;
#90619=DIRECTION ( 'NONE',  ( 0.000000000000000000, -1.000000000000000000, 0.000000000000000000 ) ) ;
#90659=AXIS2_PLACEMENT_3D ( 'NONE', #131575, #211115, #87298 ) ;
#90690=VERTEX_POINT ( 'NONE', #149508 ) ;
#90702=VECTOR ( 'NONE', #111733, 1000.000000000000000 ) ;
#90718=DIRECTION ( 'NONE',  ( 1.000000000000000000, -0.000000000000000000, 0.000000000000000000 ) ) ;
#90739=EDGE_CURVE ( 'NONE', #210883, #171697, #197570, .T. ) ;
#90752=ADVANCED_FACE ( 'NONE', ( #49086 ), #128648, .T. ) ;
#90766=FACE_OUTER_BOUND ( 'NONE', #241479, .T. ) ;
#90805=CARTESIAN_POINT ( 'NONE',  ( -18.69999999999999929, 8.000000000000000000, 1.212568896937007867 ) ) ;
#90834=AXIS2_PLACEMENT_3D ( 'NONE', #251501, #194131, #95000 ) ;
#90936=CIRCLE ( 'NONE', #136717, 2.699999999999999289 ) ;
#90945=ORIENTED_EDGE ( 'NONE', *, *, #163347, .T. ) ;
#90984=AXIS2_PLACEMENT_3D ( 'NONE', #180794, #140359, #102494 ) ;
#91020=DIRECTION ( 'NONE',  ( 0.000000000000000000, 0.000000000000000000, -1.000000000000000000 ) ) ;
#91145=DIRECTION ( 'NONE',  ( 0.000000000000000000, -0.1335171055202901413, 0.9910465087640860649 ) ) ;
#91156=CIRCLE ( 'NONE', #3653, 4.041421356237310469 ) ;
#91182=DIRECTION ( 'NONE',  ( 1.000000000000000000, 0.000000000000000000, 0.000000000000000000 ) ) ;
#91205=EDGE_LOOP ( 'NONE', ( #103062, #206416, #86227, #28361 ) ) ;
#91216=DIRECTION ( 'NONE',  ( 0.000000000000000000, -0.5773469543544729188, -0.8164989248600478255 ) ) ;
#91235=EDGE_CURVE ( 'NONE', #47981, #163656, #39588, .T. ) ;
#91258=VECTOR ( 'NONE', #141995, 1000.000000000000000 ) ;
#91259=EDGE_LOOP ( 'NONE', ( #212513, #11946, #57261 ) ) ;
#91317=CARTESIAN_POINT ( 'NONE',  ( -20.90000000000000213, 11.49641995933507843, -1.885425182446133885 ) ) ;
#91340=ADVANCED_FACE ( 'NONE', ( #181603 ), #2933, .T. ) ;
#91341=ADVANCED_FACE ( 'NONE', ( #99454 ), #240288, .F. ) ;
#91361=LINE ( 'NONE', #204856, #75200 ) ;
#91465=CIRCLE ( 'NONE', #49760, 0.09999999999999939493 ) ;
#91483=ORIENTED_EDGE ( 'NONE', *, *, #234520, .T. ) ;
#91491=VERTEX_POINT ( 'NONE', #132856 ) ;
#91496=AXIS2_PLACEMENT_3D ( 'NONE', #25642, #26953, #166466 ) ;
#91499=VERTEX_POINT ( 'NONE', #44651 ) ;
#91517=EDGE_CURVE ( 'NONE', #169022, #136640, #202057, .T. ) ;
#91575=LINE ( 'NONE', #92845, #148086 ) ;
#91617=DIRECTION ( 'NONE',  ( 0.000000000000000000, 0.000000000000000000, -1.000000000000000000 ) ) ;
#91659=ORIENTED_EDGE ( 'NONE', *, *, #128994, .F. ) ;
#91704=ORIENTED_EDGE ( 'NONE', *, *, #110517, .T. ) ;
#91799=ORIENTED_EDGE ( 'NONE', *, *, #96181, .F. ) ;
#91802=EDGE_CURVE ( 'NONE', #160911, #234077, #209490, .T. ) ;
#91817=ORIENTED_EDGE ( 'NONE', *, *, #209568, .T. ) ;
#91909=CARTESIAN_POINT ( 'NONE',  ( -18.69999999999999929, 10.31653824539118069, -11.82383137372478110 ) ) ;
#91939=EDGE_CURVE ( 'NONE', #59375, #215604, #135577, .T. ) ;
#91989=DIRECTION ( 'NONE',  ( -1.000000000000000000, 0.000000000000000000, 0.000000000000000000 ) ) ;
#92015=EDGE_CURVE ( 'NONE', #198523, #18345, #217177, .T. ) ;
#92032=AXIS2_PLACEMENT_3D ( 'NONE', #230285, #193740, #131184 ) ;
#92035=DIRECTION ( 'NONE',  ( 1.000000000000000000, 1.476360405086644309E-16, -0.000000000000000000 ) ) ;
#92101=CYLINDRICAL_SURFACE ( 'NONE', #214100, 0.1000000000000000472 ) ;
#92156=DIRECTION ( 'NONE',  ( 1.000000000000000000, 0.000000000000000000, 0.000000000000000000 ) ) ;
#92174=CARTESIAN_POINT ( 'NONE',  ( -20.90000000000000213, 1.212568896937007645, -7.800000000000000711 ) ) ;
#92180=VERTEX_POINT ( 'NONE', #67112 ) ;
#92221=DIRECTION ( 'NONE',  ( -0.000000000000000000, 0.9910465087640860649, 0.1335171055202901413 ) ) ;
#92236=CARTESIAN_POINT ( 'NONE',  ( -11.60000000000000320, -11.75000000000000000, 17.70000000000000639 ) ) ;
#92326=ADVANCED_FACE ( 'NONE', ( #189638 ), #70994, .T. ) ;
#92338=FACE_OUTER_BOUND ( 'NONE', #153370, .T. ) ;
#92366=AXIS2_PLACEMENT_3D ( 'NONE', #96397, #175981, #93845 ) ;
#92377=AXIS2_PLACEMENT_3D ( 'NONE', #58318, #77898, #76620 ) ;
#92393=CARTESIAN_POINT ( 'NONE',  ( 0.8999999999999992450, -8.279289321881350361, 22.02928932188134326 ) ) ;
#92420=ORIENTED_EDGE ( 'NONE', *, *, #38254, .F. ) ;
#92428=ADVANCED_FACE ( 'NONE', ( #111376 ), #202413, .T. ) ;
#92441=AXIS2_PLACEMENT_3D ( 'NONE', #182961, #121709, #97260 ) ;
#92445=DIRECTION ( 'NONE',  ( -1.476360405086644309E-16, -1.000000000000000000, -1.445602896647339410E-16 ) ) ;
#92448=VERTEX_POINT ( 'NONE', #154393 ) ;
#92469=CARTESIAN_POINT ( 'NONE',  ( -21.00000000000000000, 0.000000000000000000, 0.000000000000000000 ) ) ;
#92476=CARTESIAN_POINT ( 'NONE',  ( -18.79999999999999716, 7.900000000000000355, 1.212568896937007867 ) ) ;
#92478=EDGE_LOOP ( 'NONE', ( #130816, #175934, #210640, #230036 ) ) ;
#92485=CIRCLE ( 'NONE', #21778, 0.09999999999999939493 ) ;
#92499=ORIENTED_EDGE ( 'NONE', *, *, #230025, .T. ) ;
#92500=CARTESIAN_POINT ( 'NONE',  ( 18.79999999999999005, 8.000000000000000000, -1.212568896937008089 ) ) ;
#92527=CARTESIAN_POINT ( 'NONE',  ( -0.8999999999999993561, -11.65000000000000036, 28.70000000000000284 ) ) ;
#92553=CIRCLE ( 'NONE', #13469, 0.09999999999999939493 ) ;
#92587=VECTOR ( 'NONE', #198493, 1000.000000000000000 ) ;
#92663=ORIENTED_EDGE ( 'NONE', *, *, #186911, .T. ) ;
#92686=DIRECTION ( 'NONE',  ( -0.000000000000000000, -0.000000000000000000, 1.000000000000000000 ) ) ;
#92697=DIRECTION ( 'NONE',  ( 0.000000000000000000, 0.000000000000000000, 1.000000000000000000 ) ) ;
#92734=CARTESIAN_POINT ( 'NONE',  ( -22.94999999999999929, 11.49641995933507843, -1.885425182446134107 ) ) ;
#92774=EDGE_LOOP ( 'NONE', ( #211514, #33596, #177494, #99226 ) ) ;
#92791=FACE_OUTER_BOUND ( 'NONE', #94293, .T. ) ;
#92803=AXIS2_PLACEMENT_3D ( 'NONE', #240628, #162392, #183231 ) ;
#92845=CARTESIAN_POINT ( 'NONE',  ( 19.90000000000000568, 1.250000000000000000, 16.50000000000000000 ) ) ;
#92855=VERTEX_POINT ( 'NONE', #119861 ) ;
#92872=CARTESIAN_POINT ( 'NONE',  ( -18.79999999999999716, 5.488301202077016328, 16.39999999999999858 ) ) ;
#92889=DIRECTION ( 'NONE',  ( 0.000000000000000000, 0.000000000000000000, 1.000000000000000000 ) ) ;
#92927=VERTEX_POINT ( 'NONE', #222768 ) ;
#92957=ADVANCED_FACE ( 'NONE', ( #4992 ), #68864, .T. ) ;
#92995=VECTOR ( 'NONE', #76607, 1000.000000000000000 ) ;
#93022=ORIENTED_EDGE ( 'NONE', *, *, #245743, .F. ) ;
#93071=VECTOR ( 'NONE', #16132, 1000.000000000000000 ) ;
#93079=ORIENTED_EDGE ( 'NONE', *, *, #63052, .T. ) ;
#93088=ORIENTED_EDGE ( 'NONE', *, *, #175225, .F. ) ;
#93171=CARTESIAN_POINT ( 'NONE',  ( -18.79999999999999716, 7.799999999999999822, 1.212568896937007867 ) ) ;
#93173=FACE_OUTER_BOUND ( 'NONE', #230455, .T. ) ;
#93189=DIRECTION ( 'NONE',  ( -5.790381434762883172E-16, 0.9910465087640865089, 0.1335171055202867274 ) ) ;
#93207=( NAMED_UNIT ( * ) PLANE_ANGLE_UNIT ( ) SI_UNIT ( $, .RADIAN. ) );
#93256=AXIS2_PLACEMENT_3D ( 'NONE', #191907, #109753, #48504 ) ;
#93316=ORIENTED_EDGE ( 'NONE', *, *, #153227, .T. ) ;
#93347=DIRECTION ( 'NONE',  ( 0.000000000000000000, -1.000000000000000000, 0.000000000000000000 ) ) ;
#93367=FACE_OUTER_BOUND ( 'NONE', #80216, .T. ) ;
#93376=EDGE_CURVE ( 'NONE', #975, #129212, #111382, .T. ) ;
#93383=AXIS2_PLACEMENT_3D ( 'NONE', #108710, #188244, #9592 ) ;
#93388=DIRECTION ( 'NONE',  ( -1.000000000000000000, 0.000000000000000000, 0.000000000000000000 ) ) ;
#93454=SPHERICAL_SURFACE ( 'NONE', #251424, 0.1000000000000000056 ) ;
#93544=CARTESIAN_POINT ( 'NONE',  ( -20.90000000000000213, 6.258114003436813455, 11.90000000000000036 ) ) ;
#93628=FACE_OUTER_BOUND ( 'NONE', #219481, .T. ) ;
#93681=FACE_OUTER_BOUND ( 'NONE', #163646, .T. ) ;
#93744=DIRECTION ( 'NONE',  ( 0.000000000000000000, 0.000000000000000000, 1.000000000000000000 ) ) ;
#93750=ORIENTED_EDGE ( 'NONE', *, *, #29048, .F. ) ;
#93760=DIRECTION ( 'NONE',  ( 0.000000000000000000, 0.000000000000000000, -1.000000000000000000 ) ) ;
#93782=ADVANCED_FACE ( 'NONE', ( #160925 ), #169879, .F. ) ;
#93845=DIRECTION ( 'NONE',  ( 0.000000000000000000, 0.000000000000000000, 1.000000000000000000 ) ) ;
#93857=ORIENTED_EDGE ( 'NONE', *, *, #87543, .F. ) ;
#93865=VERTEX_POINT ( 'NONE', #229875 ) ;
#93871=FACE_OUTER_BOUND ( 'NONE', #97854, .T. ) ;
#93879=DIRECTION ( 'NONE',  ( 0.000000000000000000, 0.000000000000000000, 1.000000000000000000 ) ) ;
#93885=DIRECTION ( 'NONE',  ( -1.000000000000000000, 0.000000000000000000, -0.000000000000000000 ) ) ;
#93900=LINE ( 'NONE', #173504, #19811 ) ;
#93902=AXIS2_PLACEMENT_3D ( 'NONE', #217532, #195451, #78034 ) ;
#93985=DIRECTION ( 'NONE',  ( 0.000000000000000000, 0.1335171055202867274, 0.9910465087640866200 ) ) ;
#94002=CARTESIAN_POINT ( 'NONE',  ( 18.79999999999999716, 10.88519226655716565, -15.14794223642649840 ) ) ;
#94022=CARTESIAN_POINT ( 'NONE',  ( 21.00000000000000000, 11.49641995933507843, 1.885425182446133885 ) ) ;
#94038=DIRECTION ( 'NONE',  ( 0.000000000000000000, 0.000000000000000000, 1.000000000000000000 ) ) ;
#94090=EDGE_CURVE ( 'NONE', #203870, #223079, #70077, .T. ) ;
#94194=EDGE_CURVE ( 'NONE', #78387, #203718, #240930, .T. ) ;
#94208=FACE_OUTER_BOUND ( 'NONE', #229328, .T. ) ;
#94218=ADVANCED_FACE ( 'NONE', ( #172215 ), #28603, .F. ) ;
#94267=CARTESIAN_POINT ( 'NONE',  ( 22.10000000000000142, -11.65000000000000036, 32.89999999999999858 ) ) ;
#94284=ORIENTED_EDGE ( 'NONE', *, *, #11419, .T. ) ;
#94293=EDGE_LOOP ( 'NONE', ( #140823, #165662, #181390, #32775 ) ) ;
#94332=CARTESIAN_POINT ( 'NONE',  ( -19.89999999999999858, 1.350000000000000089, 21.90000000000000213 ) ) ;
#94336=VERTEX_POINT ( 'NONE', #198137 ) ;
#94345=CARTESIAN_POINT ( 'NONE',  ( -22.10000000000000142, -1.467286812112899463, 33.00000000000000000 ) ) ;
#94389=EDGE_CURVE ( 'NONE', #22402, #107433, #93900, .T. ) ;
#94427=VECTOR ( 'NONE', #106217, 1000.000000000000000 ) ;
#94449=CIRCLE ( 'NONE', #219354, 0.09999999999999939493 ) ;
#94477=AXIS2_PLACEMENT_3D ( 'NONE', #168654, #166060, #72083 ) ;
#94478=EDGE_CURVE ( 'NONE', #147074, #92855, #224359, .T. ) ;
#94487=EDGE_CURVE ( 'NONE', #99741, #235390, #49008, .T. ) ;
#94534=FACE_OUTER_BOUND ( 'NONE', #231407, .T. ) ;
#94553=CYLINDRICAL_SURFACE ( 'NONE', #59299, 0.09999999999999990841 ) ;
#94571=ADVANCED_FACE ( 'NONE', ( #189815 ), #15039, .F. ) ;
#94600=DIRECTION ( 'NONE',  ( 0.000000000000000000, 1.000000000000000000, 0.000000000000000000 ) ) ;
#94616=EDGE_CURVE ( 'NONE', #46280, #233154, #191064, .T. ) ;
#94633=DIRECTION ( 'NONE',  ( 1.000000000000000000, -0.000000000000000000, 0.000000000000000000 ) ) ;
#94682=EDGE_LOOP ( 'NONE', ( #238609, #234167, #217563, #35153 ) ) ;
#94713=DIRECTION ( 'NONE',  ( 1.000000000000000000, 0.000000000000000000, 0.000000000000000000 ) ) ;
#94763=EDGE_LOOP ( 'NONE', ( #244144, #172518, #140064 ) ) ;
#94784=DIRECTION ( 'NONE',  ( 1.000000000000000000, 0.000000000000000000, 0.000000000000000000 ) ) ;
#94820=DIRECTION ( 'NONE',  ( 0.000000000000000000, 0.000000000000000000, 1.000000000000000000 ) ) ;
#94864=FACE_OUTER_BOUND ( 'NONE', #134437, .T. ) ;
#94912=PLANE ( 'NONE',  #107865 ) ;
#94972=FACE_OUTER_BOUND ( 'NONE', #16244, .T. ) ;
#95000=DIRECTION ( 'NONE',  ( 0.000000000000000000, 0.000000000000000000, 1.000000000000000000 ) ) ;
#95010=ORIENTED_EDGE ( 'NONE', *, *, #29971, .F. ) ;
#95024=DIRECTION ( 'NONE',  ( -0.000000000000000000, 0.000000000000000000, 1.000000000000000000 ) ) ;
#95037=FACE_OUTER_BOUND ( 'NONE', #100538, .T. ) ;
#95059=ORIENTED_EDGE ( 'NONE', *, *, #57290, .T. ) ;
#95135=FACE_OUTER_BOUND ( 'NONE', #101786, .T. ) ;
#95175=ORIENTED_EDGE ( 'NONE', *, *, #87441, .F. ) ;
#95248=EDGE_CURVE ( 'NONE', #131374, #104540, #181516, .T. ) ;
#95253=CARTESIAN_POINT ( 'NONE',  ( -18.79999999999999716, -11.65000000000000036, 0.000000000000000000 ) ) ;
#95259=CARTESIAN_POINT ( 'NONE',  ( -20.90000000000000213, 8.000000000000000000, -1.212568896937008089 ) ) ;
#95324=DIRECTION ( 'NONE',  ( 0.000000000000000000, 0.000000000000000000, -1.000000000000000000 ) ) ;
#95328=CARTESIAN_POINT ( 'NONE',  ( -22.94999999999999929, 11.49641995933507843, 1.885425182446134107 ) ) ;
#95333=EDGE_CURVE ( 'NONE', #691, #173524, #152674, .T. ) ;
#95338=AXIS2_PLACEMENT_3D ( 'NONE', #247629, #10322, #209795 ) ;
#95343=DIRECTION ( 'NONE',  ( -1.000000000000000000, 0.000000000000000000, 0.000000000000000000 ) ) ;
#95395=ORIENTED_EDGE ( 'NONE', *, *, #63875, .T. ) ;
#95433=ORIENTED_EDGE ( 'NONE', *, *, #235614, .T. ) ;
#95439=LINE ( 'NONE', #150296, #228421 ) ;
#95460=LINE ( 'NONE', #117597, #156960 ) ;
#95471=ORIENTED_EDGE ( 'NONE', *, *, #32888, .T. ) ;
#95474=CARTESIAN_POINT ( 'NONE',  ( 18.69999999999999929, -10.84999999999999076, 31.59999999999999787 ) ) ;
#95485=VECTOR ( 'NONE', #22128, 1000.000000000000114 ) ;
#95499=DIRECTION ( 'NONE',  ( 0.000000000000000000, 0.9910465087640860649, -0.1335171055202901413 ) ) ;
#95524=DIRECTION ( 'NONE',  ( 0.000000000000000000, 0.000000000000000000, -1.000000000000000000 ) ) ;
#95525=DIRECTION ( 'NONE',  ( 0.000000000000000000, 0.000000000000000000, -1.000000000000000000 ) ) ;
#95554=AXIS2_PLACEMENT_3D ( 'NONE', #27687, #6794, #147592 ) ;
#95570=VERTEX_POINT ( 'NONE', #66381 ) ;
#95585=ORIENTED_EDGE ( 'NONE', *, *, #35431, .T. ) ;
#95599=CARTESIAN_POINT ( 'NONE',  ( -20.90000000000000213, 7.973296578895943121, 1.410778198689825347 ) ) ;
#95616=LINE ( 'NONE', #210453, #161768 ) ;
#95655=EDGE_LOOP ( 'NONE', ( #69923, #64132, #72807, #103899 ) ) ;
#95697=CIRCLE ( 'NONE', #120673, 0.09999999999999939493 ) ;
#95699=CIRCLE ( 'NONE', #12529, 11.65000000000000036 ) ;
#95700=EDGE_CURVE ( 'NONE', #127870, #80656, #53654, .T. ) ;
#95724=CARTESIAN_POINT ( 'NONE',  ( 19.90000000000000568, 5.586869315528661062, 16.41686199900910736 ) ) ;
#95749=EDGE_CURVE ( 'NONE', #166926, #183834, #190192, .T. ) ;
#95764=APPLICATION_CONTEXT ( 'automotive_design' ) ;
#95774=FACE_OUTER_BOUND ( 'NONE', #226102, .T. ) ;
#95791=CARTESIAN_POINT ( 'NONE',  ( -18.79999999999999716, 11.59510167572422112, -1.901609089591594470 ) ) ;
#95878=LINE ( 'NONE', #73792, #243984 ) ;
#95898=ORIENTED_EDGE ( 'NONE', *, *, #135117, .T. ) ;
#95903=EDGE_CURVE ( 'NONE', #9700, #18932, #57907, .T. ) ;
#95972=DIRECTION ( 'NONE',  ( -0.000000000000000000, 0.000000000000000000, -1.000000000000000000 ) ) ;
#95996=EDGE_LOOP ( 'NONE', ( #194029, #105298, #55335 ) ) ;
#96004=TOROIDAL_SURFACE ( 'NONE', #158591, 4.041421356237312246, 0.1000000000000000056 ) ;
#96016=CARTESIAN_POINT ( 'NONE',  ( -0.8999999999999993561, -8.250000000000005329, 28.60000000000000142 ) ) ;
#96044=DIRECTION ( 'NONE',  ( -1.000000000000000000, 0.000000000000000000, -0.000000000000000000 ) ) ;
#96052=ORIENTED_EDGE ( 'NONE', *, *, #133360, .T. ) ;
#96054=AXIS2_PLACEMENT_3D ( 'NONE', #127756, #6504, #7810 ) ;
#96181=EDGE_CURVE ( 'NONE', #242362, #60954, #232863, .T. ) ;
#96197=CARTESIAN_POINT ( 'NONE',  ( 21.10000000000000142, 6.342459739679072506, 12.00000000000000000 ) ) ;
#96203=CARTESIAN_POINT ( 'NONE',  ( 20.90000000326035590, 6.338045365888074656, 12.02580456186802671 ) ) ;
#96232=DIRECTION ( 'NONE',  ( 0.000000000000000000, 1.000000000000000000, 0.000000000000000000 ) ) ;
#96238=LINE ( 'NONE', #59662, #184048 ) ;
#96267=ORIENTED_EDGE ( 'NONE', *, *, #183752, .T. ) ;
#96270=ORIENTED_EDGE ( 'NONE', *, *, #75031, .T. ) ;
#96395=EDGE_LOOP ( 'NONE', ( #171091, #218482, #62871, #129246 ) ) ;
#96397=CARTESIAN_POINT ( 'NONE',  ( -22.84999999999999787, 0.000000000000000000, 0.000000000000000000 ) ) ;
#96398=DIRECTION ( 'NONE',  ( -1.000000000000000000, 0.000000000000000000, 0.000000000000000000 ) ) ;
#96401=EDGE_CURVE ( 'NONE', #181466, #37087, #90299, .T. ) ;
#96420=EDGE_CURVE ( 'NONE', #156184, #114049, #128870, .T. ) ;
#96426=CARTESIAN_POINT ( 'NONE',  ( 5.899999999999996803, -11.65000000000000036, 14.00000000000000178 ) ) ;
#96437=FACE_OUTER_BOUND ( 'NONE', #112701, .T. ) ;
#96461=EDGE_CURVE ( 'NONE', #209609, #176903, #43340, .T. ) ;
#96522=CARTESIAN_POINT ( 'NONE',  ( -11.60000000000000320, -8.250000000000007105, 12.40000000000000391 ) ) ;
#96583=CARTESIAN_POINT ( 'NONE',  ( -18.59999999999999787, -8.262584272387851314, 10.47734830970188824 ) ) ;
#96617=ADVANCED_FACE ( 'NONE', ( #46911 ), #127765, .T. ) ;
#96754=CARTESIAN_POINT ( 'NONE',  ( -19.99999999999999645, 5.472724050409169649, 16.54552871969761796 ) ) ;
#96767=EDGE_CURVE ( 'NONE', #224623, #190789, #95699, .T. ) ;
#96797=DIRECTION ( 'NONE',  ( 1.000000000000000000, -1.734723475976817507E-14, 0.000000000000000000 ) ) ;
#96835=ORIENTED_EDGE ( 'NONE', *, *, #97666, .F. ) ;
#96903=CARTESIAN_POINT ( 'NONE',  ( 22.10000000000000497, 6.223900101154161923, 12.09999999999999964 ) ) ;
#96960=LINE ( 'NONE', #256018, #17973 ) ;
#96968=CARTESIAN_POINT ( 'NONE',  ( -20.90000000000000213, -11.65000000000000036, 0.000000000000000000 ) ) ;
#97005=CARTESIAN_POINT ( 'NONE',  ( -19.99999999999999645, 5.488301202077012775, 16.50000000000000000 ) ) ;
#97013=SPHERICAL_SURFACE ( 'NONE', #103844, 0.1000000000000000056 ) ;
#97041=DIRECTION ( 'NONE',  ( -1.000000000000000000, 0.000000000000000000, 0.000000000000000000 ) ) ;
#97115=CARTESIAN_POINT ( 'NONE',  ( -18.79999999999999716, 7.973296578895943121, -1.410778198689825791 ) ) ;
#97159=CARTESIAN_POINT ( 'NONE',  ( -21.10000000000000142, 6.223900101154156594, 12.09999999999999964 ) ) ;
#97203=CARTESIAN_POINT ( 'NONE',  ( 18.79999999999999716, 1.885425182446133663, -11.49641995933507843 ) ) ;
#97231=CARTESIAN_POINT ( 'NONE',  ( -5.900000000000003020, -11.75000000000000000, 10.10000000000000142 ) ) ;
#97236=AXIS2_PLACEMENT_3D ( 'NONE', #114596, #196685, #93744 ) ;
#97260=DIRECTION ( 'NONE',  ( 1.000000000000000000, 0.000000000000000000, 0.000000000000000000 ) ) ;
#97290=ADVANCED_FACE ( 'NONE', ( #143805 ), #103380, .T. ) ;
#97303=DIRECTION ( 'NONE',  ( 0.000000000000000000, -0.1335171055202867274, -0.9910465087640866200 ) ) ;
#97305=CARTESIAN_POINT ( 'NONE',  ( -22.94999999999999929, -1.786320531569725478, -11.50977166988710820 ) ) ;
#97381=CARTESIAN_POINT ( 'NONE',  ( -0.8999999999999993561, -9.650000000000003908, 26.00000000000000355 ) ) ;
#97387=DIRECTION ( 'NONE',  ( -0.000000000000000000, -0.000000000000000000, -1.000000000000000000 ) ) ;
#97401=CARTESIAN_POINT ( 'NONE',  ( 21.10000000000000142, -11.75000000000000000, 11.89999999999999680 ) ) ;
#97416=DIRECTION ( 'NONE',  ( 1.000000000000000000, -0.000000000000000000, 0.000000000000000000 ) ) ;
#97445=LINE ( 'NONE', #239561, #32130 ) ;
#97454=FACE_OUTER_BOUND ( 'NONE', #192735, .T. ) ;
#97459=CARTESIAN_POINT ( 'NONE',  ( -13.40000000000000213, -8.279289321881350361, 15.00000000000000355 ) ) ;
#97467=CARTESIAN_POINT ( 'NONE',  ( 21.10000000000000497, 6.342459739679071618, 12.00000000000000355 ) ) ;
#97471=CARTESIAN_POINT ( 'NONE',  ( -22.94999999999999929, 0.000000000000000000, 0.000000000000000000 ) ) ;
#97490=VERTEX_POINT ( 'NONE', #212791 ) ;
#97494=CARTESIAN_POINT ( 'NONE',  ( -18.79999999999999716, -1.786320531569725478, -11.50977166988710820 ) ) ;
#97514=DIRECTION ( 'NONE',  ( -1.000000000000000000, -0.000000000000000000, -0.000000000000000000 ) ) ;
#97530=ORIENTED_EDGE ( 'NONE', *, *, #178631, .F. ) ;
#97534=CARTESIAN_POINT ( 'NONE',  ( -20.90000000000000213, 6.742993295648862961, 9.658650260582458458 ) ) ;
#97537=CARTESIAN_POINT ( 'NONE',  ( 22.10000000000000497, 6.223900101154157483, 12.09999999999999964 ) ) ;
#97541=VERTEX_POINT ( 'NONE', #255708 ) ;
#97593=DIRECTION ( 'NONE',  ( 0.000000000000000000, 0.000000000000000000, 1.000000000000000000 ) ) ;
#97647=SPHERICAL_SURFACE ( 'NONE', #138682, 0.1000000000000000056 ) ;
#97653=DIRECTION ( 'NONE',  ( 1.000000000000000000, 0.000000000000000000, 0.000000000000000000 ) ) ;
#97654=CARTESIAN_POINT ( 'NONE',  ( -0.8999999999999991340, -9.650000000000003908, 23.40000000000000213 ) ) ;
#97666=EDGE_CURVE ( 'NONE', #120372, #14875, #80118, .T. ) ;
#97711=AXIS2_PLACEMENT_3D ( 'NONE', #37228, #58032, #201414 ) ;
#97712=FACE_OUTER_BOUND ( 'NONE', #56230, .T. ) ;
#97752=LINE ( 'NONE', #19545, #188311 ) ;
#97774=EDGE_LOOP ( 'NONE', ( #117255, #79039, #74075, #83469 ) ) ;
#97781=ORIENTED_EDGE ( 'NONE', *, *, #7108, .F. ) ;
#97800=VECTOR ( 'NONE', #128183, 1000.000000000000000 ) ;
#97808=ORIENTED_EDGE ( 'NONE', *, *, #170387, .T. ) ;
#97810=CYLINDRICAL_SURFACE ( 'NONE', #246669, 0.09999999999999939493 ) ;
#97832=LINE ( 'NONE', #213968, #51741 ) ;
#97854=EDGE_LOOP ( 'NONE', ( #95059, #8968, #183679, #126982 ) ) ;
#97871=EDGE_CURVE ( 'NONE', #173524, #38945, #129089, .T. ) ;
#97882=CIRCLE ( 'NONE', #110379, 0.1000000000000002554 ) ;
#97966=DIRECTION ( 'NONE',  ( 0.000000000000000000, 0.000000000000000000, -1.000000000000000000 ) ) ;
#98031=ORIENTED_EDGE ( 'NONE', *, *, #56859, .F. ) ;
#98037=CARTESIAN_POINT ( 'NONE',  ( -11.60000000000000320, -8.350000000000004974, 15.00000000000000355 ) ) ;
#98051=CARTESIAN_POINT ( 'NONE',  ( 18.69999999999999929, -11.65000000000000036, 32.89999999999999858 ) ) ;
#98074=EDGE_CURVE ( 'NONE', #184776, #201448, #109560, .T. ) ;
#98100=AXIS2_PLACEMENT_3D ( 'NONE', #193129, #35370, #71900 ) ;
#98150=VERTEX_POINT ( 'NONE', #122362 ) ;
#98194=EDGE_CURVE ( 'NONE', #99532, #84823, #71538, .T. ) ;
#98227=EDGE_CURVE ( 'NONE', #253747, #39190, #238570, .T. ) ;
#98234=ORIENTED_EDGE ( 'NONE', *, *, #182490, .T. ) ;
#98238=CIRCLE ( 'NONE', #252381, 0.2000000000000000944 ) ;
#98252=CARTESIAN_POINT ( 'NONE',  ( -18.79999999999999716, 1.149999999999999911, 16.60000000000000142 ) ) ;
#98282=DIRECTION ( 'NONE',  ( 1.000000000000000000, 0.000000000000000000, -0.000000000000000000 ) ) ;
#98287=ORIENTED_EDGE ( 'NONE', *, *, #218301, .F. ) ;
#98341=CARTESIAN_POINT ( 'NONE',  ( 18.59999999999999787, -8.262584272387851314, 10.47734830970188824 ) ) ;
#98360=CARTESIAN_POINT ( 'NONE',  ( -18.79999999999999716, 1.350000000000000089, 16.60000000000000142 ) ) ;
#98368=VERTEX_POINT ( 'NONE', #195191 ) ;
#98416=AXIS2_PLACEMENT_3D ( 'NONE', #136229, #112851, #131121 ) ;
#98439=EDGE_CURVE ( 'NONE', #118720, #182139, #162949, .T. ) ;
#98510=EDGE_CURVE ( 'NONE', #84718, #46280, #100355, .T. ) ;
#98512=DIRECTION ( 'NONE',  ( 1.000000000000000000, 0.000000000000000000, 0.000000000000000000 ) ) ;
#98535=VECTOR ( 'NONE', #73398, 1000.000000000000000 ) ;
#98556=CARTESIAN_POINT ( 'NONE',  ( 21.00000000000000000, 6.258114003436814343, 11.90000000000000036 ) ) ;
#98558=EDGE_CURVE ( 'NONE', #79286, #183834, #227553, .T. ) ;
#98559=EDGE_CURVE ( 'NONE', #10010, #36888, #250403, .T. ) ;
#98578=DIRECTION ( 'NONE',  ( 0.000000000000000000, -0.9910465087640865089, 0.1335171055202867274 ) ) ;
#98632=FACE_OUTER_BOUND ( 'NONE', #18109, .T. ) ;
#98651=ORIENTED_EDGE ( 'NONE', *, *, #168222, .F. ) ;
#98736=LINE ( 'NONE', #252091, #122738 ) ;
#98763=DIRECTION ( 'NONE',  ( 0.000000000000000000, -0.000000000000000000, -1.000000000000000000 ) ) ;
#98775=DIRECTION ( 'NONE',  ( -0.000000000000000000, -0.000000000000000000, 1.000000000000000000 ) ) ;
#98789=VECTOR ( 'NONE', #85637, 1000.000000000000000 ) ;
#98822=CARTESIAN_POINT ( 'NONE',  ( 5.999999999999995559, -11.25000000000000000, 10.00000000000000178 ) ) ;
#98854=ORIENTED_EDGE ( 'NONE', *, *, #75607, .T. ) ;
#98872=TOROIDAL_SURFACE ( 'NONE', #194799, 0.2000000000000000111, 0.1000000000000000056 ) ;
#98899=VERTEX_POINT ( 'NONE', #47310 ) ;
#98924=VECTOR ( 'NONE', #194303, 1000.000000000000000 ) ;
#98946=ORIENTED_EDGE ( 'NONE', *, *, #212768, .F. ) ;
#98977=FACE_OUTER_BOUND ( 'NONE', #29521, .T. ) ;
#99040=CYLINDRICAL_SURFACE ( 'NONE', #119711, 11.75000000000000000 ) ;
#99045=EDGE_CURVE ( 'NONE', #192176, #48243, #254650, .T. ) ;
#99068=CYLINDRICAL_SURFACE ( 'NONE', #159599, 0.1000000000000000472 ) ;
#99073=DIRECTION ( 'NONE',  ( 0.000000000000000000, 0.9910465087640865089, 0.1335171055202867274 ) ) ;
#99081=EDGE_CURVE ( 'NONE', #206620, #132097, #183959, .T. ) ;
#99083=CARTESIAN_POINT ( 'NONE',  ( -21.00000000000000000, 1.212568896937007645, -7.800000000000000711 ) ) ;
#99087=CARTESIAN_POINT ( 'NONE',  ( 20.90000000000000213, 6.841561409100513025, 9.675512259591560138 ) ) ;
#99100=ADVANCED_FACE ( 'NONE', ( #95135 ), #208895, .T. ) ;
#99118=EDGE_CURVE ( 'NONE', #41516, #219374, #192330, .T. ) ;
#99187=VERTEX_POINT ( 'NONE', #64983 ) ;
#99189=ORIENTED_EDGE ( 'NONE', *, *, #103593, .F. ) ;
#99201=CIRCLE ( 'NONE', #40993, 0.09999999999999939493 ) ;
#99209=VERTEX_POINT ( 'NONE', #178553 ) ;
#99224=EDGE_LOOP ( 'NONE', ( #8650, #12888, #207011, #171771 ) ) ;
#99226=ORIENTED_EDGE ( 'NONE', *, *, #219217, .F. ) ;
#99232=VECTOR ( 'NONE', #29448, 1000.000000000000000 ) ;
#99239=CARTESIAN_POINT ( 'NONE',  ( -18.69999999999999929, 1.212568896937007645, -8.000000000000000000 ) ) ;
#99242=CIRCLE ( 'NONE', #211511, 0.09999999999999939493 ) ;
#99243=ADVANCED_FACE ( 'NONE', ( #41604 ), #183666, .T. ) ;
#99254=ADVANCED_FACE ( 'NONE', ( #184935 ), #29751, .T. ) ;
#99293=DIRECTION ( 'NONE',  ( 0.000000000000000000, -0.5773469543544729188, -0.8164989248600478255 ) ) ;
#99326=CARTESIAN_POINT ( 'NONE',  ( -22.94999999999999929, -1.300000000000000044, -7.900000000000000355 ) ) ;
#99357=VECTOR ( 'NONE', #85507, 1000.000000000000000 ) ;
#99361=ORIENTED_EDGE ( 'NONE', *, *, #58865, .F. ) ;
#99378=AXIS2_PLACEMENT_3D ( 'NONE', #121775, #162187, #40962 ) ;
#99389=VECTOR ( 'NONE', #79393, 1000.000000000000227 ) ;
#99411=LINE ( 'NONE', #138530, #107301 ) ;
#99421=AXIS2_PLACEMENT_3D ( 'NONE', #196833, #116041, #133037 ) ;
#99430=CIRCLE ( 'NONE', #86768, 3.900000000000000355 ) ;
#99449=DIRECTION ( 'NONE',  ( 0.000000000000000000, 0.1335171055202901413, -0.9910465087640860649 ) ) ;
#99452=FACE_OUTER_BOUND ( 'NONE', #193870, .T. ) ;
#99454=FACE_OUTER_BOUND ( 'NONE', #133596, .T. ) ;
#99457=FACE_OUTER_BOUND ( 'NONE', #45652, .T. ) ;
#99458=CARTESIAN_POINT ( 'NONE',  ( 18.69999999999999929, 7.800000000000000711, 1.212568896937007867 ) ) ;
#99481=DIRECTION ( 'NONE',  ( 0.000000000000000000, 0.000000000000000000, -1.000000000000000000 ) ) ;
#99510=DIRECTION ( 'NONE',  ( 1.000000000000000000, -0.000000000000000000, -0.000000000000000000 ) ) ;
#99529=EDGE_CURVE ( 'NONE', #10423, #219183, #133937, .T. ) ;
#99532=VERTEX_POINT ( 'NONE', #115674 ) ;
#99552=EDGE_LOOP ( 'NONE', ( #93079, #173310, #21648, #133223 ) ) ;
#99601=DIRECTION ( 'NONE',  ( 0.000000000000000000, -1.000000000000000000, -0.000000000000000000 ) ) ;
#99655=DIRECTION ( 'NONE',  ( -2.168404344971008868E-16, -0.000000000000000000, -1.000000000000000000 ) ) ;
#99656=( BOUNDED_SURFACE ( )  B_SPLINE_SURFACE ( 3, 2, ( 
 ( #26479, #6897, #105974 ),
 ( #240386, #182986, #201239 ),
 ( #222062, #185542, #123010 ),
 ( #3030, #164699, #22636 ) ),
 .UNSPECIFIED., .F., .F., .F. ) 
 B_SPLINE_SURFACE_WITH_KNOTS ( ( 4, 4 ),
 ( 3, 3 ),
 ( 3.141592653589793116, 4.712388980384689674 ),
 ( 0.000000000000000000, 1.000000000000000000 ),
 .UNSPECIFIED. ) 
 GEOMETRIC_REPRESENTATION_ITEM ( )  RATIONAL_B_SPLINE_SURFACE ( (
 ( 1.000000000000000000, 0.6447402616204922499, 1.000000000000000000),
 ( 1.000000000000000000, 0.6438648806865591157, 1.000000000000000000),
 ( 1.000000000000000000, 0.6753870962079413509, 1.000000000000000000),
 ( 1.000000000000000000, 0.7071067811865475727, 1.000000000000000000) ) ) 
 REPRESENTATION_ITEM ( '' )  SURFACE ( )  );
#99669=DIRECTION ( 'NONE',  ( 0.000000000000000000, 0.9910465087640866200, 0.1335171055202867274 ) ) ;
#99702=EDGE_CURVE ( 'NONE', #82512, #34850, #133677, .T. ) ;
#99710=DIRECTION ( 'NONE',  ( 0.000000000000000000, -1.000000000000000000, 0.000000000000000000 ) ) ;
#99741=VERTEX_POINT ( 'NONE', #30719 ) ;
#99756=ORIENTED_EDGE ( 'NONE', *, *, #249589, .F. ) ;
#99773=DIRECTION ( 'NONE',  ( -1.000000000000000000, 0.000000000000000000, -0.000000000000000000 ) ) ;
#99867=VECTOR ( 'NONE', #189888, 1000.000000000000000 ) ;
#99874=CARTESIAN_POINT ( 'NONE',  ( -20.90000000000000213, 0.000000000000000000, 0.000000000000000000 ) ) ;
#99885=ORIENTED_EDGE ( 'NONE', *, *, #17319, .T. ) ;
#99903=CARTESIAN_POINT ( 'NONE',  ( -18.60000000000000142, -8.150000000000005684, 32.89999999999999858 ) ) ;
#99922=VECTOR ( 'NONE', #32142, 1000.000000000000000 ) ;
#99931=DIRECTION ( 'NONE',  ( -1.000000000000000000, 0.000000000000000000, 0.000000000000000000 ) ) ;
#99989=DIRECTION ( 'NONE',  ( -1.000000000000000000, 0.000000000000000000, 0.000000000000000000 ) ) ;
#100041=EDGE_CURVE ( 'NONE', #18345, #27940, #229724, .T. ) ;
#100042=EDGE_CURVE ( 'NONE', #201448, #89956, #54757, .T. ) ;
#100050=PRODUCT_DEFINITION_CONTEXT ( 'detailed design', #95764, 'design' ) ;
#100076=CARTESIAN_POINT ( 'NONE',  ( 20.00000000000000355, 4.631764625546179737, 21.90000000000000213 ) ) ;
#100081=CARTESIAN_POINT ( 'NONE',  ( 13.40000000000000036, -11.75000000000000000, 15.00000000000000355 ) ) ;
#100109=CARTESIAN_POINT ( 'NONE',  ( -20.90000000000000213, 7.900000000000000355, 1.300000000000000044 ) ) ;
#100158=DIRECTION ( 'NONE',  ( 1.000000000000000000, 0.000000000000000000, 0.000000000000000000 ) ) ;
#100185=ORIENTED_EDGE ( 'NONE', *, *, #25043, .T. ) ;
#100191=DIRECTION ( 'NONE',  ( 0.000000000000000000, -0.000000000000000000, 1.000000000000000000 ) ) ;
#100226=CARTESIAN_POINT ( 'NONE',  ( 5.999999999999995559, -11.65000000000000036, 10.00000000000000178 ) ) ;
#100294=DIRECTION ( 'NONE',  ( 0.000000000000000000, 0.000000000000000000, -1.000000000000000000 ) ) ;
#100313=PRODUCT_CONTEXT ( 'NONE', #127392, 'mechanical' ) ;
#100355=CIRCLE ( 'NONE', #137964, 0.1000000000000002554 ) ;
#100362=ORIENTED_EDGE ( 'NONE', *, *, #111236, .F. ) ;
#100398=ORIENTED_EDGE ( 'NONE', *, *, #133655, .T. ) ;
#100427=DIRECTION ( 'NONE',  ( -0.000000000000000000, 0.000000000000000000, 1.000000000000000000 ) ) ;
#100538=EDGE_LOOP ( 'NONE', ( #257810, #68261, #46077, #169779 ) ) ;
#100555=CARTESIAN_POINT ( 'NONE',  ( 20.00000000000000355, 1.350000000000000089, 16.60000000000000142 ) ) ;
#100666=CARTESIAN_POINT ( 'NONE',  ( -18.60000000000000142, -8.250000000000005329, 10.52591260281975138 ) ) ;
#100703=CYLINDRICAL_SURFACE ( 'NONE', #68160, 0.09999999999999939493 ) ;
#100705=DIRECTION ( 'NONE',  ( 0.000000000000000000, 1.000000000000000000, 0.000000000000000000 ) ) ;
#100775=CYLINDRICAL_SURFACE ( 'NONE', #167045, 11.75000000000000000 ) ;
#100790=ADVANCED_FACE ( 'NONE', ( #197514 ), #119286, .F. ) ;
#100795=DIRECTION ( 'NONE',  ( 0.000000000000000000, -1.000000000000000000, 0.000000000000000000 ) ) ;
#100809=DIRECTION ( 'NONE',  ( -1.000000000000000000, 0.000000000000000000, 0.000000000000000000 ) ) ;
#100812=DIRECTION ( 'NONE',  ( -1.000000000000000000, -0.000000000000000000, -0.000000000000000000 ) ) ;
#100875=EDGE_CURVE ( 'NONE', #88008, #8033, #80207, .T. ) ;
#100936=AXIS2_PLACEMENT_3D ( 'NONE', #235127, #133455, #110032 ) ;
#100976=CARTESIAN_POINT ( 'NONE',  ( -18.69999999999999929, 0.000000000000000000, 0.000000000000000000 ) ) ;
#101019=DIRECTION ( 'NONE',  ( 1.645090726704136556E-14, -0.1618390714546045217, -0.9868171638914230437 ) ) ;
#101033=FACE_OUTER_BOUND ( 'NONE', #31900, .T. ) ;
#101060=DIRECTION ( 'NONE',  ( 0.000000000000000000, 0.000000000000000000, -1.000000000000000000 ) ) ;
#101122=VECTOR ( 'NONE', #233456, 1000.000000000000000 ) ;
#101136=EDGE_CURVE ( 'NONE', #99741, #126102, #192691, .T. ) ;
#101140=EDGE_LOOP ( 'NONE', ( #15854, #211432, #243980, #78208 ) ) ;
#101143=CARTESIAN_POINT ( 'NONE',  ( 18.59999999999999787, -11.65000000000000036, 5.900000000000001243 ) ) ;
#101160=ADVANCED_FACE ( 'NONE', ( #159398 ), #137249, .F. ) ;
#101176=EDGE_CURVE ( 'NONE', #49507, #168528, #4152, .T. ) ;
#101183=CIRCLE ( 'NONE', #238612, 4.000000000000000000 ) ;
#101244=DIRECTION ( 'NONE',  ( 0.000000000000000000, 0.000000000000000000, -1.000000000000000000 ) ) ;
#101265=SPHERICAL_SURFACE ( 'NONE', #247442, 0.1000000000000000056 ) ;
#101268=DIRECTION ( 'NONE',  ( 0.000000000000000000, 0.000000000000000000, 1.000000000000000000 ) ) ;
#101294=SPHERICAL_SURFACE ( 'NONE', #251679, 0.1000000000000000056 ) ;
#101341=ORIENTED_EDGE ( 'NONE', *, *, #256543, .F. ) ;
#101371=FACE_OUTER_BOUND ( 'NONE', #180239, .T. ) ;
#101374=FACE_OUTER_BOUND ( 'NONE', #1351, .T. ) ;
#101392=CARTESIAN_POINT ( 'NONE',  ( -21.00000000000000000, 7.973296578895943121, 1.410778198689825347 ) ) ;
#101403=ORIENTED_EDGE ( 'NONE', *, *, #178631, .T. ) ;
#101443=EDGE_LOOP ( 'NONE', ( #123316, #112660, #32283, #234580 ) ) ;
#101482=DIRECTION ( 'NONE',  ( 0.000000000000000000, 0.000000000000000000, -1.000000000000000000 ) ) ;
#101506=AXIS2_PLACEMENT_3D ( 'NONE', #95253, #133108, #11896 ) ;
#101508=CARTESIAN_POINT ( 'NONE',  ( -20.90000000000000213, 7.886648289447972360, 1.399104650876408451 ) ) ;
#101519=LINE ( 'NONE', #244916, #103935 ) ;
#101566=CARTESIAN_POINT ( 'NONE',  ( -18.79999999999999716, 5.586869315528661062, 16.41686199900910736 ) ) ;
#101579=FACE_OUTER_BOUND ( 'NONE', #174554, .T. ) ;
#101619=ORIENTED_EDGE ( 'NONE', *, *, #155840, .F. ) ;
#101636=EDGE_CURVE ( 'NONE', #70728, #82204, #226333, .T. ) ;
#101639=DIRECTION ( 'NONE',  ( 0.000000000000000000, 0.000000000000000000, 1.000000000000000000 ) ) ;
#101662=LINE ( 'NONE', #41750, #134914 ) ;
#101761=VERTEX_POINT ( 'NONE', #182512 ) ;
#101786=EDGE_LOOP ( 'NONE', ( #121825, #173393, #234177, #80200 ) ) ;
#101841=CIRCLE ( 'NONE', #235151, 0.1000000000000028644 ) ;
#101860=DIRECTION ( 'NONE',  ( -0.000000000000000000, 0.000000000000000000, 1.000000000000000000 ) ) ;
#101879=LINE ( 'NONE', #61507, #104539 ) ;
#101909=ORIENTED_EDGE ( 'NONE', *, *, #122122, .T. ) ;
#101931=ORIENTED_EDGE ( 'NONE', *, *, #185689, .F. ) ;
#101936=DIRECTION ( 'NONE',  ( -0.000000000000000000, -0.9910465087640865089, 0.1335171055202867274 ) ) ;
#101975=DIRECTION ( 'NONE',  ( 0.000000000000000000, 0.000000000000000000, 1.000000000000000000 ) ) ;
#101996=CARTESIAN_POINT ( 'NONE',  ( -20.09999999673964410, 4.627350251755220079, 22.02580456186781177 ) ) ;
#102007=DIRECTION ( 'NONE',  ( -1.000000000000000000, 0.000000000000000000, -0.000000000000000000 ) ) ;
#102048=ORIENTED_EDGE ( 'NONE', *, *, #167257, .F. ) ;
#102049=EDGE_LOOP ( 'NONE', ( #251793, #58628, #63624, #227421 ) ) ;
#102059=CARTESIAN_POINT ( 'NONE',  ( -22.10000000000000142, -3.262756495241484158E-15, 33.00000000000000000 ) ) ;
#102105=ADVANCED_FACE ( 'NONE', ( #23125 ), #101294, .T. ) ;
#102182=CARTESIAN_POINT ( 'NONE',  ( 18.59999999999999787, -10.72142460728770352, 6.051435706882140053 ) ) ;
#102299=DIRECTION ( 'NONE',  ( 0.000000000000000000, 0.000000000000000000, -1.000000000000000000 ) ) ;
#102329=EDGE_CURVE ( 'NONE', #200951, #73306, #214269, .T. ) ;
#102424=ORIENTED_EDGE ( 'NONE', *, *, #172448, .T. ) ;
#102460=TOROIDAL_SURFACE ( 'NONE', #110693, 0.2000000000000000111, 0.1000000000000000056 ) ;
#102494=DIRECTION ( 'NONE',  ( 1.000000000000000000, 0.000000000000000000, 0.000000000000000000 ) ) ;
#102512=CARTESIAN_POINT ( 'NONE',  ( 19.90000000000000213, 5.572646938319268273, 16.50000000000000000 ) ) ;
#102514=DIRECTION ( 'NONE',  ( -0.000000000000000000, 1.000000000000000000, -0.000000000000000000 ) ) ;
#102530=EDGE_CURVE ( 'NONE', #11158, #89225, #231031, .T. ) ;
#102546=ORIENTED_EDGE ( 'NONE', *, *, #173328, .F. ) ;
#102607=FACE_OUTER_BOUND ( 'NONE', #57213, .T. ) ;
#102624=CARTESIAN_POINT ( 'NONE',  ( 18.69999999999999929, -10.84999999999999076, 31.50000000000000000 ) ) ;
#102627=CARTESIAN_POINT ( 'NONE',  ( -19.89999999999999858, 1.350000000000000089, 16.50000000000000000 ) ) ;
#102629=CARTESIAN_POINT ( 'NONE',  ( 13.40000000000000036, -8.350000000000004974, 10.95857864376269397 ) ) ;
#102632=CARTESIAN_POINT ( 'NONE',  ( 20.00000000000000355, 5.454087299794355914, 16.60000000000000142 ) ) ;
#102658=ORIENTED_EDGE ( 'NONE', *, *, #255799, .T. ) ;
#102715=( BOUNDED_CURVE ( )  B_SPLINE_CURVE ( 3, ( #145009, #184142, #165900, #242836 ),
 .UNSPECIFIED., .F., .T. ) 
 B_SPLINE_CURVE_WITH_KNOTS ( ( 4, 4 ),
 ( 0.000000000000000000, 1.570796326794895892 ),
 .UNSPECIFIED. ) 
 CURVE ( )  GEOMETRIC_REPRESENTATION_ITEM ( )  RATIONAL_B_SPLINE_CURVE ( ( 1.000000000000000000, 0.8047378541243652705, 0.8047378541243652705, 1.000000000000000000 ) ) 
 REPRESENTATION_ITEM ( '' )  );
#102722=VERTEX_POINT ( 'NONE', #157883 ) ;
#102733=SPHERICAL_SURFACE ( 'NONE', #172352, 0.1000000000000000056 ) ;
#102843=CARTESIAN_POINT ( 'NONE',  ( -18.69999999999999929, 1.212568896937007645, -7.800000000000000711 ) ) ;
#102867=CARTESIAN_POINT ( 'NONE',  ( 22.19999999999999929, -11.65000000000000036, -15.00000000000000000 ) ) ;
#102875=EDGE_CURVE ( 'NONE', #176716, #130825, #258051, .T. ) ;
#102889=VERTEX_POINT ( 'NONE', #84667 ) ;
#102937=DIRECTION ( 'NONE',  ( 0.000000000000000000, 0.000000000000000000, 1.000000000000000000 ) ) ;
#102958=AXIS2_PLACEMENT_3D ( 'NONE', #178583, #79429, #61169 ) ;
#103041=ORIENTED_EDGE ( 'NONE', *, *, #125729, .T. ) ;
#103062=ORIENTED_EDGE ( 'NONE', *, *, #90035, .T. ) ;
#103087=CARTESIAN_POINT ( 'NONE',  ( -18.59999999999999787, 11.75000000000000000, 31.50000000000000000 ) ) ;
#103097=DIRECTION ( 'NONE',  ( 1.000000000000000000, -0.000000000000000000, -0.000000000000000000 ) ) ;
#103122=AXIS2_PLACEMENT_3D ( 'NONE', #8156, #242900, #227186 ) ;
#103147=DIRECTION ( 'NONE',  ( -1.000000000000000000, 0.000000000000000000, -0.000000000000000000 ) ) ;
#103172=ADVANCED_FACE ( 'NONE', ( #94972 ), #255278, .T. ) ;
#103225=LINE ( 'NONE', #58952, #92587 ) ;
#103287=FACE_OUTER_BOUND ( 'NONE', #139223, .T. ) ;
#103305=CARTESIAN_POINT ( 'NONE',  ( -18.79999999999999716, 0.000000000000000000, 0.000000000000000000 ) ) ;
#103363=ORIENTED_EDGE ( 'NONE', *, *, #52792, .T. ) ;
#103380=CYLINDRICAL_SURFACE ( 'NONE', #92441, 0.09999999999999939493 ) ;
#103394=EDGE_CURVE ( 'NONE', #6846, #71198, #239756, .T. ) ;
#103421=CARTESIAN_POINT ( 'NONE',  ( 18.59999999999999787, -10.74999999999999289, 32.89999999999999858 ) ) ;
#103430=VECTOR ( 'NONE', #89450, 1000.000000000000000 ) ;
#103440=DIRECTION ( 'NONE',  ( -0.000000000000000000, 1.000000000000000000, -0.000000000000000000 ) ) ;
#103466=AXIS2_PLACEMENT_3D ( 'NONE', #178956, #237614, #160667 ) ;
#103469=VERTEX_POINT ( 'NONE', #110371 ) ;
#103482=SPHERICAL_SURFACE ( 'NONE', #200624, 0.1000000000000000056 ) ;
#103483=VERTEX_POINT ( 'NONE', #129925 ) ;
#103505=EDGE_CURVE ( 'NONE', #244339, #253988, #56384, .T. ) ;
#103525=FACE_OUTER_BOUND ( 'NONE', #75005, .T. ) ;
#103546=ORIENTED_EDGE ( 'NONE', *, *, #21163, .F. ) ;
#103575=CIRCLE ( 'NONE', #249361, 0.09999999999999939493 ) ;
#103588=VERTEX_POINT ( 'NONE', #175515 ) ;
#103593=EDGE_CURVE ( 'NONE', #186764, #26765, #51897, .T. ) ;
#103701=EDGE_CURVE ( 'NONE', #84718, #256719, #181914, .T. ) ;
#103726=DIRECTION ( 'NONE',  ( -1.000000000000000000, 0.000000000000000000, 0.000000000000000000 ) ) ;
#103731=DIRECTION ( 'NONE',  ( -1.000000000000000000, 0.000000000000000000, 0.000000000000000000 ) ) ;
#103732=DIRECTION ( 'NONE',  ( 0.000000000000000000, 0.000000000000000000, 1.000000000000000000 ) ) ;
#103743=ORIENTED_EDGE ( 'NONE', *, *, #108779, .F. ) ;
#103763=FILL_AREA_STYLE_COLOUR ( '', #81715 ) ;
#103786=DIRECTION ( 'NONE',  ( 1.000000000000000000, 0.000000000000000000, 0.000000000000000000 ) ) ;
#103804=EDGE_CURVE ( 'NONE', #10810, #48863, #47514, .T. ) ;
#103825=ADVANCED_FACE ( 'NONE', ( #170095 ), #249597, .T. ) ;
#103836=AXIS2_PLACEMENT_3D ( 'NONE', #55440, #228987, #210697 ) ;
#103837=ORIENTED_EDGE ( 'NONE', *, *, #72673, .F. ) ;
#103844=AXIS2_PLACEMENT_3D ( 'NONE', #179195, #504, #176615 ) ;
#103899=ORIENTED_EDGE ( 'NONE', *, *, #59997, .F. ) ;
#103935=VECTOR ( 'NONE', #44166, 1000.000000000000000 ) ;
#103947=CARTESIAN_POINT ( 'NONE',  ( -18.69999999999999929, -9.749999999999996447, 31.39999999999999858 ) ) ;
#103980=ORIENTED_EDGE ( 'NONE', *, *, #173899, .T. ) ;
#104008=EDGE_CURVE ( 'NONE', #150585, #254139, #44050, .T. ) ;
#104069=ORIENTED_EDGE ( 'NONE', *, *, #233015, .F. ) ;
#104080=DIRECTION ( 'NONE',  ( 4.336808689942017736E-16, -0.000000000000000000, 1.000000000000000000 ) ) ;
#104091=EDGE_CURVE ( 'NONE', #18932, #225036, #10421, .T. ) ;
#104097=CARTESIAN_POINT ( 'NONE',  ( -18.79999999999999716, 11.49641995933507843, 1.885425182446135883 ) ) ;
#104124=CARTESIAN_POINT ( 'NONE',  ( -20.90000000000000213, 0.000000000000000000, 0.000000000000000000 ) ) ;
#104167=EDGE_CURVE ( 'NONE', #241189, #157564, #191292, .T. ) ;
#104256=CARTESIAN_POINT ( 'NONE',  ( -18.79999999999999716, 11.49641995933507843, -1.885425182446133885 ) ) ;
#104294=CIRCLE ( 'NONE', #112518, 11.75000000000000000 ) ;
#104300=DIRECTION ( 'NONE',  ( 1.000000000000000000, 0.000000000000000000, 0.000000000000000000 ) ) ;
#104326=EDGE_CURVE ( 'NONE', #194632, #107433, #68881, .T. ) ;
#104361=CARTESIAN_POINT ( 'NONE',  ( 20.90000000000000213, 1.800000000000000044, -11.61130914238355771 ) ) ;
#104419=PLANE ( 'NONE',  #253629 ) ;
#104433=CARTESIAN_POINT ( 'NONE',  ( 20.10000000000000853, 4.625944962820097039, 22.03401928653448749 ) ) ;
#104480=CARTESIAN_POINT ( 'NONE',  ( 21.00000000000000000, -0.3305886640091971196, 0.04453801223857078301 ) ) ;
#104497=CARTESIAN_POINT ( 'NONE',  ( 22.10000000000000142, -11.65000000000000036, 12.09999999999999609 ) ) ;
#104534=CARTESIAN_POINT ( 'NONE',  ( 18.59999999999999787, -11.65000000000000036, 29.89999999999999858 ) ) ;
#104538=CARTESIAN_POINT ( 'NONE',  ( -6.000000000000003553, -11.65000000000000036, 10.10000000000000142 ) ) ;
#104539=VECTOR ( 'NONE', #141047, 1000.000000000000000 ) ;
#104540=VERTEX_POINT ( 'NONE', #112710 ) ;
#104566=DIRECTION ( 'NONE',  ( 0.000000000000000000, 0.000000000000000000, 1.000000000000000000 ) ) ;
#104619=DIRECTION ( 'NONE',  ( 0.000000000000000000, 0.000000000000000000, -1.000000000000000000 ) ) ;
#104632=ORIENTED_EDGE ( 'NONE', *, *, #7332, .F. ) ;
#104642=CARTESIAN_POINT ( 'NONE',  ( -37.88850191057539973, -10.64999999999999325, 31.59999999999999787 ) ) ;
#104646=ORIENTED_EDGE ( 'NONE', *, *, #52792, .F. ) ;
#104677=DIRECTION ( 'NONE',  ( -0.000000000000000000, 1.000000000000000000, 0.000000000000000000 ) ) ;
#104721=CYLINDRICAL_SURFACE ( 'NONE', #27130, 0.09999999999999990841 ) ;
#104751=DIRECTION ( 'NONE',  ( 0.000000000000000000, 2.168404344971021884E-15, -1.000000000000000000 ) ) ;
#104760=CARTESIAN_POINT ( 'NONE',  ( 21.00000000000000000, 0.000000000000000000, 0.000000000000000000 ) ) ;
#104787=DIRECTION ( 'NONE',  ( 0.000000000000000000, -1.156482317317873105E-15, 1.000000000000000000 ) ) ;
#104792=DIRECTION ( 'NONE',  ( 0.000000000000000000, 0.7071067811865472397, -0.7071067811865479058 ) ) ;
#104855=EDGE_CURVE ( 'NONE', #46601, #194632, #72002, .T. ) ;
#104913=ORIENTED_EDGE ( 'NONE', *, *, #104326, .T. ) ;
#104920=ORIENTED_EDGE ( 'NONE', *, *, #122782, .F. ) ;
#104957=ORIENTED_EDGE ( 'NONE', *, *, #179314, .F. ) ;
#105035=AXIS2_PLACEMENT_3D ( 'NONE', #46972, #26164, #10447 ) ;
#105043=CARTESIAN_POINT ( 'NONE',  ( 18.69999999999999929, -1.212568896937008089, -8.000000000000000000 ) ) ;
#105056=ORIENTED_EDGE ( 'NONE', *, *, #26671, .F. ) ;
#105114=DIRECTION ( 'NONE',  ( 0.000000000000000000, 1.000000000000000000, 0.000000000000000000 ) ) ;
#105214=ORIENTED_EDGE ( 'NONE', *, *, #103804, .T. ) ;
#105217=ORIENTED_EDGE ( 'NONE', *, *, #23162, .F. ) ;
#105250=CARTESIAN_POINT ( 'NONE',  ( -18.79999999999999716, 7.900000000000000355, -1.300000000000000044 ) ) ;
#105298=ORIENTED_EDGE ( 'NONE', *, *, #179087, .T. ) ;
#105323=ORIENTED_EDGE ( 'NONE', *, *, #225918, .T. ) ;
#105355=ORIENTED_EDGE ( 'NONE', *, *, #253681, .T. ) ;
#105362=DIRECTION ( 'NONE',  ( 0.000000000000000000, 0.000000000000000000, 1.000000000000000000 ) ) ;
#105372=ORIENTED_EDGE ( 'NONE', *, *, #211857, .T. ) ;
#105377=VECTOR ( 'NONE', #34773, 1000.000000000000000 ) ;
#105384=EDGE_LOOP ( 'NONE', ( #85281, #28092, #115923, #106324 ) ) ;
#105396=CIRCLE ( 'NONE', #176189, 0.09999999999999939493 ) ;
#105403=DIRECTION ( 'NONE',  ( 0.000000000000000000, 1.000000000000000000, 0.000000000000000000 ) ) ;
#105406=ORIENTED_EDGE ( 'NONE', *, *, #113828, .F. ) ;
#105508=CIRCLE ( 'NONE', #180561, 0.09999999999999939493 ) ;
#105525=ORIENTED_EDGE ( 'NONE', *, *, #185533, .F. ) ;
#105551=FACE_OUTER_BOUND ( 'NONE', #115255, .T. ) ;
#105564=VERTEX_POINT ( 'NONE', #227544 ) ;
#105612=ORIENTED_EDGE ( 'NONE', *, *, #226241, .F. ) ;
#105629=DIRECTION ( 'NONE',  ( 0.000000000000000000, 0.000000000000000000, -1.000000000000000000 ) ) ;
#105678=VERTEX_POINT ( 'NONE', #95724 ) ;
#105706=DIRECTION ( 'NONE',  ( -1.000000000000000000, -0.000000000000000000, -0.000000000000000000 ) ) ;
#105720=CIRCLE ( 'NONE', #5762, 0.1000000000000028644 ) ;
#105780=( BOUNDED_CURVE ( )  B_SPLINE_CURVE ( 3, ( #246034, #225154, #122237, #102632 ),
 .UNSPECIFIED., .F., .F. ) 
 B_SPLINE_CURVE_WITH_KNOTS ( ( 4, 4 ),
 ( 0.000000000000000000, 1.570796326794891229 ),
 .UNSPECIFIED. ) 
 CURVE ( )  GEOMETRIC_REPRESENTATION_ITEM ( )  RATIONAL_B_SPLINE_CURVE ( ( 1.000000000000000000, 0.8047378541243662697, 0.8047378541243662697, 1.000000000000000000 ) ) 
 REPRESENTATION_ITEM ( '' )  );
#105786=DIRECTION ( 'NONE',  ( 0.000000000000000000, 1.000000000000000000, 0.000000000000000000 ) ) ;
#105815=CIRCLE ( 'NONE', #251584, 0.09999999999999982514 ) ;
#105846=VECTOR ( 'NONE', #172588, 1000.000000000000000 ) ;
#105850=CARTESIAN_POINT ( 'NONE',  ( 20.90000000000000213, 11.49641995933507843, 1.885425182446133885 ) ) ;
#105855=CARTESIAN_POINT ( 'NONE',  ( -19.89999999999999503, 4.631764625546185066, 22.00000000000000355 ) ) ;
#105858=DIRECTION ( 'NONE',  ( 1.000000000000000000, 0.000000000000000000, 0.000000000000000000 ) ) ;
#105862=CARTESIAN_POINT ( 'NONE',  ( 20.90000000000000213, -1.901609089591594470, -11.59510167572422112 ) ) ;
#105931=EDGE_CURVE ( 'NONE', #28188, #204919, #7204, .T. ) ;
#105941=AXIS2_PLACEMENT_3D ( 'NONE', #34117, #35399, #94038 ) ;
#105944=VERTEX_POINT ( 'NONE', #103421 ) ;
#105946=DIRECTION ( 'NONE',  ( -1.000000000000000000, -1.476360405086644309E-16, 0.000000000000000000 ) ) ;
#105966=CARTESIAN_POINT ( 'NONE',  ( 22.10000000000000142, -11.75000000000000355, 12.09999999999999609 ) ) ;
#105974=CARTESIAN_POINT ( 'NONE',  ( 19.90000000000000924, 4.513204987021262937, 22.00000000000000355 ) ) ;
#106026=VERTEX_POINT ( 'NONE', #113721 ) ;
#106122=DIRECTION ( 'NONE',  ( -0.000000000000000000, 0.000000000000000000, 1.000000000000000000 ) ) ;
#106160=VECTOR ( 'NONE', #66767, 1000.000000000000114 ) ;
#106217=DIRECTION ( 'NONE',  ( 1.284434275755705296E-16, -0.7071067811865471286, 0.7071067811865479058 ) ) ;
#106224=EDGE_LOOP ( 'NONE', ( #127850, #183176, #205737 ) ) ;
#106225=EDGE_CURVE ( 'NONE', #156269, #248318, #15648, .T. ) ;
#106228=LINE ( 'NONE', #209198, #120174 ) ;
#106271=CARTESIAN_POINT ( 'NONE',  ( -18.69999999999999929, -8.150000000000005684, 10.52591260281975138 ) ) ;
#106292=CIRCLE ( 'NONE', #122912, 0.09999999999999939493 ) ;
#106306=DIRECTION ( 'NONE',  ( 0.000000000000000000, 0.000000000000000000, 1.000000000000000000 ) ) ;
#106322=DIRECTION ( 'NONE',  ( 0.000000000000000000, 1.000000000000000000, -0.000000000000000000 ) ) ;
#106324=ORIENTED_EDGE ( 'NONE', *, *, #31853, .F. ) ;
#106343=ORIENTED_EDGE ( 'NONE', *, *, #78130, .F. ) ;
#106344=TOROIDAL_SURFACE ( 'NONE', #93902, 0.2000000000000000111, 0.1000000000000000056 ) ;
#106382=EDGE_LOOP ( 'NONE', ( #48257, #678, #217896, #182097 ) ) ;
#106426=ADVANCED_FACE ( 'NONE', ( #31355 ), #76850, .F. ) ;
#106449=DIRECTION ( 'NONE',  ( -1.000000000000000000, 0.000000000000000000, 0.000000000000000000 ) ) ;
#106460=DIRECTION ( 'NONE',  ( 0.000000000000000000, 0.1335171055202867274, 0.9910465087640866200 ) ) ;
#106503=ORIENTED_EDGE ( 'NONE', *, *, #96461, .F. ) ;
#106544=EDGE_CURVE ( 'NONE', #91499, #88476, #65847, .T. ) ;
#106563=DIRECTION ( 'NONE',  ( 0.000000000000000000, 0.000000000000000000, -1.000000000000000000 ) ) ;
#106580=VERTEX_POINT ( 'NONE', #224056 ) ;
#106587=CARTESIAN_POINT ( 'NONE',  ( 18.69999999999999929, -8.350000000000004974, 21.95857864376268864 ) ) ;
#106592=CARTESIAN_POINT ( 'NONE',  ( 11.60000000000000142, -8.250000000000005329, 19.04142135623731136 ) ) ;
#106609=ORIENTED_EDGE ( 'NONE', *, *, #58498, .T. ) ;
#106636=EDGE_LOOP ( 'NONE', ( #181510, #207027, #181673 ) ) ;
#106652=( NAMED_UNIT ( * ) PLANE_ANGLE_UNIT ( ) SI_UNIT ( $, .RADIAN. ) );
#106665=CARTESIAN_POINT ( 'NONE',  ( -18.69999999999999929, -11.65000000000000036, 5.900000000000001243 ) ) ;
#106693=CARTESIAN_POINT ( 'NONE',  ( 18.59999999999999787, -14.27107483842559610, -0.5438473119858301397 ) ) ;
#106710=ORIENTED_EDGE ( 'NONE', *, *, #123004, .T. ) ;
#106711=FACE_OUTER_BOUND ( 'NONE', #238077, .T. ) ;
#106731=CARTESIAN_POINT ( 'NONE',  ( -5.900000000000005684, -11.25000000000000000, 1.279358563532896415E-15 ) ) ;
#106790=TOROIDAL_SURFACE ( 'NONE', #140096, 0.2000000000000000111, 0.1000000000000000056 ) ;
#106804=CARTESIAN_POINT ( 'NONE',  ( -18.60000000000000142, -8.150000000000005684, -15.00000000000000000 ) ) ;
#106839=DIRECTION ( 'NONE',  ( 0.000000000000000000, 0.000000000000000000, 1.000000000000000000 ) ) ;
#106860=ORIENTED_EDGE ( 'NONE', *, *, #34248, .T. ) ;
#106863=PLANE ( 'NONE',  #90659 ) ;
#106882=DIRECTION ( 'NONE',  ( -1.000000000000000000, 0.000000000000000000, 0.000000000000000000 ) ) ;
#106932=EDGE_LOOP ( 'NONE', ( #160242, #174039, #42045, #147524 ) ) ;
#106955=SPHERICAL_SURFACE ( 'NONE', #105035, 0.1000000000000000056 ) ;
#106959=EDGE_CURVE ( 'NONE', #232547, #67059, #64680, .T. ) ;
#106971=ADVANCED_FACE ( 'NONE', ( #4690 ), #5977, .T. ) ;
#106995=DIRECTION ( 'NONE',  ( 0.000000000000000000, 0.000000000000000000, 1.000000000000000000 ) ) ;
#107037=CIRCLE ( 'NONE', #236229, 0.09999999999999939493 ) ;
#107069=EDGE_CURVE ( 'NONE', #179078, #48863, #128586, .T. ) ;
#107115=VECTOR ( 'NONE', #213778, 1000.000000000000000 ) ;
#107118=DIRECTION ( 'NONE',  ( 0.000000000000000000, 0.000000000000000000, -1.000000000000000000 ) ) ;
#107160=DIRECTION ( 'NONE',  ( 0.000000000000000000, 0.000000000000000000, -1.000000000000000000 ) ) ;
#107165=EDGE_LOOP ( 'NONE', ( #208961, #144810, #195142, #117128 ) ) ;
#107169=DIRECTION ( 'NONE',  ( -1.000000000000000000, -0.000000000000000000, -0.000000000000000000 ) ) ;
#107259=CIRCLE ( 'NONE', #153098, 0.09999999999999939493 ) ;
#107277=CYLINDRICAL_SURFACE ( 'NONE', #216112, 0.09999999999999939493 ) ;
#107284=DIRECTION ( 'NONE',  ( 0.000000000000000000, 0.000000000000000000, -1.000000000000000000 ) ) ;
#107301=VECTOR ( 'NONE', #241514, 1000.000000000000000 ) ;
#107361=AXIS2_PLACEMENT_3D ( 'NONE', #117574, #160587, #18477 ) ;
#107397=DIRECTION ( 'NONE',  ( 0.000000000000000000, 0.000000000000000000, 1.000000000000000000 ) ) ;
#107418=CARTESIAN_POINT ( 'NONE',  ( 18.79999999999999716, 1.350000000000000089, 16.60000000000000142 ) ) ;
#107433=VERTEX_POINT ( 'NONE', #178453 ) ;
#107445=LINE ( 'NONE', #33096, #114514 ) ;
#107514=DIRECTION ( 'NONE',  ( 0.000000000000000000, 0.000000000000000000, -1.000000000000000000 ) ) ;
#107536=DIRECTION ( 'NONE',  ( 0.000000000000000000, 1.224646799147353207E-16, 1.000000000000000000 ) ) ;
#107556=CARTESIAN_POINT ( 'NONE',  ( -22.84999999999999787, 4.776122516674678272E-16, -3.900000000000000355 ) ) ;
#107558=AXIS2_PLACEMENT_3D ( 'NONE', #235159, #176482, #56490 ) ;
#107606=CARTESIAN_POINT ( 'NONE',  ( 11.60000000000000320, -9.650000000000002132, 12.40000000000000391 ) ) ;
#107612=DIRECTION ( 'NONE',  ( -1.000000000000000000, 0.000000000000000000, 0.000000000000000000 ) ) ;
#107619=CIRCLE ( 'NONE', #11811, 0.1000000000000000472 ) ;
#107640=CIRCLE ( 'NONE', #20174, 0.09999999999999939493 ) ;
#107671=EDGE_CURVE ( 'NONE', #203823, #150529, #89658, .T. ) ;
#107720=ADVANCED_FACE ( 'NONE', ( #32298 ), #154815, .T. ) ;
#107783=DIRECTION ( 'NONE',  ( 0.000000000000000000, 0.000000000000000000, 1.000000000000000000 ) ) ;
#107822=DIRECTION ( 'NONE',  ( -1.000000000000000000, 0.000000000000000000, -0.000000000000000000 ) ) ;
#107857=CARTESIAN_POINT ( 'NONE',  ( -20.90000000000000213, -1.885425182446133885, -11.49641995933507843 ) ) ;
#107865=AXIS2_PLACEMENT_3D ( 'NONE', #213581, #50643, #194049 ) ;
#107882=ORIENTED_EDGE ( 'NONE', *, *, #111758, .F. ) ;
#107889=DIRECTION ( 'NONE',  ( 0.000000000000000000, 0.000000000000000000, 1.000000000000000000 ) ) ;
#107895=LINE ( 'NONE', #207002, #84128 ) ;
#107920=DIRECTION ( 'NONE',  ( 0.000000000000000000, -1.000000000000000000, 0.000000000000000000 ) ) ;
#107948=CARTESIAN_POINT ( 'NONE',  ( 18.79999999999999716, 1.350000000000000089, 22.10000000000000142 ) ) ;
#108003=FACE_OUTER_BOUND ( 'NONE', #88932, .T. ) ;
#108017=MANIFOLD_SOLID_BREP ( 'Stock-MAS-200-1', #74159 ) ;
#108033=CARTESIAN_POINT ( 'NONE',  ( -18.69999999999999929, -8.250000000000005329, -7.800000000000000711 ) ) ;
#108034=CARTESIAN_POINT ( 'NONE',  ( -21.00000000000000000, 7.973296578895943121, -1.410778198689825347 ) ) ;
#108092=VECTOR ( 'NONE', #111868, 1000.000000000000000 ) ;
#108138=AXIS2_PLACEMENT_3D ( 'NONE', #257388, #215742, #254826 ) ;
#108140=CARTESIAN_POINT ( 'NONE',  ( -0.8999999999999993561, -8.250000000000005329, 26.00000000000000355 ) ) ;
#108152=ORIENTED_EDGE ( 'NONE', *, *, #164491, .T. ) ;
#108176=DIRECTION ( 'NONE',  ( 1.000000000000000000, 0.000000000000000000, 0.000000000000000000 ) ) ;
#108180=EDGE_LOOP ( 'NONE', ( #115477, #139936, #226991, #68278 ) ) ;
#108217=DIRECTION ( 'NONE',  ( 0.000000000000000000, 0.000000000000000000, 1.000000000000000000 ) ) ;
#108222=LINE ( 'NONE', #224307, #113292 ) ;
#108245=CYLINDRICAL_SURFACE ( 'NONE', #160244, 11.75000000000000000 ) ;
#108282=AXIS2_PLACEMENT_3D ( 'NONE', #203405, #142134, #121334 ) ;
#108294=DIRECTION ( 'NONE',  ( 0.000000000000000000, -1.000000000000000000, 0.000000000000000000 ) ) ;
#108339=DIRECTION ( 'NONE',  ( 1.476360405086644309E-16, 1.000000000000000000, 0.000000000000000000 ) ) ;
#108346=CIRCLE ( 'NONE', #29273, 0.09999999999999939493 ) ;
#108408=CYLINDRICAL_SURFACE ( 'NONE', #185784, 0.1000000000000002554 ) ;
#108433=EDGE_LOOP ( 'NONE', ( #254824, #182582, #171171 ) ) ;
#108456=CARTESIAN_POINT ( 'NONE',  ( -11.60000000000000320, -11.65000000000000036, 17.70000000000000639 ) ) ;
#108458=CARTESIAN_POINT ( 'NONE',  ( -22.94999999999999929, 8.000000000000000000, -1.212568896937008089 ) ) ;
#108472=LINE ( 'NONE', #88886, #194668 ) ;
#108476=DIRECTION ( 'NONE',  ( 0.000000000000000000, 1.000000000000000000, 0.000000000000000000 ) ) ;
#108514=EDGE_CURVE ( 'NONE', #33376, #158009, #87759, .T. ) ;
#108582=VERTEX_POINT ( 'NONE', #139401 ) ;
#108595=DIRECTION ( 'NONE',  ( 1.000000000000000000, -0.000000000000000000, -0.000000000000000000 ) ) ;
#108633=ADVANCED_FACE ( 'NONE', ( #98977 ), #236245, .F. ) ;
#108658=DIRECTION ( 'NONE',  ( 0.000000000000000000, 0.000000000000000000, -1.000000000000000000 ) ) ;
#108659=DIRECTION ( 'NONE',  ( 0.000000000000000000, 0.000000000000000000, 1.000000000000000000 ) ) ;
#108688=CARTESIAN_POINT ( 'NONE',  ( -22.10000000000000497, 6.223900101154156594, 12.00000000000000000 ) ) ;
#108709=AXIS2_PLACEMENT_3D ( 'NONE', #110629, #231885, #188887 ) ;
#108710=CARTESIAN_POINT ( 'NONE',  ( 18.69999999999999929, -10.64999999999999325, 31.59999999999999787 ) ) ;
#108711=FACE_OUTER_BOUND ( 'NONE', #27335, .T. ) ;
#108779=EDGE_CURVE ( 'NONE', #107433, #78394, #89704, .T. ) ;
#108785=EDGE_CURVE ( 'NONE', #168244, #99187, #198646, .T. ) ;
#108822=CARTESIAN_POINT ( 'NONE',  ( 20.90000000000000213, 3.362550747017865493, 28.82623795144604983 ) ) ;
#108825=DIRECTION ( 'NONE',  ( -1.000000000000000000, 0.000000000000000000, -0.000000000000000000 ) ) ;
#108833=DIRECTION ( 'NONE',  ( -1.000000000000000000, -0.000000000000000000, -0.000000000000000000 ) ) ;
#108885=CARTESIAN_POINT ( 'NONE',  ( -18.79999999999999716, 1.885425182446133663, -11.49641995933507665 ) ) ;
#108896=CARTESIAN_POINT ( 'NONE',  ( -5.900000000000002132, -11.25000000000000000, 13.90000000000000213 ) ) ;
#108921=EDGE_LOOP ( 'NONE', ( #200148, #14698, #224732, #38964 ) ) ;
#108930=DIRECTION ( 'NONE',  ( 0.000000000000000000, 0.000000000000000000, -1.000000000000000000 ) ) ;
#108959=EDGE_CURVE ( 'NONE', #192900, #141175, #40480, .T. ) ;
#108966=CARTESIAN_POINT ( 'NONE',  ( -13.40000000000000213, -8.250000000000007105, 15.00000000000000355 ) ) ;
#109003=DIRECTION ( 'NONE',  ( -0.000000000000000000, -0.9868171638914230437, 0.1618390714546045217 ) ) ;
#109026=ADVANCED_FACE ( 'NONE', ( #80386 ), #60847, .T. ) ;
#109055=DIRECTION ( 'NONE',  ( 1.000000000000000000, 0.000000000000000000, 0.000000000000000000 ) ) ;
#109113=DIRECTION ( 'NONE',  ( -1.284434275755705789E-16, 0.7071067811865472397, -0.7071067811865479058 ) ) ;
#109197=ORIENTED_EDGE ( 'NONE', *, *, #212768, .T. ) ;
#109237=ORIENTED_EDGE ( 'NONE', *, *, #176025, .T. ) ;
#109239=CARTESIAN_POINT ( 'NONE',  ( 18.69999999999999929, 0.000000000000000000, 0.000000000000000000 ) ) ;
#109297=LINE ( 'NONE', #106731, #170854 ) ;
#109299=CARTESIAN_POINT ( 'NONE',  ( 22.10000000000000497, -11.65000000000000036, -15.00000000000000000 ) ) ;
#109320=AXIS2_PLACEMENT_3D ( 'NONE', #232803, #35885, #77526 ) ;
#109340=ORIENTED_EDGE ( 'NONE', *, *, #247380, .F. ) ;
#109353=EDGE_LOOP ( 'NONE', ( #125576, #233217, #6463, #248161 ) ) ;
#109354=CYLINDRICAL_SURFACE ( 'NONE', #24756, 0.1000000000000002554 ) ;
#109382=PLANE ( 'NONE',  #143314 ) ;
#109386=CYLINDRICAL_SURFACE ( 'NONE', #95338, 0.09999999999999982514 ) ;
#109487=VERTEX_POINT ( 'NONE', #143928 ) ;
#109502=AXIS2_PLACEMENT_3D ( 'NONE', #107948, #66260, #87078 ) ;
#109505=VERTEX_POINT ( 'NONE', #12157 ) ;
#109524=LINE ( 'NONE', #70456, #225895 ) ;
#109548=( BOUNDED_SURFACE ( )  B_SPLINE_SURFACE ( 3, 2, ( 
 ( #244101, #167178, #65467 ),
 ( #101996, #45909, #246665 ),
 ( #68037, #125455, #26357 ),
 ( #181590, #105855, #86291 ) ),
 .UNSPECIFIED., .F., .F., .F. ) 
 B_SPLINE_SURFACE_WITH_KNOTS ( ( 4, 4 ),
 ( 3, 3 ),
 ( 1.570796326794896558, 3.141592653589793116 ),
 ( 0.000000000000000000, 1.000000000000000000 ),
 .UNSPECIFIED. ) 
 GEOMETRIC_REPRESENTATION_ITEM ( )  RATIONAL_B_SPLINE_SURFACE ( (
 ( 1.000000000000000000, 0.7071067811865475727, 1.000000000000000000),
 ( 1.000000000000000000, 0.6753870962079413509, 1.000000000000000000),
 ( 1.000000000000000000, 0.6438648806865591157, 1.000000000000000000),
 ( 1.000000000000000000, 0.6447402616204922499, 1.000000000000000000) ) ) 
 REPRESENTATION_ITEM ( '' )  SURFACE ( )  );
#109553=AXIS2_PLACEMENT_3D ( 'NONE', #176051, #76913, #237289 ) ;
#109560=CIRCLE ( 'NONE', #138751, 0.09999999999999939493 ) ;
#109566=CARTESIAN_POINT ( 'NONE',  ( -21.00000000000000000, 11.49641995933507843, 1.885425182446133885 ) ) ;
#109572=DIRECTION ( 'NONE',  ( 0.000000000000000000, 0.000000000000000000, -1.000000000000000000 ) ) ;
#109578=CARTESIAN_POINT ( 'NONE',  ( -13.40000000000000213, -8.250000000000005329, 19.04142135623731491 ) ) ;
#109588=CARTESIAN_POINT ( 'NONE',  ( -22.10000000000000142, -3.262756495241484158E-15, 32.89999999999999858 ) ) ;
#109599=CARTESIAN_POINT ( 'NONE',  ( 20.10000000000000853, 4.645987002755569861, 21.91686199900910736 ) ) ;
#109743=ORIENTED_EDGE ( 'NONE', *, *, #114815, .F. ) ;
#109753=DIRECTION ( 'NONE',  ( 1.000000000000000000, 0.000000000000000000, 0.000000000000000000 ) ) ;
#109756=CARTESIAN_POINT ( 'NONE',  ( -18.59999999999999787, -11.75000000000000000, 30.09999999999999787 ) ) ;
#109758=AXIS2_PLACEMENT_3D ( 'NONE', #209569, #169188, #70084 ) ;
#109776=DIRECTION ( 'NONE',  ( 0.000000000000000000, -0.000000000000000000, -1.000000000000000000 ) ) ;
#109784=CIRCLE ( 'NONE', #159886, 0.1000000000000028644 ) ;
#109809=ORIENTED_EDGE ( 'NONE', *, *, #189737, .F. ) ;
#109826=ORIENTED_EDGE ( 'NONE', *, *, #139046, .F. ) ;
#109856=AXIS2_PLACEMENT_3D ( 'NONE', #86365, #130656, #248038 ) ;
#109914=VERTEX_POINT ( 'NONE', #182774 ) ;
#109919=DIRECTION ( 'NONE',  ( 0.000000000000000000, 0.000000000000000000, 1.000000000000000000 ) ) ;
#109965=CYLINDRICAL_SURFACE ( 'NONE', #124702, 0.09999999999999939493 ) ;
#109973=ORIENTED_EDGE ( 'NONE', *, *, #45197, .T. ) ;
#109975=TOROIDAL_SURFACE ( 'NONE', #214039, 0.2000000000000000111, 0.1000000000000000056 ) ;
#109983=EDGE_LOOP ( 'NONE', ( #214144, #123674, #68292, #153530 ) ) ;
#110001=EDGE_LOOP ( 'NONE', ( #249704, #246719, #121596, #72983 ) ) ;
#110007=CARTESIAN_POINT ( 'NONE',  ( 18.69999999999999929, -2.105948478070175156, -13.13328020565119125 ) ) ;
#110016=EDGE_CURVE ( 'NONE', #47140, #256719, #174306, .T. ) ;
#110032=DIRECTION ( 'NONE',  ( 0.000000000000000000, 0.000000000000000000, 1.000000000000000000 ) ) ;
#110046=DIRECTION ( 'NONE',  ( -1.000000000000000000, 0.000000000000000000, 0.000000000000000000 ) ) ;
#110062=AXIS2_PLACEMENT_3D ( 'NONE', #152135, #170444, #12624 ) ;
#110106=CIRCLE ( 'NONE', #43483, 0.1999999999999996503 ) ;
#110114=DIRECTION ( 'NONE',  ( 0.000000000000000000, 0.9856811345164803173, 0.1686199900910455851 ) ) ;
#110124=ORIENTED_EDGE ( 'NONE', *, *, #205007, .T. ) ;
#110181=CARTESIAN_POINT ( 'NONE',  ( -18.79999999999999716, 0.000000000000000000, 0.000000000000000000 ) ) ;
#110202=EDGE_CURVE ( 'NONE', #219374, #252440, #66301, .T. ) ;
#110212=AXIS2_PLACEMENT_3D ( 'NONE', #107556, #189677, #25479 ) ;
#110213=CARTESIAN_POINT ( 'NONE',  ( -5.900000000000003020, -11.65000000000000036, 10.10000000000000142 ) ) ;
#110226=DIRECTION ( 'NONE',  ( 0.000000000000000000, 0.000000000000000000, -1.000000000000000000 ) ) ;
#110259=ORIENTED_EDGE ( 'NONE', *, *, #209568, .F. ) ;
#110262=DIRECTION ( 'NONE',  ( 1.000000000000000000, 0.000000000000000000, 0.000000000000000000 ) ) ;
#110297=AXIS2_PLACEMENT_3D ( 'NONE', #234470, #137931, #212373 ) ;
#110345=UNCERTAINTY_MEASURE_WITH_UNIT (LENGTH_MEASURE( 1.000000000000000082E-05 ), #71424, 'distance_accuracy_value', 'NONE');
#110350=DIRECTION ( 'NONE',  ( 0.000000000000000000, 0.000000000000000000, -1.000000000000000000 ) ) ;
#110371=CARTESIAN_POINT ( 'NONE',  ( 18.69999999999999929, -11.65000000000000036, 30.09999999999999787 ) ) ;
#110372=AXIS2_PLACEMENT_3D ( 'NONE', #206966, #171723, #10045 ) ;
#110379=AXIS2_PLACEMENT_3D ( 'NONE', #67260, #84195, #166399 ) ;
#110415=DIRECTION ( 'NONE',  ( 0.000000000000000000, -0.1686199900910313187, 0.9856811345164828708 ) ) ;
#110475=VECTOR ( 'NONE', #226670, 1000.000000000000000 ) ;
#110516=DIRECTION ( 'NONE',  ( -1.000000000000000000, -0.000000000000000000, -0.000000000000000000 ) ) ;
#110517=EDGE_CURVE ( 'NONE', #91491, #134169, #87308, .T. ) ;
#110561=DIRECTION ( 'NONE',  ( 0.000000000000000000, -0.1335171055202867274, -0.9910465087640866200 ) ) ;
#110565=CARTESIAN_POINT ( 'NONE',  ( -5.900000000000003020, -11.34999999999999964, 10.10000000000000142 ) ) ;
#110567=DIRECTION ( 'NONE',  ( 1.000000000000000000, -0.000000000000000000, -0.000000000000000000 ) ) ;
#110578=ORIENTED_EDGE ( 'NONE', *, *, #116209, .T. ) ;
#110593=ORIENTED_EDGE ( 'NONE', *, *, #37285, .F. ) ;
#110600=AXIS2_PLACEMENT_3D ( 'NONE', #232552, #233816, #197246 ) ;
#110601=EDGE_LOOP ( 'NONE', ( #127811, #41601, #161770, #68530 ) ) ;
#110629=CARTESIAN_POINT ( 'NONE',  ( -18.69999999999999929, 0.000000000000000000, 0.000000000000000000 ) ) ;
#110633=ORIENTED_EDGE ( 'NONE', *, *, #83187, .T. ) ;
#110677=ORIENTED_EDGE ( 'NONE', *, *, #170066, .T. ) ;
#110693=AXIS2_PLACEMENT_3D ( 'NONE', #47665, #148078, #28154 ) ;
#110717=ORIENTED_EDGE ( 'NONE', *, *, #110016, .T. ) ;
#110721=DIRECTION ( 'NONE',  ( 0.000000000000000000, 1.000000000000000000, 0.000000000000000000 ) ) ;
#110814=EDGE_LOOP ( 'NONE', ( #73888, #9509, #242748, #40538 ) ) ;
#110835=AXIS2_PLACEMENT_3D ( 'NONE', #151808, #17410, #171392 ) ;
#110926=VERTEX_POINT ( 'NONE', #191989 ) ;
#110943=VERTEX_POINT ( 'NONE', #197084 ) ;
#110967=CARTESIAN_POINT ( 'NONE',  ( 20.99105743725315776, 6.322468215188231433, 12.11686199560448252 ) ) ;
#110998=DIRECTION ( 'NONE',  ( -0.000000000000000000, 0.000000000000000000, -1.000000000000000000 ) ) ;
#111024=DIRECTION ( 'NONE',  ( -1.000000000000000000, 0.000000000000000000, 0.000000000000000000 ) ) ;
#111027=ORIENTED_EDGE ( 'NONE', *, *, #134984, .T. ) ;
#111074=ORIENTED_EDGE ( 'NONE', *, *, #198958, .F. ) ;
#111118=DIRECTION ( 'NONE',  ( 0.000000000000000000, -0.9910465087640866200, -0.1335171055202867274 ) ) ;
#111143=ORIENTED_EDGE ( 'NONE', *, *, #169202, .F. ) ;
#111160=EDGE_CURVE ( 'NONE', #243832, #172933, #244968, .T. ) ;
#111236=EDGE_CURVE ( 'NONE', #188929, #240745, #206091, .T. ) ;
#111257=EDGE_CURVE ( 'NONE', #243888, #225036, #32635, .T. ) ;
#111295=ORIENTED_EDGE ( 'NONE', *, *, #94478, .F. ) ;
#111310=ORIENTED_EDGE ( 'NONE', *, *, #91939, .F. ) ;
#111337=AXIS2_PLACEMENT_3D ( 'NONE', #108458, #111024, #190583 ) ;
#111357=LINE ( 'NONE', #34417, #43214 ) ;
#111376=FACE_OUTER_BOUND ( 'NONE', #213878, .T. ) ;
#111382=CIRCLE ( 'NONE', #119780, 0.09999999999999939493 ) ;
#111437=DIRECTION ( 'NONE',  ( 0.000000000000000000, -0.7071067811865479058, -0.7071067811865472397 ) ) ;
#111448=VECTOR ( 'NONE', #69670, 1000.000000000000000 ) ;
#111451=EDGE_CURVE ( 'NONE', #149939, #13384, #213787, .T. ) ;
#111458=DIRECTION ( 'NONE',  ( 1.000000000000000000, 0.000000000000000000, 0.000000000000000000 ) ) ;
#111480=CARTESIAN_POINT ( 'NONE',  ( -18.59999999999999787, -11.65000000000000036, 30.00000000000000000 ) ) ;
#111500=( LENGTH_UNIT ( ) NAMED_UNIT ( * ) SI_UNIT ( .MILLI., .METRE. ) );
#111579=EDGE_CURVE ( 'NONE', #168032, #217337, #58544, .T. ) ;
#111594=ORIENTED_EDGE ( 'NONE', *, *, #154179, .F. ) ;
#111605=ADVANCED_FACE ( 'NONE', ( #211888 ), #49524, .T. ) ;
#111662=DIRECTION ( 'NONE',  ( -0.000000000000000000, -1.000000000000000000, -0.000000000000000000 ) ) ;
#111685=CARTESIAN_POINT ( 'NONE',  ( -18.59999999999999787, -10.84999999999999076, 32.89999999999999858 ) ) ;
#111716=ADVANCED_FACE ( 'NONE', ( #67545 ), #246191, .T. ) ;
#111733=DIRECTION ( 'NONE',  ( -1.000000000000000000, -0.000000000000000000, -0.000000000000000000 ) ) ;
#111758=EDGE_CURVE ( 'NONE', #150585, #119824, #70588, .T. ) ;
#111811=ADVANCED_FACE ( 'NONE', ( #14968 ), #97013, .T. ) ;
#111815=CARTESIAN_POINT ( 'NONE',  ( 20.90000000000000213, 6.258114003436814343, 11.90000000000000036 ) ) ;
#111818=CARTESIAN_POINT ( 'NONE',  ( -22.94999999999999929, 0.000000000000000000, 0.000000000000000000 ) ) ;
#111868=DIRECTION ( 'NONE',  ( -0.000000000000000000, 1.000000000000000000, 1.445602896647339410E-16 ) ) ;
#111932=CIRCLE ( 'NONE', #57737, 2.599999999999998312 ) ;
#111998=ORIENTED_EDGE ( 'NONE', *, *, #216028, .T. ) ;
#112005=DIRECTION ( 'NONE',  ( 0.000000000000000000, -0.000000000000000000, -1.000000000000000000 ) ) ;
#112029=DIRECTION ( 'NONE',  ( -4.632305147810306538E-15, 0.1335171055202867274, -0.9910465087640865089 ) ) ;
#112031=DIRECTION ( 'NONE',  ( 1.000000000000000000, -0.000000000000000000, -0.000000000000000000 ) ) ;
#112082=ORIENTED_EDGE ( 'NONE', *, *, #94487, .F. ) ;
#112130=DIRECTION ( 'NONE',  ( 1.000000000000000000, 0.000000000000000000, 0.000000000000000000 ) ) ;
#112135=DIRECTION ( 'NONE',  ( 0.000000000000000000, 0.000000000000000000, 1.000000000000000000 ) ) ;
#112150=DIRECTION ( 'NONE',  ( -0.000000000000000000, -1.000000000000000000, 0.000000000000000000 ) ) ;
#112164=CARTESIAN_POINT ( 'NONE',  ( 11.60000000000000142, -8.250000000000005329, 19.04142135623731136 ) ) ;
#112215=DIRECTION ( 'NONE',  ( 0.000000000000000000, 0.000000000000000000, -1.000000000000000000 ) ) ;
#112334=EDGE_LOOP ( 'NONE', ( #174115, #253440, #147338, #205376 ) ) ;
#112341=AXIS2_PLACEMENT_3D ( 'NONE', #103305, #27684, #184133 ) ;
#112403=CARTESIAN_POINT ( 'NONE',  ( -18.69999999999999929, -8.150000000000005684, 10.50000000000000178 ) ) ;
#112430=VECTOR ( 'NONE', #83906, 1000.000000000000114 ) ;
#112471=CARTESIAN_POINT ( 'NONE',  ( -11.60000000000000320, -8.250000000000005329, 19.04142135623731491 ) ) ;
#112477=CIRCLE ( 'NONE', #220790, 0.1999999999999987899 ) ;
#112495=CYLINDRICAL_SURFACE ( 'NONE', #9527, 0.09999999999999939493 ) ;
#112518=AXIS2_PLACEMENT_3D ( 'NONE', #99874, #142858, #221125 ) ;
#112527=EDGE_CURVE ( 'NONE', #156184, #86293, #199932, .T. ) ;
#112537=AXIS2_PLACEMENT_3D ( 'NONE', #245906, #249749, #9850 ) ;
#112660=ORIENTED_EDGE ( 'NONE', *, *, #233241, .T. ) ;
#112688=EDGE_CURVE ( 'NONE', #249092, #252440, #250172, .T. ) ;
#112701=EDGE_LOOP ( 'NONE', ( #49496, #216425, #5962, #181684 ) ) ;
#112710=CARTESIAN_POINT ( 'NONE',  ( -18.79999999999999716, 1.212568896937007645, -7.900000000000000355 ) ) ;
#112716=EDGE_CURVE ( 'NONE', #56541, #248319, #246238, .T. ) ;
#112723=ORIENTED_EDGE ( 'NONE', *, *, #198684, .T. ) ;
#112724=DIRECTION ( 'NONE',  ( -1.000000000000000000, 0.000000000000000000, 0.000000000000000000 ) ) ;
#112787=AXIS2_PLACEMENT_3D ( 'NONE', #237991, #215848, #118052 ) ;
#112795=ORIENTED_EDGE ( 'NONE', *, *, #85503, .F. ) ;
#112826=VECTOR ( 'NONE', #85694, 1000.000000000000000 ) ;
#112851=DIRECTION ( 'NONE',  ( 1.000000000000000000, 0.000000000000000000, -0.000000000000000000 ) ) ;
#112902=EDGE_CURVE ( 'NONE', #49823, #255967, #173165, .T. ) ;
#112950=DIRECTION ( 'NONE',  ( 0.000000000000000000, 1.000000000000000000, 0.000000000000000000 ) ) ;
#112997=EDGE_LOOP ( 'NONE', ( #141389, #248480, #55220, #91799 ) ) ;
#113056=VERTEX_POINT ( 'NONE', #243347 ) ;
#113086=ORIENTED_EDGE ( 'NONE', *, *, #134976, .F. ) ;
#113095=DIRECTION ( 'NONE',  ( 0.000000000000000000, 0.000000000000000000, -1.000000000000000000 ) ) ;
#113114=ORIENTED_EDGE ( 'NONE', *, *, #11882, .F. ) ;
#113134=CARTESIAN_POINT ( 'NONE',  ( -20.90000000000000213, 11.59510167572422112, 1.901609089591594470 ) ) ;
#113177=DIRECTION ( 'NONE',  ( 0.000000000000000000, -0.1335171055202901691, -0.9910465087640861759 ) ) ;
#113196=DIRECTION ( 'NONE',  ( -0.000000000000000000, -0.4856429311786357728, -0.8741572761215358200 ) ) ;
#113235=ORIENTED_EDGE ( 'NONE', *, *, #46938, .T. ) ;
#113253=FACE_OUTER_BOUND ( 'NONE', #62066, .T. ) ;
#113260=ORIENTED_EDGE ( 'NONE', *, *, #48158, .T. ) ;
#113263=ADVANCED_FACE ( 'NONE', ( #157107 ), #175359, .T. ) ;
#113292=VECTOR ( 'NONE', #183903, 1000.000000000000000 ) ;
#113303=CARTESIAN_POINT ( 'NONE',  ( -18.69999999999999929, -8.250000000000005329, 10.52591260281975138 ) ) ;
#113312=CIRCLE ( 'NONE', #208987, 0.1000000000000002137 ) ;
#113327=ORIENTED_EDGE ( 'NONE', *, *, #218045, .F. ) ;
#113336=ORIENTED_EDGE ( 'NONE', *, *, #41916, .T. ) ;
#113384=ORIENTED_EDGE ( 'NONE', *, *, #221498, .F. ) ;
#113398=DIRECTION ( 'NONE',  ( 0.000000000000000000, 0.000000000000000000, 1.000000000000000000 ) ) ;
#113419=DIRECTION ( 'NONE',  ( 1.000000000000000000, 0.000000000000000000, 0.000000000000000000 ) ) ;
#113487=AXIS2_PLACEMENT_3D ( 'NONE', #187284, #105114, #242087 ) ;
#113572=AXIS2_PLACEMENT_3D ( 'NONE', #94267, #79820, #198508 ) ;
#113613=CARTESIAN_POINT ( 'NONE',  ( 11.60000000000000142, -8.350000000000004974, 19.04142135623731136 ) ) ;
#113696=ORIENTED_EDGE ( 'NONE', *, *, #145479, .F. ) ;
#113700=CARTESIAN_POINT ( 'NONE',  ( -20.90000000000000213, -1.800000000000000044, -11.61130914238355771 ) ) ;
#113721=CARTESIAN_POINT ( 'NONE',  ( 18.69999999999999929, -8.175168544775697654, 10.42878401658402510 ) ) ;
#113727=DIRECTION ( 'NONE',  ( 0.000000000000000000, 0.000000000000000000, -1.000000000000000000 ) ) ;
#113733=ORIENTED_EDGE ( 'NONE', *, *, #161606, .T. ) ;
#113766=CARTESIAN_POINT ( 'NONE',  ( 21.00000000000000000, -11.65000000000000036, 0.000000000000000000 ) ) ;
#113779=EDGE_CURVE ( 'NONE', #105678, #212150, #92485, .T. ) ;
#113781=VECTOR ( 'NONE', #11745, 1000.000000000000000 ) ;
#113785=CIRCLE ( 'NONE', #17917, 0.1000000000000000472 ) ;
#113819=ORIENTED_EDGE ( 'NONE', *, *, #129936, .T. ) ;
#113828=EDGE_CURVE ( 'NONE', #29621, #169297, #204912, .T. ) ;
#113857=ORIENTED_EDGE ( 'NONE', *, *, #108959, .T. ) ;
#113887=ADVANCED_FACE ( 'NONE', ( #235678 ), #135286, .T. ) ;
#113992=CARTESIAN_POINT ( 'NONE',  ( -22.94999999999999929, 7.900000000000000355, 1.300000000000000044 ) ) ;
#113995=CARTESIAN_POINT ( 'NONE',  ( -19.99999999999999645, 5.474129339729826960, 16.54142135623731136 ) ) ;
#114026=ORIENTED_EDGE ( 'NONE', *, *, #230832, .T. ) ;
#114028=DIRECTION ( 'NONE',  ( -1.000000000000000000, -0.000000000000000000, -0.000000000000000000 ) ) ;
#114043=EDGE_CURVE ( 'NONE', #121041, #130825, #196555, .T. ) ;
#114046=ORIENTED_EDGE ( 'NONE', *, *, #230648, .T. ) ;
#114049=VERTEX_POINT ( 'NONE', #77884 ) ;
#114116=DIRECTION ( 'NONE',  ( -0.000000000000000000, 0.1686199900910312910, -0.9856811345164826488 ) ) ;
#114145=EDGE_CURVE ( 'NONE', #91499, #128875, #50961, .T. ) ;
#114155=LINE ( 'NONE', #178008, #184502 ) ;
#114324=ADVANCED_FACE ( 'NONE', ( #254876 ), #34451, .F. ) ;
#114327=CARTESIAN_POINT ( 'NONE',  ( -21.00000000000000000, 0.3305886640091971196, 0.04453801223857078301 ) ) ;
#114345=FACE_OUTER_BOUND ( 'NONE', #36081, .T. ) ;
#114499=LINE ( 'NONE', #231900, #201111 ) ;
#114514=VECTOR ( 'NONE', #9628, 1000.000000000000000 ) ;
#114515=AXIS2_PLACEMENT_3D ( 'NONE', #208180, #11249, #177743 ) ;
#114524=EDGE_CURVE ( 'NONE', #6496, #203964, #101183, .T. ) ;
#114565=VECTOR ( 'NONE', #119716, 1000.000000000000114 ) ;
#114596=CARTESIAN_POINT ( 'NONE',  ( -0.8999999999999993561, -8.279289321881350361, 26.00000000000000355 ) ) ;
#114614=VERTEX_POINT ( 'NONE', #135718 ) ;
#114731=AXIS2_PLACEMENT_3D ( 'NONE', #34719, #115501, #17681 ) ;
#114747=EDGE_CURVE ( 'NONE', #248444, #203718, #61334, .T. ) ;
#114815=EDGE_CURVE ( 'NONE', #12728, #241189, #9654, .T. ) ;
#114824=EDGE_CURVE ( 'NONE', #176884, #33376, #246970, .T. ) ;
#114837=VECTOR ( 'NONE', #182127, 1000.000000000000000 ) ;
#114912=CARTESIAN_POINT ( 'NONE',  ( 0.8999999999999992450, -8.250000000000005329, 21.95857864376268864 ) ) ;
#114920=ORIENTED_EDGE ( 'NONE', *, *, #114747, .F. ) ;
#115029=ORIENTED_EDGE ( 'NONE', *, *, #99529, .F. ) ;
#115039=CARTESIAN_POINT ( 'NONE',  ( 20.90000000000000213, 11.59510167572422112, 1.901609089591594470 ) ) ;
#115051=DIRECTION ( 'NONE',  ( 1.000000000000000000, 0.000000000000000000, 0.000000000000000000 ) ) ;
#115072=CARTESIAN_POINT ( 'NONE',  ( -19.89999999999999503, 5.572646938319268273, 16.50000000000000000 ) ) ;
#115077=ORIENTED_EDGE ( 'NONE', *, *, #90052, .T. ) ;
#115181=AXIS2_PLACEMENT_3D ( 'NONE', #196973, #155328, #56172 ) ;
#115224=ORIENTED_EDGE ( 'NONE', *, *, #63541, .T. ) ;
#115232=ORIENTED_EDGE ( 'NONE', *, *, #198288, .F. ) ;
#115255=EDGE_LOOP ( 'NONE', ( #182957, #44771, #214037, #47355 ) ) ;
#115315=EDGE_CURVE ( 'NONE', #37087, #158566, #163967, .T. ) ;
#115335=ORIENTED_EDGE ( 'NONE', *, *, #54973, .T. ) ;
#115386=EDGE_CURVE ( 'NONE', #126102, #136069, #221998, .T. ) ;
#115406=ORIENTED_EDGE ( 'NONE', *, *, #13954, .F. ) ;
#115410=LINE ( 'NONE', #171575, #221051 ) ;
#115417=AXIS2_PLACEMENT_3D ( 'NONE', #142289, #101860, #43204 ) ;
#115436=DIRECTION ( 'NONE',  ( 0.000000000000000000, 0.000000000000000000, -1.000000000000000000 ) ) ;
#115462=AXIS2_PLACEMENT_3D ( 'NONE', #139909, #199926, #104619 ) ;
#115473=DIRECTION ( 'NONE',  ( 1.000000000000000000, -0.000000000000000000, -0.000000000000000000 ) ) ;
#115477=ORIENTED_EDGE ( 'NONE', *, *, #136852, .T. ) ;
#115489=ORIENTED_EDGE ( 'NONE', *, *, #31730, .F. ) ;
#115500=LINE ( 'NONE', #37279, #136390 ) ;
#115501=DIRECTION ( 'NONE',  ( -1.000000000000000000, 0.000000000000000000, -0.000000000000000000 ) ) ;
#115534=CIRCLE ( 'NONE', #128033, 0.09999999999999939493 ) ;
#115594=DIRECTION ( 'NONE',  ( 0.000000000000000000, -0.000000000000000000, -1.000000000000000000 ) ) ;
#115601=CARTESIAN_POINT ( 'NONE',  ( -21.10000000000000142, 5.021051876504148371E-16, -4.100000000000000533 ) ) ;
#115608=ORIENTED_EDGE ( 'NONE', *, *, #104091, .T. ) ;
#115613=CARTESIAN_POINT ( 'NONE',  ( 0.000000000000000000, 1.350000000000000089, 21.90000000000000213 ) ) ;
#115633=CARTESIAN_POINT ( 'NONE',  ( -13.40000000000000213, -11.65000000000000036, 12.30000000000000426 ) ) ;
#115651=ORIENTED_EDGE ( 'NONE', *, *, #251682, .T. ) ;
#115663=CIRCLE ( 'NONE', #207262, 0.09999999999999939493 ) ;
#115672=ORIENTED_EDGE ( 'NONE', *, *, #155762, .T. ) ;
#115674=CARTESIAN_POINT ( 'NONE',  ( -20.09999999999999787, 4.645987002755569861, 21.91686199900910736 ) ) ;
#115709=CARTESIAN_POINT ( 'NONE',  ( -18.79999999999999716, -1.311673547813416718, -7.986648289447971116 ) ) ;
#115714=ORIENTED_EDGE ( 'NONE', *, *, #188246, .T. ) ;
#115772=FACE_OUTER_BOUND ( 'NONE', #53274, .T. ) ;
#115803=CARTESIAN_POINT ( 'NONE',  ( 20.90000000000000213, 7.900000000000000355, 1.300000000000000044 ) ) ;
#115831=EDGE_LOOP ( 'NONE', ( #228731, #58219, #223369, #65817 ) ) ;
#115835=DIRECTION ( 'NONE',  ( -1.000000000000000000, 0.000000000000000000, 0.000000000000000000 ) ) ;
#115923=ORIENTED_EDGE ( 'NONE', *, *, #127082, .F. ) ;
#115957=ADVANCED_FACE ( 'NONE', ( #57174 ), #63613, .F. ) ;
#116030=DIRECTION ( 'NONE',  ( -1.462545276649518737E-15, -0.1686199900910448357, 0.9856811345164805394 ) ) ;
#116041=DIRECTION ( 'NONE',  ( 0.000000000000000000, 0.000000000000000000, -1.000000000000000000 ) ) ;
#116060=CARTESIAN_POINT ( 'NONE',  ( 22.10000000000000497, 6.322468214605804882, 12.11686199900910310 ) ) ;
#116065=LINE ( 'NONE', #173515, #101122 ) ;
#116083=CARTESIAN_POINT ( 'NONE',  ( -5.900000000000003020, -11.34999999999999964, 10.10000000000000142 ) ) ;
#116087=CARTESIAN_POINT ( 'NONE',  ( 18.79999999999999716, 5.488301202077012775, 16.40000000000000213 ) ) ;
#116102=EDGE_LOOP ( 'NONE', ( #150016, #111310, #190527, #144800 ) ) ;
#116112=DIRECTION ( 'NONE',  ( 0.000000000000000000, -0.1335171055202867274, 0.9910465087640866200 ) ) ;
#116130=CARTESIAN_POINT ( 'NONE',  ( -18.79999999999999716, 11.49641995933507843, 1.885425182446133885 ) ) ;
#116209=EDGE_CURVE ( 'NONE', #98368, #161437, #63813, .T. ) ;
#116262=DIRECTION ( 'NONE',  ( 0.000000000000000000, -1.000000000000000000, 0.000000000000000000 ) ) ;
#116291=DIRECTION ( 'NONE',  ( 0.000000000000000000, -1.000000000000000000, -1.445602896647339410E-16 ) ) ;
#116301=ADVANCED_FACE ( 'NONE', ( #167889 ), #66192, .T. ) ;
#116314=CARTESIAN_POINT ( 'NONE',  ( 18.79999999999999716, 1.350000000000000089, 16.60000000000000142 ) ) ;
#116347=EDGE_CURVE ( 'NONE', #247506, #14875, #4900, .T. ) ;
#116387=VECTOR ( 'NONE', #108595, 1000.000000000000000 ) ;
#116400=LINE ( 'NONE', #233780, #84265 ) ;
#116462=DIRECTION ( 'NONE',  ( 0.000000000000000000, 0.9910465087640865089, 0.1335171055202867274 ) ) ;
#116485=FACE_OUTER_BOUND ( 'NONE', #215630, .T. ) ;
#116522=SPHERICAL_SURFACE ( 'NONE', #151500, 0.1000000000000000056 ) ;
#116537=FACE_OUTER_BOUND ( 'NONE', #62132, .T. ) ;
#116571=CARTESIAN_POINT ( 'NONE',  ( -18.79999999999999716, 1.786320531569725478, -11.50977166988710820 ) ) ;
#116575=DIRECTION ( 'NONE',  ( -0.000000000000000000, 1.000000000000000000, -0.000000000000000000 ) ) ;
#116579=DIRECTION ( 'NONE',  ( 0.000000000000000000, -0.4856429311786292224, -0.8741572761215394838 ) ) ;
#116623=CARTESIAN_POINT ( 'NONE',  ( -22.94999999999999929, 4.611773100472912112, 22.11686199900910665 ) ) ;
#116640=EDGE_LOOP ( 'NONE', ( #32661, #91483, #24337 ) ) ;
#116710=CARTESIAN_POINT ( 'NONE',  ( 18.59999999999999787, -8.150000000000007461, 32.89999999999999858 ) ) ;
#116753=ADVANCED_FACE ( 'NONE', ( #243222 ), #204095, .F. ) ;
#116813=ORIENTED_EDGE ( 'NONE', *, *, #13394, .T. ) ;
#116853=EDGE_LOOP ( 'NONE', ( #230981, #158748, #147765, #43756 ) ) ;
#116915=DIRECTION ( 'NONE',  ( 0.000000000000000000, 0.000000000000000000, -1.000000000000000000 ) ) ;
#116936=DIRECTION ( 'NONE',  ( -0.000000000000000000, 0.000000000000000000, -1.000000000000000000 ) ) ;
#116974=ORIENTED_EDGE ( 'NONE', *, *, #257812, .F. ) ;
#117027=DIRECTION ( 'NONE',  ( -1.000000000000000000, 0.000000000000000000, -0.000000000000000000 ) ) ;
#117073=ORIENTED_EDGE ( 'NONE', *, *, #91802, .T. ) ;
#117110=DIRECTION ( 'NONE',  ( 1.000000000000000000, -0.000000000000000000, -0.000000000000000000 ) ) ;
#117128=ORIENTED_EDGE ( 'NONE', *, *, #78130, .T. ) ;
#117180=DIRECTION ( 'NONE',  ( 0.000000000000000000, 0.000000000000000000, 1.000000000000000000 ) ) ;
#117195=ADVANCED_FACE ( 'NONE', ( #185207 ), #108245, .T. ) ;
#117201=ORIENTED_EDGE ( 'NONE', *, *, #172732, .F. ) ;
#117214=FACE_OUTER_BOUND ( 'NONE', #112334, .T. ) ;
#117223=ORIENTED_EDGE ( 'NONE', *, *, #201304, .T. ) ;
#117228=ORIENTED_EDGE ( 'NONE', *, *, #254114, .F. ) ;
#117252=LINE ( 'NONE', #97654, #107115 ) ;
#117255=ORIENTED_EDGE ( 'NONE', *, *, #142002, .T. ) ;
#117280=EDGE_LOOP ( 'NONE', ( #112723, #10449, #205318, #166966 ) ) ;
#117342=CIRCLE ( 'NONE', #92377, 2.600000000000001421 ) ;
#117351=CARTESIAN_POINT ( 'NONE',  ( 20.90000000000000213, 7.900000000000000355, -1.300000000000000044 ) ) ;
#117388=EDGE_LOOP ( 'NONE', ( #215046, #131635, #186744, #35091, #56769, #62732, #69091, #181909, #133846, #173152, #77051, #42397, #239320, #8618, #23569, #130652, #31762 ) ) ;
#117392=ADVANCED_FACE ( 'NONE', ( #242291 ), #24562, .T. ) ;
#117411=EDGE_CURVE ( 'NONE', #28188, #186764, #239323, .T. ) ;
#117416=DIRECTION ( 'NONE',  ( 0.000000000000000000, -1.776356839400250465E-15, -1.000000000000000000 ) ) ;
#117442=CARTESIAN_POINT ( 'NONE',  ( 18.69999999999998153, 1.311673547813416718, -7.986648289447971116 ) ) ;
#117446=EDGE_LOOP ( 'NONE', ( #15961, #16204, #169075, #194156 ) ) ;
#117460=FACE_OUTER_BOUND ( 'NONE', #40182, .T. ) ;
#117477=SPHERICAL_SURFACE ( 'NONE', #201614, 0.1000000000000000056 ) ;
#117486=DIRECTION ( 'NONE',  ( -1.000000000000000000, 0.000000000000000000, 0.000000000000000000 ) ) ;
#117491=ORIENTED_EDGE ( 'NONE', *, *, #69359, .T. ) ;
#117509=DIRECTION ( 'NONE',  ( 1.000000000000000000, 0.000000000000000000, 0.000000000000000000 ) ) ;
#117538=AXIS2_PLACEMENT_3D ( 'NONE', #122830, #159386, #42012 ) ;
#117574=CARTESIAN_POINT ( 'NONE',  ( 21.00000000000000000, 8.000000000000000000, -1.212568896937008089 ) ) ;
#117597=CARTESIAN_POINT ( 'NONE',  ( -22.19999999999999929, -11.75000000000000178, 12.09999999999999609 ) ) ;
#117637=FACE_OUTER_BOUND ( 'NONE', #10308, .T. ) ;
#117658=DIRECTION ( 'NONE',  ( 0.000000000000000000, -1.000000000000000000, 0.000000000000000000 ) ) ;
#117674=CARTESIAN_POINT ( 'NONE',  ( -22.94999999999999929, 4.837354856632045057E-16, -3.900000000000000355 ) ) ;
#117685=AXIS2_PLACEMENT_3D ( 'NONE', #141694, #223793, #120889 ) ;
#117704=DIRECTION ( 'NONE',  ( 0.000000000000000000, -0.9856811345164803173, -0.1686199900910455851 ) ) ;
#117720=EDGE_CURVE ( 'NONE', #42394, #207660, #129262, .T. ) ;
#117726=CIRCLE ( 'NONE', #163509, 0.09999999999999990841 ) ;
#117740=AXIS2_PLACEMENT_3D ( 'NONE', #200633, #22004, #141929 ) ;
#117758=EDGE_CURVE ( 'NONE', #245573, #65906, #104294, .T. ) ;
#117795=ORIENTED_EDGE ( 'NONE', *, *, #100041, .F. ) ;
#117837=AXIS2_PLACEMENT_3D ( 'NONE', #142667, #226042, #123137 ) ;
#117842=DIRECTION ( 'NONE',  ( 0.000000000000000000, 0.000000000000000000, 1.000000000000000000 ) ) ;
#117860=EDGE_LOOP ( 'NONE', ( #245748, #201298, #36308, #149621 ) ) ;
#117869=EDGE_CURVE ( 'NONE', #184776, #70370, #118192, .T. ) ;
#117876=AXIS2_PLACEMENT_3D ( 'NONE', #99903, #116936, #176938 ) ;
#117909=ORIENTED_EDGE ( 'NONE', *, *, #161141, .T. ) ;
#117922=LINE ( 'NONE', #196190, #158755 ) ;
#117952=VECTOR ( 'NONE', #30104, 1000.000000000000000 ) ;
#117955=EDGE_CURVE ( 'NONE', #233025, #173202, #4213, .T. ) ;
#117987=DIRECTION ( 'NONE',  ( -0.000000000000000000, 0.9910465087640860649, 0.1335171055202901413 ) ) ;
#118049=ORIENTED_EDGE ( 'NONE', *, *, #144624, .F. ) ;
#118052=DIRECTION ( 'NONE',  ( 0.000000000000000000, 0.000000000000000000, -1.000000000000000000 ) ) ;
#118073=SPHERICAL_SURFACE ( 'NONE', #153049, 0.1000000000000000056 ) ;
#118085=EDGE_CURVE ( 'NONE', #141361, #135547, #124601, .T. ) ;
#118192=LINE ( 'NONE', #158630, #175101 ) ;
#118202=CARTESIAN_POINT ( 'NONE',  ( -18.79999999999999716, -10.84999999999999076, 33.00000000000000000 ) ) ;
#118275=DIRECTION ( 'NONE',  ( 0.000000000000000000, 0.000000000000000000, 1.000000000000000000 ) ) ;
#118347=CARTESIAN_POINT ( 'NONE',  ( -22.94999999999999929, 4.513204987021263825, 22.10000000000000142 ) ) ;
#118368=AXIS2_PLACEMENT_3D ( 'NONE', #105966, #40917, #100809 ) ;
#118398=CYLINDRICAL_SURFACE ( 'NONE', #147921, 0.09999999999999939493 ) ;
#118417=EDGE_CURVE ( 'NONE', #173202, #40449, #191455, .T. ) ;
#118486=EDGE_CURVE ( 'NONE', #99209, #169022, #91465, .T. ) ;
#118501=DIRECTION ( 'NONE',  ( 0.000000000000000000, 8.673617379884087537E-15, 1.000000000000000000 ) ) ;
#118553=LINE ( 'NONE', #23309, #135764 ) ;
#118574=CARTESIAN_POINT ( 'NONE',  ( -0.8999999999999993561, -8.250000000000005329, 23.40000000000000568 ) ) ;
#118606=CIRCLE ( 'NONE', #151749, 2.600000000000001421 ) ;
#118720=VERTEX_POINT ( 'NONE', #181710 ) ;
#118734=DIRECTION ( 'NONE',  ( 0.000000000000000000, 0.1686199900910313187, -0.9856811345164828708 ) ) ;
#118769=VERTEX_POINT ( 'NONE', #85133 ) ;
#118827=EDGE_LOOP ( 'NONE', ( #40279, #15044, #31285, #147967 ) ) ;
#118856=CARTESIAN_POINT ( 'NONE',  ( -19.99999999999999645, 1.350000000000000089, 16.60000000000000142 ) ) ;
#118866=CARTESIAN_POINT ( 'NONE',  ( 0.000000000000000000, -11.65000000000000036, 32.89999999999999858 ) ) ;
#118875=CARTESIAN_POINT ( 'NONE',  ( 18.69999999999999929, -8.350000000000004974, 10.95857864376268864 ) ) ;
#118883=CARTESIAN_POINT ( 'NONE',  ( 5.999999999999995559, -11.34999999999999964, 10.00000000000000178 ) ) ;
#118921=EDGE_CURVE ( 'NONE', #46280, #23059, #193274, .T. ) ;
#118957=DIRECTION ( 'NONE',  ( 0.000000000000000000, -1.000000000000000000, 0.000000000000000000 ) ) ;
#118958=CYLINDRICAL_SURFACE ( 'NONE', #165866, 0.1000000000000028644 ) ;
#119009=VECTOR ( 'NONE', #223972, 1000.000000000000114 ) ;
#119040=ADVANCED_FACE ( 'NONE', ( #120192 ), #23653, .T. ) ;
#119077=VECTOR ( 'NONE', #95499, 1000.000000000000114 ) ;
#119096=DIRECTION ( 'NONE',  ( 1.000000000000000000, 0.000000000000000000, 0.000000000000000000 ) ) ;
#119109=CARTESIAN_POINT ( 'NONE',  ( -18.79999999999999716, 11.59510167572422112, 1.901609089591594470 ) ) ;
#119119=DIRECTION ( 'NONE',  ( 1.000000000000000000, 0.000000000000000000, 0.000000000000000000 ) ) ;
#119138=ORIENTED_EDGE ( 'NONE', *, *, #195040, .T. ) ;
#119153=FACE_OUTER_BOUND ( 'NONE', #59993, .T. ) ;
#119163=CYLINDRICAL_SURFACE ( 'NONE', #128329, 0.09999999999999939493 ) ;
#119166=VECTOR ( 'NONE', #208643, 1000.000000000000000 ) ;
#119222=CIRCLE ( 'NONE', #206878, 0.1999999999999987899 ) ;
#119240=AXIS2_PLACEMENT_3D ( 'NONE', #207820, #168715, #227343 ) ;
#119252=CIRCLE ( 'NONE', #77701, 0.2000000000000005107 ) ;
#119268=DIRECTION ( 'NONE',  ( -1.000000000000000000, 0.000000000000000000, -0.000000000000000000 ) ) ;
#119286=CYLINDRICAL_SURFACE ( 'NONE', #238273, 0.1000000000000028644 ) ;
#119300=ORIENTED_EDGE ( 'NONE', *, *, #207301, .F. ) ;
#119310=DIRECTION ( 'NONE',  ( -1.000000000000000000, 0.000000000000000000, 0.000000000000000000 ) ) ;
#119362=ORIENTED_EDGE ( 'NONE', *, *, #230229, .F. ) ;
#119365=AXIS2_PLACEMENT_3D ( 'NONE', #158304, #116575, #137405 ) ;
#119391=CIRCLE ( 'NONE', #144294, 0.09999999999999939493 ) ;
#119430=ORIENTED_EDGE ( 'NONE', *, *, #32335, .T. ) ;
#119446=AXIS2_PLACEMENT_3D ( 'NONE', #90485, #48795, #170085 ) ;
#119551=CIRCLE ( 'NONE', #248710, 0.1999999999999987899 ) ;
#119583=AXIS2_PLACEMENT_3D ( 'NONE', #106587, #47908, #25791 ) ;
#119606=CARTESIAN_POINT ( 'NONE',  ( -5.900000000000002132, -11.25000000000000000, 14.00000000000000178 ) ) ;
#119612=CIRCLE ( 'NONE', #152953, 0.09999999999999939493 ) ;
#119630=EDGE_CURVE ( 'NONE', #103469, #238394, #128842, .T. ) ;
#119652=ORIENTED_EDGE ( 'NONE', *, *, #61934, .T. ) ;
#119664=DIRECTION ( 'NONE',  ( 0.000000000000000000, -0.9910465087640860649, -0.1335171055202901413 ) ) ;
#119673=DIRECTION ( 'NONE',  ( 0.000000000000000000, 0.000000000000000000, 1.000000000000000000 ) ) ;
#119681=FACE_OUTER_BOUND ( 'NONE', #73308, .T. ) ;
#119694=DIRECTION ( 'NONE',  ( -0.000000000000000000, 0.000000000000000000, 1.000000000000000000 ) ) ;
#119696=CARTESIAN_POINT ( 'NONE',  ( -13.40000000000000213, -12.25000000000000178, 15.00000000000000355 ) ) ;
#119711=AXIS2_PLACEMENT_3D ( 'NONE', #59918, #40419, #179908 ) ;
#119716=DIRECTION ( 'NONE',  ( 0.000000000000000000, 0.9910465087640860649, 0.1335171055202901413 ) ) ;
#119730=CARTESIAN_POINT ( 'NONE',  ( -22.10000000000000142, -11.65000000000000036, 33.00000000000000000 ) ) ;
#119780=AXIS2_PLACEMENT_3D ( 'NONE', #187219, #225014, #67246 ) ;
#119803=AXIS2_PLACEMENT_3D ( 'NONE', #253056, #154020, #92697 ) ;
#119804=VERTEX_POINT ( 'NONE', #217328 ) ;
#119824=VERTEX_POINT ( 'NONE', #23030 ) ;
#119835=CARTESIAN_POINT ( 'NONE',  ( -18.79999999999999716, 4.513204987021263825, 22.10000000000000142 ) ) ;
#119852=ADVANCED_FACE ( 'NONE', ( #24308 ), #150632, .T. ) ;
#119860=DIRECTION ( 'NONE',  ( 0.000000000000000000, 0.000000000000000000, 1.000000000000000000 ) ) ;
#119861=CARTESIAN_POINT ( 'NONE',  ( -20.90000000000000213, 1.885425182446134107, -11.59641995933507808 ) ) ;
#119924=DIRECTION ( 'NONE',  ( -0.000000000000000000, -0.000000000000000000, -1.000000000000000000 ) ) ;
#119949=ORIENTED_EDGE ( 'NONE', *, *, #87625, .F. ) ;
#119950=DIRECTION ( 'NONE',  ( 0.000000000000000000, -0.000000000000000000, -1.000000000000000000 ) ) ;
#119985=AXIS2_PLACEMENT_3D ( 'NONE', #174358, #236836, #60759 ) ;
#120003=VERTEX_POINT ( 'NONE', #247169 ) ;
#120006=AXIS2_PLACEMENT_3D ( 'NONE', #120008, #140826, #121300 ) ;
#120008=CARTESIAN_POINT ( 'NONE',  ( -6.000000000000003553, -11.25000000000000000, 10.00000000000000178 ) ) ;
#120043=DIRECTION ( 'NONE',  ( 1.000000000000000000, 0.000000000000000000, 0.000000000000000000 ) ) ;
#120062=ORIENTED_EDGE ( 'NONE', *, *, #5812, .F. ) ;
#120158=ORIENTED_EDGE ( 'NONE', *, *, #222922, .F. ) ;
#120174=VECTOR ( 'NONE', #11005, 1000.000000000000000 ) ;
#120189=VECTOR ( 'NONE', #197888, 1000.000000000000000 ) ;
#120192=FACE_OUTER_BOUND ( 'NONE', #133554, .T. ) ;
#120193=CARTESIAN_POINT ( 'NONE',  ( -21.10000000000000142, 6.322468214605804882, 12.11686199900910310 ) ) ;
#120337=TOROIDAL_SURFACE ( 'NONE', #7880, 11.65000000000000036, 0.1000000000000000056 ) ;
#120341=AXIS2_PLACEMENT_3D ( 'NONE', #187627, #188894, #28591 ) ;
#120364=CARTESIAN_POINT ( 'NONE',  ( -18.79999999999999716, 6.841561409100513025, 9.675512259591560138 ) ) ;
#120372=VERTEX_POINT ( 'NONE', #255488 ) ;
#120377=ADVANCED_FACE ( 'NONE', ( #196838 ), #237271, .T. ) ;
#120383=AXIS2_PLACEMENT_3D ( 'NONE', #97459, #177056, #37532 ) ;
#120442=ORIENTED_EDGE ( 'NONE', *, *, #69625, .T. ) ;
#120506=FACE_OUTER_BOUND ( 'NONE', #178549, .T. ) ;
#120562=ORIENTED_EDGE ( 'NONE', *, *, #171310, .T. ) ;
#120569=VERTEX_POINT ( 'NONE', #101566 ) ;
#120581=DIRECTION ( 'NONE',  ( 1.000000000000000000, 0.000000000000000000, 0.000000000000000000 ) ) ;
#120614=CARTESIAN_POINT ( 'NONE',  ( -21.10000000000000142, -11.64999999999999858, 11.89999999999999680 ) ) ;
#120655=DIRECTION ( 'NONE',  ( -0.000000000000000000, 1.000000000000000000, -0.000000000000000000 ) ) ;
#120657=ORIENTED_EDGE ( 'NONE', *, *, #239482, .F. ) ;
#120673=AXIS2_PLACEMENT_3D ( 'NONE', #214936, #234493, #157578 ) ;
#120725=ORIENTED_EDGE ( 'NONE', *, *, #180645, .T. ) ;
#120747=TOROIDAL_SURFACE ( 'NONE', #4188, 0.2000000000000000111, 0.1000000000000000056 ) ;
#120759=CARTESIAN_POINT ( 'NONE',  ( 21.00000000000000000, 6.841561409100513025, 9.675512259591560138 ) ) ;
#120789=DIRECTION ( 'NONE',  ( 0.000000000000000000, 0.000000000000000000, -1.000000000000000000 ) ) ;
#120867=DIRECTION ( 'NONE',  ( 1.000000000000000000, 0.000000000000000000, 0.000000000000000000 ) ) ;
#120871=EDGE_CURVE ( 'NONE', #203964, #169815, #13462, .T. ) ;
#120889=DIRECTION ( 'NONE',  ( 0.000000000000000000, 1.224646799147358384E-16, 1.000000000000000000 ) ) ;
#120947=AXIS2_PLACEMENT_3D ( 'NONE', #29407, #209279, #7218 ) ;
#120981=EDGE_CURVE ( 'NONE', #224623, #975, #17701, .T. ) ;
#121028=CYLINDRICAL_SURFACE ( 'NONE', #209334, 0.1000000000000002554 ) ;
#121031=FACE_OUTER_BOUND ( 'NONE', #75610, .T. ) ;
#121041=VERTEX_POINT ( 'NONE', #68594 ) ;
#121043=CARTESIAN_POINT ( 'NONE',  ( -0.8999999999999986899, -12.25000000000000355, 26.00000000000000355 ) ) ;
#121088=ORIENTED_EDGE ( 'NONE', *, *, #34948, .T. ) ;
#121104=EDGE_LOOP ( 'NONE', ( #164609, #33400, #203630, #223733 ) ) ;
#121119=AXIS2_PLACEMENT_3D ( 'NONE', #104124, #88407, #84532 ) ;
#121141=DIRECTION ( 'NONE',  ( -1.000000000000000000, -0.000000000000000000, 0.000000000000000000 ) ) ;
#121229=CIRCLE ( 'NONE', #25349, 0.1000000000000000472 ) ;
#121233=LINE ( 'NONE', #40409, #233727 ) ;
#121245=DIRECTION ( 'NONE',  ( 1.000000000000000000, -0.000000000000000000, -0.000000000000000000 ) ) ;
#121300=DIRECTION ( 'NONE',  ( -2.168404344971008868E-16, 0.000000000000000000, -1.000000000000000000 ) ) ;
#121306=FACE_OUTER_BOUND ( 'NONE', #188390, .T. ) ;
#121334=DIRECTION ( 'NONE',  ( 0.000000000000000000, 0.000000000000000000, -1.000000000000000000 ) ) ;
#121337=CARTESIAN_POINT ( 'NONE',  ( 18.79999999999999716, -11.65000000000000036, 32.89999999999999858 ) ) ;
#121373=CIRCLE ( 'NONE', #175516, 11.75000000000000000 ) ;
#121375=DIRECTION ( 'NONE',  ( 0.000000000000000000, 0.000000000000000000, -1.000000000000000000 ) ) ;
#121410=ORIENTED_EDGE ( 'NONE', *, *, #77344, .T. ) ;
#121424=AXIS2_PLACEMENT_3D ( 'NONE', #68749, #188682, #51715 ) ;
#121435=ADVANCED_FACE ( 'NONE', ( #124416 ), #189532, .F. ) ;
#121454=AXIS2_PLACEMENT_3D ( 'NONE', #226724, #27290, #127643 ) ;
#121479=CARTESIAN_POINT ( 'NONE',  ( 22.94999999999999929, 0.000000000000000000, -3.900000000000000355 ) ) ;
#121482=LINE ( 'NONE', #161886, #161222 ) ;
#121494=DIRECTION ( 'NONE',  ( 0.000000000000000000, 0.9910465087640866200, 0.1335171055202873380 ) ) ;
#121551=AXIS2_PLACEMENT_3D ( 'NONE', #186088, #246069, #122266 ) ;
#121596=ORIENTED_EDGE ( 'NONE', *, *, #121810, .F. ) ;
#121627=ORIENTED_EDGE ( 'NONE', *, *, #67939, .T. ) ;
#121638=DIRECTION ( 'NONE',  ( -1.000000000000000000, 0.000000000000000000, -0.000000000000000000 ) ) ;
#121643=CARTESIAN_POINT ( 'NONE',  ( -19.89999999999999858, 5.488301202077012775, 16.40000000000000213 ) ) ;
#121677=CYLINDRICAL_SURFACE ( 'NONE', #11441, 0.09999999999999990841 ) ;
#121709=DIRECTION ( 'NONE',  ( 0.000000000000000000, 0.000000000000000000, 1.000000000000000000 ) ) ;
#121735=FACE_OUTER_BOUND ( 'NONE', #33864, .T. ) ;
#121739=AXIS2_PLACEMENT_3D ( 'NONE', #18915, #56725, #38494 ) ;
#121741=VECTOR ( 'NONE', #45447, 1000.000000000000227 ) ;
#121775=CARTESIAN_POINT ( 'NONE',  ( 18.79999999999999716, -1.467286812112899463, 28.00000000000000000 ) ) ;
#121783=ORIENTED_EDGE ( 'NONE', *, *, #250512, .F. ) ;
#121795=DIRECTION ( 'NONE',  ( 0.000000000000000000, 1.000000000000000000, -0.000000000000000000 ) ) ;
#121810=EDGE_CURVE ( 'NONE', #76759, #193899, #213906, .T. ) ;
#121819=DIRECTION ( 'NONE',  ( 1.000000000000000000, 0.000000000000000000, 0.000000000000000000 ) ) ;
#121825=ORIENTED_EDGE ( 'NONE', *, *, #137120, .F. ) ;
#121833=CARTESIAN_POINT ( 'NONE',  ( 22.10000000000000142, -1.467286812112899463, 28.00000000000000000 ) ) ;
#121871=CIRCLE ( 'NONE', #142682, 0.1999999999999996503 ) ;
#121872=AXIS2_PLACEMENT_3D ( 'NONE', #123960, #84782, #203489 ) ;
#121878=CARTESIAN_POINT ( 'NONE',  ( 18.69999999999999574, -9.849999999999990763, 31.50000000000000000 ) ) ;
#121917=LINE ( 'NONE', #201432, #151785 ) ;
#121918=DIRECTION ( 'NONE',  ( 0.000000000000000000, -1.000000000000000000, 0.000000000000000000 ) ) ;
#121946=AXIS2_PLACEMENT_3D ( 'NONE', #195962, #18596, #237645 ) ;
#122006=VERTEX_POINT ( 'NONE', #89178 ) ;
#122104=FACE_OUTER_BOUND ( 'NONE', #78117, .T. ) ;
#122114=ADVANCED_FACE ( 'NONE', ( #103287 ), #100703, .F. ) ;
#122122=EDGE_CURVE ( 'NONE', #249092, #184776, #181582, .T. ) ;
#122124=DIRECTION ( 'NONE',  ( 0.000000000000000000, 0.9910465087640860649, -0.1335171055202901413 ) ) ;
#122127=LINE ( 'NONE', #196512, #192587 ) ;
#122182=DIRECTION ( 'NONE',  ( 0.000000000000000000, 0.000000000000000000, 1.000000000000000000 ) ) ;
#122229=ORIENTED_EDGE ( 'NONE', *, *, #215592, .F. ) ;
#122237=CARTESIAN_POINT ( 'NONE',  ( 20.00000000000000000, 5.474129339729826960, 16.54142135623731136 ) ) ;
#122251=VERTEX_POINT ( 'NONE', #147573 ) ;
#122262=CARTESIAN_POINT ( 'NONE',  ( -18.79999999999999716, -1.885425182446133885, -11.49641995933507843 ) ) ;
#122266=DIRECTION ( 'NONE',  ( -1.000000000000000000, 0.000000000000000000, 0.000000000000000000 ) ) ;
#122325=VECTOR ( 'NONE', #83701, 1000.000000000000000 ) ;
#122328=FACE_OUTER_BOUND ( 'NONE', #150816, .T. ) ;
#122362=CARTESIAN_POINT ( 'NONE',  ( -20.90000000000000213, -1.311673547813416718, -7.986648289447971116 ) ) ;
#122369=CARTESIAN_POINT ( 'NONE',  ( -13.40000000000000213, -8.279289321881350361, 18.97071067811866030 ) ) ;
#122384=ORIENTED_EDGE ( 'NONE', *, *, #171966, .T. ) ;
#122446=ADVANCED_FACE ( 'NONE', ( #14509 ), #237382, .T. ) ;
#122454=EDGE_CURVE ( 'NONE', #30076, #70167, #97832, .T. ) ;
#122485=ADVANCED_FACE ( 'NONE', ( #60004 ), #10074, .T. ) ;
#122496=DIRECTION ( 'NONE',  ( 0.000000000000000000, 0.000000000000000000, -1.000000000000000000 ) ) ;
#122559=DIRECTION ( 'NONE',  ( -0.000000000000000000, -0.1686199900910463068, 0.9856811345164802063 ) ) ;
#122597=ORIENTED_EDGE ( 'NONE', *, *, #186447, .T. ) ;
#122658=ADVANCED_FACE ( 'NONE', ( #29910 ), #228096, .F. ) ;
#122676=CYLINDRICAL_SURFACE ( 'NONE', #172811, 0.1000000000000000472 ) ;
#122738=VECTOR ( 'NONE', #87857, 1000.000000000000000 ) ;
#122756=CIRCLE ( 'NONE', #10323, 0.09999999999999939493 ) ;
#122782=EDGE_CURVE ( 'NONE', #31617, #168244, #137945, .T. ) ;
#122830=CARTESIAN_POINT ( 'NONE',  ( -18.60000000000000142, -8.150000000000005684, 33.00000000000000000 ) ) ;
#122843=ORIENTED_EDGE ( 'NONE', *, *, #23246, .T. ) ;
#122894=TOROIDAL_SURFACE ( 'NONE', #10287, 4.900000000000003020, 0.1000000000000000056 ) ;
#122912=AXIS2_PLACEMENT_3D ( 'NONE', #187332, #45235, #7385 ) ;
#122921=TOROIDAL_SURFACE ( 'NONE', #10495, 0.2000000000000000111, 0.1000000000000000056 ) ;
#122960=DIRECTION ( 'NONE',  ( 0.000000000000000000, 0.1686199900910463068, -0.9856811345164802063 ) ) ;
#122964=EDGE_CURVE ( 'NONE', #208058, #215605, #143130, .T. ) ;
#122979=EDGE_CURVE ( 'NONE', #241189, #257982, #155660, .T. ) ;
#123004=EDGE_CURVE ( 'NONE', #86293, #203870, #111357, .T. ) ;
#123010=CARTESIAN_POINT ( 'NONE',  ( 20.00000000000000711, 4.528782138689105174, 21.95447128030238915 ) ) ;
#123030=AXIS2_PLACEMENT_3D ( 'NONE', #204545, #25927, #100294 ) ;
#123079=CARTESIAN_POINT ( 'NONE',  ( 5.899999999999996803, -11.34999999999999964, 14.00000000000000178 ) ) ;
#123101=TOROIDAL_SURFACE ( 'NONE', #60532, 2.699999999999999734, 0.1000000000000000056 ) ;
#123136=ORIENTED_EDGE ( 'NONE', *, *, #252746, .T. ) ;
#123137=DIRECTION ( 'NONE',  ( 0.000000000000000000, 0.000000000000000000, -1.000000000000000000 ) ) ;
#123154=LINE ( 'NONE', #121878, #169479 ) ;
#123156=EDGE_LOOP ( 'NONE', ( #113235, #18635, #2042, #205754 ) ) ;
#123186=EDGE_CURVE ( 'NONE', #189932, #118769, #159480, .T. ) ;
#123195=ORIENTED_EDGE ( 'NONE', *, *, #9516, .T. ) ;
#123220=CARTESIAN_POINT ( 'NONE',  ( -0.000000000000000000, -11.25000000000000000, 13.90000000000000213 ) ) ;
#123316=ORIENTED_EDGE ( 'NONE', *, *, #176352, .T. ) ;
#123320=EDGE_CURVE ( 'NONE', #120569, #48243, #72438, .T. ) ;
#123368=AXIS2_PLACEMENT_3D ( 'NONE', #6639, #4072, #125319 ) ;
#123383=CARTESIAN_POINT ( 'NONE',  ( -18.69999999999999929, -11.65000000000000036, -15.00000000000000000 ) ) ;
#123427=ORIENTED_EDGE ( 'NONE', *, *, #152153, .F. ) ;
#123519=ADVANCED_FACE ( 'NONE', ( #219122 ), #40548, .F. ) ;
#123523=ADVANCED_FACE ( 'NONE', ( #234859 ), #238703, .T. ) ;
#123620=VECTOR ( 'NONE', #144393, 1000.000000000000000 ) ;
#123634=AXIS2_PLACEMENT_3D ( 'NONE', #118875, #177588, #139680 ) ;
#123674=ORIENTED_EDGE ( 'NONE', *, *, #24096, .T. ) ;
#123744=CARTESIAN_POINT ( 'NONE',  ( -19.89999999999999858, 5.586869315528661062, 16.41686199900910736 ) ) ;
#123813=ADVANCED_FACE ( 'NONE', ( #87315 ), #5938, .T. ) ;
#123837=DIRECTION ( 'NONE',  ( 0.000000000000000000, 0.9910465087640860649, -0.1335171055202901413 ) ) ;
#123857=TOROIDAL_SURFACE ( 'NONE', #48817, 11.65000000000000036, 0.1000000000000000056 ) ;
#123880=EDGE_LOOP ( 'NONE', ( #228461, #51547, #190300, #154938 ) ) ;
#123908=EDGE_CURVE ( 'NONE', #181190, #109505, #118606, .T. ) ;
#123960=CARTESIAN_POINT ( 'NONE',  ( 11.60000000000000142, -11.65000000000000036, 17.70000000000000284 ) ) ;
#123978=CARTESIAN_POINT ( 'NONE',  ( 18.79999999999999716, 1.250000000000000000, 16.60000000000000142 ) ) ;
#123985=ORIENTED_EDGE ( 'NONE', *, *, #166934, .T. ) ;
#124014=CARTESIAN_POINT ( 'NONE',  ( -13.40000000000000036, -8.350000000000004974, 19.04142135623731491 ) ) ;
#124045=CIRCLE ( 'NONE', #40687, 0.09999999999999939493 ) ;
#124069=ADVANCED_FACE ( 'NONE', ( #80569 ), #161442, .F. ) ;
#124092=DIRECTION ( 'NONE',  ( 1.000000000000000000, 0.000000000000000000, 0.000000000000000000 ) ) ;
#124118=ORIENTED_EDGE ( 'NONE', *, *, #2358, .F. ) ;
#124131=EDGE_CURVE ( 'NONE', #182139, #255967, #68694, .T. ) ;
#124177=EDGE_CURVE ( 'NONE', #129212, #65906, #256065, .T. ) ;
#124285=CARTESIAN_POINT ( 'NONE',  ( 20.90000000000000213, -11.75000000000000178, 0.000000000000000000 ) ) ;
#124303=CARTESIAN_POINT ( 'NONE',  ( -22.94999999999999929, 6.841561409100513025, 9.675512259591560138 ) ) ;
#124307=AXIS2_PLACEMENT_3D ( 'NONE', #245901, #72409, #30726 ) ;
#124328=DIRECTION ( 'NONE',  ( 1.000000000000000000, 0.000000000000000000, 0.000000000000000000 ) ) ;
#124350=ORIENTED_EDGE ( 'NONE', *, *, #225856, .F. ) ;
#124398=DIRECTION ( 'NONE',  ( -1.000000000000000000, 1.476360405086644309E-16, -0.000000000000000000 ) ) ;
#124416=FACE_OUTER_BOUND ( 'NONE', #167426, .T. ) ;
#124434=EDGE_CURVE ( 'NONE', #11158, #149638, #240646, .T. ) ;
#124437=SPHERICAL_SURFACE ( 'NONE', #199559, 0.1000000000000000056 ) ;
#124444=CARTESIAN_POINT ( 'NONE',  ( -20.90000000000000213, 7.900000000000000355, 1.212568896937007867 ) ) ;
#124451=CARTESIAN_POINT ( 'NONE',  ( 18.79999999999999361, -11.75000000000000000, 30.09999999999999787 ) ) ;
#124468=ORIENTED_EDGE ( 'NONE', *, *, #146894, .F. ) ;
#124514=EDGE_CURVE ( 'NONE', #190169, #184818, #69734, .T. ) ;
#124520=ADVANCED_FACE ( 'NONE', ( #184511 ), #206661, .T. ) ;
#124541=AXIS2_PLACEMENT_3D ( 'NONE', #116083, #219011, #35295 ) ;
#124552=DIRECTION ( 'NONE',  ( -0.000000000000000000, -1.000000000000000000, -0.000000000000000000 ) ) ;
#124570=EDGE_LOOP ( 'NONE', ( #102658, #194569, #163945, #209634 ) ) ;
#124601=CIRCLE ( 'NONE', #95554, 0.09999999999999990841 ) ;
#124644=ORIENTED_EDGE ( 'NONE', *, *, #245317, .F. ) ;
#124658=ORIENTED_EDGE ( 'NONE', *, *, #255489, .T. ) ;
#124670=DIRECTION ( 'NONE',  ( 0.000000000000000000, -0.000000000000000000, -1.000000000000000000 ) ) ;
#124702=AXIS2_PLACEMENT_3D ( 'NONE', #74744, #30457, #231230 ) ;
#124704=AXIS2_PLACEMENT_3D ( 'NONE', #152707, #10603, #52264 ) ;
#124734=ADVANCED_FACE ( 'NONE', ( #255688 ), #127132, .T. ) ;
#124795=LINE ( 'NONE', #23145, #133008 ) ;
#124901=DIRECTION ( 'NONE',  ( 1.000000000000000000, 0.000000000000000000, 0.000000000000000000 ) ) ;
#124974=DIRECTION ( 'NONE',  ( 0.000000000000000000, -0.1335171055202867274, 0.9910465087640866200 ) ) ;
#125018=CYLINDRICAL_SURFACE ( 'NONE', #70694, 0.09999999999999939493 ) ;
#125033=CARTESIAN_POINT ( 'NONE',  ( -18.79999999999999716, 1.350000000000000089, 16.50000000000000000 ) ) ;
#125064=FACE_OUTER_BOUND ( 'NONE', #108921, .T. ) ;
#125139=AXIS2_PLACEMENT_3D ( 'NONE', #11487, #110567, #150990 ) ;
#125217=CARTESIAN_POINT ( 'NONE',  ( 18.69999999999998153, -1.212568896937008089, -7.900000000000000355 ) ) ;
#125254=FACE_OUTER_BOUND ( 'NONE', #135843, .T. ) ;
#125266=AXIS2_PLACEMENT_3D ( 'NONE', #6100, #7390, #28286 ) ;
#125319=DIRECTION ( 'NONE',  ( 0.000000000000000000, 0.000000000000000000, -1.000000000000000000 ) ) ;
#125396=ORIENTED_EDGE ( 'NONE', *, *, #228993, .T. ) ;
#125412=EDGE_CURVE ( 'NONE', #56204, #59508, #140138, .T. ) ;
#125442=ORIENTED_EDGE ( 'NONE', *, *, #149758, .F. ) ;
#125455=CARTESIAN_POINT ( 'NONE',  ( -19.93974701750897083, 4.631764625248131928, 22.00000000173902137 ) ) ;
#125541=ADVANCED_FACE ( 'NONE', ( #150088 ), #73550, .T. ) ;
#125563=CARTESIAN_POINT ( 'NONE',  ( 21.00000000000000000, 1.212568896937007645, -7.800000000000000711 ) ) ;
#125576=ORIENTED_EDGE ( 'NONE', *, *, #99702, .T. ) ;
#125681=CARTESIAN_POINT ( 'NONE',  ( 18.79999999999999716, -8.150000000000007461, 32.89999999999999858 ) ) ;
#125688=AXIS2_PLACEMENT_3D ( 'NONE', #134289, #75644, #135576 ) ;
#125696=DIRECTION ( 'NONE',  ( 1.000000000000000000, -0.000000000000000000, -0.000000000000000000 ) ) ;
#125713=ORIENTED_EDGE ( 'NONE', *, *, #196893, .F. ) ;
#125729=EDGE_CURVE ( 'NONE', #224623, #65906, #244385, .T. ) ;
#125742=ORIENTED_EDGE ( 'NONE', *, *, #47982, .F. ) ;
#125813=ORIENTED_EDGE ( 'NONE', *, *, #218045, .T. ) ;
#125866=VERTEX_POINT ( 'NONE', #15066 ) ;
#125878=CARTESIAN_POINT ( 'NONE',  ( -18.79999999999999716, 7.800000000000000711, -1.212568896937008089 ) ) ;
#125902=ORIENTED_EDGE ( 'NONE', *, *, #38774, .F. ) ;
#125911=SURFACE_STYLE_FILL_AREA ( #183340 ) ;
#125912=EDGE_CURVE ( 'NONE', #256387, #219738, #2774, .T. ) ;
#125913=EDGE_CURVE ( 'NONE', #45320, #59375, #32034, .T. ) ;
#125994=ORIENTED_EDGE ( 'NONE', *, *, #254250, .T. ) ;
#126074=ORIENTED_EDGE ( 'NONE', *, *, #179087, .F. ) ;
#126102=VERTEX_POINT ( 'NONE', #205230 ) ;
#126131=CARTESIAN_POINT ( 'NONE',  ( -22.94999999999999929, 1.212568896937007645, -8.000000000000000000 ) ) ;
#126158=AXIS2_PLACEMENT_3D ( 'NONE', #225509, #9057, #89867 ) ;
#126180=CARTESIAN_POINT ( 'NONE',  ( 5.899999999999995914, -11.34999999999999964, 10.10000000000000142 ) ) ;
#126185=EDGE_LOOP ( 'NONE', ( #136277, #81976, #251551, #237979 ) ) ;
#126237=DIRECTION ( 'NONE',  ( 0.000000000000000000, 0.000000000000000000, 1.000000000000000000 ) ) ;
#126244=CARTESIAN_POINT ( 'NONE',  ( 20.90000000000000213, 7.986648289447971116, 1.311673547813416718 ) ) ;
#126245=ORIENTED_EDGE ( 'NONE', *, *, #218552, .F. ) ;
#126250=ORIENTED_EDGE ( 'NONE', *, *, #48446, .F. ) ;
#126385=ORIENTED_EDGE ( 'NONE', *, *, #196466, .T. ) ;
#126407=VECTOR ( 'NONE', #137147, 1000.000000000000000 ) ;
#126448=CARTESIAN_POINT ( 'NONE',  ( 18.69999999999999929, 6.644425182197215562, 9.641788261573355001 ) ) ;
#126507=FACE_OUTER_BOUND ( 'NONE', #5456, .T. ) ;
#126626=DIRECTION ( 'NONE',  ( 0.000000000000000000, 1.000000000000000000, -0.000000000000000000 ) ) ;
#126690=CARTESIAN_POINT ( 'NONE',  ( 18.69999999999999929, 7.973296578895943121, 1.410778198689824903 ) ) ;
#126708=FACE_OUTER_BOUND ( 'NONE', #168516, .T. ) ;
#126731=DIRECTION ( 'NONE',  ( -0.000000000000000000, -1.000000000000000000, -0.000000000000000000 ) ) ;
#126749=CARTESIAN_POINT ( 'NONE',  ( 22.84999999999999787, 0.000000000000000000, 0.000000000000000000 ) ) ;
#126797=ORIENTED_EDGE ( 'NONE', *, *, #245202, .F. ) ;
#126818=ORIENTED_EDGE ( 'NONE', *, *, #102875, .T. ) ;
#126821=FACE_OUTER_BOUND ( 'NONE', #247133, .T. ) ;
#126833=ADVANCED_FACE ( 'NONE', ( #27327 ), #67691, .F. ) ;
#126851=AXIS2_PLACEMENT_3D ( 'NONE', #92734, #172337, #251817 ) ;
#126859=CIRCLE ( 'NONE', #230938, 0.1000000000000001860 ) ;
#126886=CARTESIAN_POINT ( 'NONE',  ( 13.40000000000000036, -11.75000000000000000, 17.70000000000000284 ) ) ;
#126924=AXIS2_PLACEMENT_3D ( 'NONE', #5385, #182791, #42000 ) ;
#126982=ORIENTED_EDGE ( 'NONE', *, *, #62665, .T. ) ;
#126988=ORIENTED_EDGE ( 'NONE', *, *, #45630, .T. ) ;
#126998=ORIENTED_EDGE ( 'NONE', *, *, #70594, .F. ) ;
#127001=CIRCLE ( 'NONE', #2071, 0.2000000000000005107 ) ;
#127010=LINE ( 'NONE', #110007, #24122 ) ;
#127033=AXIS2_PLACEMENT_3D ( 'NONE', #97537, #139237, #178426 ) ;
#127042=CARTESIAN_POINT ( 'NONE',  ( -22.20000000000000284, 3.362550747017869046, 28.82623795144604983 ) ) ;
#127048=CARTESIAN_POINT ( 'NONE',  ( 18.79999999999999716, 0.000000000000000000, 33.00000000000000000 ) ) ;
#127080=EDGE_CURVE ( 'NONE', #178041, #5568, #180916, .T. ) ;
#127082=EDGE_CURVE ( 'NONE', #121041, #75451, #237040, .T. ) ;
#127127=EDGE_CURVE ( 'NONE', #55862, #63429, #186049, .T. ) ;
#127132=TOROIDAL_SURFACE ( 'NONE', #235447, 3.900000000000000355, 0.1000000000000000056 ) ;
#127158=EDGE_CURVE ( 'NONE', #75404, #76759, #124795, .T. ) ;
#127182=DIRECTION ( 'NONE',  ( 1.000000000000000000, -0.000000000000000000, 0.000000000000000000 ) ) ;
#127224=CARTESIAN_POINT ( 'NONE',  ( -18.69999999999999929, -10.64999999999999325, 31.39999999999999858 ) ) ;
#127275=CARTESIAN_POINT ( 'NONE',  ( 20.89999999999999858, -11.75000000000000000, -15.00000000000000000 ) ) ;
#127288=DIRECTION ( 'NONE',  ( 0.000000000000000000, -0.9910465087640860649, 0.1335171055202901413 ) ) ;
#127315=DIRECTION ( 'NONE',  ( -1.000000000000000000, -0.000000000000000000, -0.000000000000000000 ) ) ;
#127325=ORIENTED_EDGE ( 'NONE', *, *, #239482, .T. ) ;
#127328=DIRECTION ( 'NONE',  ( 1.000000000000000000, 0.000000000000000000, -0.000000000000000000 ) ) ;
#127379=ORIENTED_EDGE ( 'NONE', *, *, #76066, .F. ) ;
#127392=APPLICATION_CONTEXT ( 'automotive_design' ) ;
#127456=CARTESIAN_POINT ( 'NONE',  ( -18.79999999999999716, 11.61130914238355771, -1.800000000000000044 ) ) ;
#127565=CARTESIAN_POINT ( 'NONE',  ( -18.69999999999999929, -9.849999999999994316, 30.09999999999999787 ) ) ;
#127613=DIRECTION ( 'NONE',  ( -0.000000000000000000, -0.4856429311786292224, -0.8741572761215394838 ) ) ;
#127634=DIRECTION ( 'NONE',  ( 1.000000000000000000, -0.000000000000000000, -0.000000000000000000 ) ) ;
#127643=DIRECTION ( 'NONE',  ( 1.476360405086644309E-16, -1.000000000000000000, 0.000000000000000000 ) ) ;
#127713=DIRECTION ( 'NONE',  ( 0.000000000000000000, 3.469446951953605354E-14, -1.000000000000000000 ) ) ;
#127750=FACE_OUTER_BOUND ( 'NONE', #229453, .T. ) ;
#127756=CARTESIAN_POINT ( 'NONE',  ( 20.90000000000000213, 0.000000000000000000, 0.000000000000000000 ) ) ;
#127765=CYLINDRICAL_SURFACE ( 'NONE', #149899, 0.09999999999999990841 ) ;
#127772=AXIS2_PLACEMENT_3D ( 'NONE', #30603, #149265, #107536 ) ;
#127783=CARTESIAN_POINT ( 'NONE',  ( -18.69999999999999929, -10.80884033489985363, 6.100000000000002309 ) ) ;
#127807=ORIENTED_EDGE ( 'NONE', *, *, #226988, .F. ) ;
#127811=ORIENTED_EDGE ( 'NONE', *, *, #172973, .F. ) ;
#127815=EDGE_CURVE ( 'NONE', #109487, #166243, #161727, .T. ) ;
#127842=DIRECTION ( 'NONE',  ( -2.489438768765008884E-17, 0.1686199900910312910, -0.9856811345164826488 ) ) ;
#127850=ORIENTED_EDGE ( 'NONE', *, *, #53549, .T. ) ;
#127870=VERTEX_POINT ( 'NONE', #46867 ) ;
#127890=DIRECTION ( 'NONE',  ( 1.000000000000000000, 1.476360405086655403E-16, 0.000000000000000000 ) ) ;
#127946=CARTESIAN_POINT ( 'NONE',  ( -20.90000000000000213, 1.800000000000000044, -11.61130914238355771 ) ) ;
#127995=CARTESIAN_POINT ( 'NONE',  ( -21.10000000000000142, 0.000000000000000000, 0.000000000000000000 ) ) ;
#128031=CARTESIAN_POINT ( 'NONE',  ( 11.60000000000000142, -11.65000000000000036, 15.00000000000000355 ) ) ;
#128033=AXIS2_PLACEMENT_3D ( 'NONE', #232605, #250837, #53935 ) ;
#128051=CARTESIAN_POINT ( 'NONE',  ( 18.69999999999999929, -10.84999999999999076, 32.89999999999999858 ) ) ;
#128083=EDGE_LOOP ( 'NONE', ( #36990, #172730, #8444, #192186 ) ) ;
#128094=CIRCLE ( 'NONE', #203093, 0.09999999999999990841 ) ;
#128183=DIRECTION ( 'NONE',  ( 4.336808689942017736E-16, -0.000000000000000000, 1.000000000000000000 ) ) ;
#128231=CARTESIAN_POINT ( 'NONE',  ( 22.94999999999999929, 11.99999999999999822, 12.00000000000000000 ) ) ;
#128252=CARTESIAN_POINT ( 'NONE',  ( -37.88850191057539973, -9.749999999999943157, -15.00000000000002309 ) ) ;
#128297=VERTEX_POINT ( 'NONE', #202633 ) ;
#128304=FACE_OUTER_BOUND ( 'NONE', #180188, .T. ) ;
#128314=EDGE_LOOP ( 'NONE', ( #25472, #192792, #251343, #43191 ) ) ;
#128315=CYLINDRICAL_SURFACE ( 'NONE', #44278, 0.1000000000000028644 ) ;
#128329=AXIS2_PLACEMENT_3D ( 'NONE', #124303, #43475, #179162 ) ;
#128416=AXIS2_PLACEMENT_3D ( 'NONE', #134647, #173857, #72155 ) ;
#128441=ADVANCED_FACE ( 'NONE', ( #140073 ), #219620, .F. ) ;
#128457=DIRECTION ( 'NONE',  ( 0.000000000000000000, 0.1618390714546044939, -0.9868171638914228216 ) ) ;
#128534=EDGE_CURVE ( 'NONE', #149638, #41516, #9566, .T. ) ;
#128586=CIRCLE ( 'NONE', #124307, 0.1999999999999987899 ) ;
#128603=CARTESIAN_POINT ( 'NONE',  ( -22.19999999999999929, -11.75000000000000000, 12.09999999999999609 ) ) ;
#128648=PLANE ( 'NONE',  #76773 ) ;
#128687=ORIENTED_EDGE ( 'NONE', *, *, #79587, .T. ) ;
#128706=LINE ( 'NONE', #208247, #86547 ) ;
#128767=ORIENTED_EDGE ( 'NONE', *, *, #143200, .F. ) ;
#128777=ORIENTED_EDGE ( 'NONE', *, *, #83583, .T. ) ;
#128815=AXIS2_PLACEMENT_3D ( 'NONE', #15966, #237555, #36818 ) ;
#128818=EDGE_LOOP ( 'NONE', ( #151293, #155522, #231748, #84422, #78635, #74654, #58776, #252469, #139449, #63518, #106503, #158031, #157820 ) ) ;
#128828=DIRECTION ( 'NONE',  ( -1.000000000000000000, 0.000000000000000000, 0.000000000000000000 ) ) ;
#128842=LINE ( 'NONE', #229226, #29676 ) ;
#128860=DIRECTION ( 'NONE',  ( -1.284434275755705296E-16, 0.7071067811865471286, -0.7071067811865479058 ) ) ;
#128870=CIRCLE ( 'NONE', #145583, 0.1000000000000002554 ) ;
#128875=VERTEX_POINT ( 'NONE', #119109 ) ;
#128883=CONICAL_SURFACE ( 'NONE', #191248, 4.000000000000000000, 0.7853981633974487231 ) ;
#128893=CARTESIAN_POINT ( 'NONE',  ( 20.90000000000000213, -1.885425182446133885, -11.49641995933507843 ) ) ;
#128899=CARTESIAN_POINT ( 'NONE',  ( -18.59999999999999787, -8.175168544775697654, 10.42878401658402510 ) ) ;
#128952=DIRECTION ( 'NONE',  ( 0.000000000000000000, 0.1686199900910312910, -0.9856811345164826488 ) ) ;
#128980=DIRECTION ( 'NONE',  ( 1.000000000000000000, 0.000000000000000000, 0.000000000000000000 ) ) ;
#128986=ORIENTED_EDGE ( 'NONE', *, *, #1267, .F. ) ;
#128994=EDGE_CURVE ( 'NONE', #14935, #66123, #166006, .T. ) ;
#129042=CARTESIAN_POINT ( 'NONE',  ( -22.94999999999999929, -1.885425182446134107, -11.59641995933507808 ) ) ;
#129058=ORIENTED_EDGE ( 'NONE', *, *, #98227, .T. ) ;
#129072=VERTEX_POINT ( 'NONE', #148956 ) ;
#129089=LINE ( 'NONE', #189059, #30292 ) ;
#129143=DIRECTION ( 'NONE',  ( 3.469446951953515108E-14, 0.000000000000000000, 1.000000000000000000 ) ) ;
#129163=CYLINDRICAL_SURFACE ( 'NONE', #38290, 0.09999999999999939493 ) ;
#129187=CIRCLE ( 'NONE', #187452, 0.09999999999999939493 ) ;
#129194=ORIENTED_EDGE ( 'NONE', *, *, #122122, .F. ) ;
#129210=DIRECTION ( 'NONE',  ( -1.000000000000000000, 0.000000000000000000, 0.000000000000000000 ) ) ;
#129212=VERTEX_POINT ( 'NONE', #161465 ) ;
#129220=DIRECTION ( 'NONE',  ( 0.000000000000000000, 0.000000000000000000, 1.000000000000000000 ) ) ;
#129246=ORIENTED_EDGE ( 'NONE', *, *, #6348, .T. ) ;
#129262=CIRCLE ( 'NONE', #199994, 0.1000000000000001860 ) ;
#129440=ORIENTED_EDGE ( 'NONE', *, *, #131754, .T. ) ;
#129443=CARTESIAN_POINT ( 'NONE',  ( 18.79999999999999716, 7.973296578895943121, -1.410778198689825347 ) ) ;
#129447=FACE_OUTER_BOUND ( 'NONE', #53059, .T. ) ;
#129471=DIRECTION ( 'NONE',  ( -0.000000000000000000, 1.000000000000000000, -0.000000000000000000 ) ) ;
#129493=DIRECTION ( 'NONE',  ( 0.000000000000000000, 0.9856811345164800953, 0.1686199900910462790 ) ) ;
#129505=CYLINDRICAL_SURFACE ( 'NONE', #29259, 0.09999999999999939493 ) ;
#129547=DIRECTION ( 'NONE',  ( 0.000000000000000000, 0.9868171638914230437, -0.1618390714546045217 ) ) ;
#129580=ORIENTED_EDGE ( 'NONE', *, *, #242015, .F. ) ;
#129592=ORIENTED_EDGE ( 'NONE', *, *, #95749, .F. ) ;
#129607=VERTEX_POINT ( 'NONE', #42465 ) ;
#129656=LINE ( 'NONE', #147940, #201169 ) ;
#129661=ORIENTED_EDGE ( 'NONE', *, *, #20918, .T. ) ;
#129673=DIRECTION ( 'NONE',  ( 1.000000000000000000, 0.000000000000000000, 0.000000000000000000 ) ) ;
#129687=DIRECTION ( 'NONE',  ( 0.000000000000000000, 0.1335171055202901413, 0.9910465087640860649 ) ) ;
#129715=DIRECTION ( 'NONE',  ( 0.000000000000000000, 1.000000000000000000, 0.000000000000000000 ) ) ;
#129748=FACE_BOUND ( 'NONE', #212383, .T. ) ;
#129817=DIRECTION ( 'NONE',  ( 2.168404344971008868E-16, -0.000000000000000000, 1.000000000000000000 ) ) ;
#129862=TOROIDAL_SURFACE ( 'NONE', #200620, 4.900000000000003020, 0.1000000000000000056 ) ;
#129886=PLANE ( 'NONE',  #162985 ) ;
#129904=CARTESIAN_POINT ( 'NONE',  ( 20.00000000000000355, 11.61130914238355771, 16.50000000000000000 ) ) ;
#129925=CARTESIAN_POINT ( 'NONE',  ( 20.90000000000000213, 11.50977166988710820, 1.786320531569725478 ) ) ;
#129936=EDGE_CURVE ( 'NONE', #140091, #75404, #145093, .T. ) ;
#129944=ORIENTED_EDGE ( 'NONE', *, *, #175225, .T. ) ;
#129957=PLANE ( 'NONE',  #180310 ) ;
#129970=ADVANCED_FACE ( 'NONE', ( #155731 ), #86825, .T. ) ;
#130103=ORIENTED_EDGE ( 'NONE', *, *, #64667, .F. ) ;
#130126=FACE_OUTER_BOUND ( 'NONE', #73692, .T. ) ;
#130128=EDGE_CURVE ( 'NONE', #156872, #78593, #74418, .T. ) ;
#130137=CARTESIAN_POINT ( 'NONE',  ( -20.09999999999999787, 5.454087299794355026, 16.60000000000000142 ) ) ;
#130141=ORIENTED_EDGE ( 'NONE', *, *, #187515, .T. ) ;
#130147=EDGE_CURVE ( 'NONE', #171566, #208058, #103575, .T. ) ;
#130154=CARTESIAN_POINT ( 'NONE',  ( -21.04552871983376505, 6.223900101736508539, 12.00000000000000178 ) ) ;
#130273=AXIS2_PLACEMENT_3D ( 'NONE', #242251, #64898, #3638 ) ;
#130323=LINE ( 'NONE', #69098, #168083 ) ;
#130363=TOROIDAL_SURFACE ( 'NONE', #234409, 0.2000000000000000111, 0.1000000000000000056 ) ;
#130372=CARTESIAN_POINT ( 'NONE',  ( -22.94999999999999929, 11.50977166988710820, 1.786320531569725478 ) ) ;
#130396=ORIENTED_EDGE ( 'NONE', *, *, #127158, .F. ) ;
#130397=VERTEX_POINT ( 'NONE', #118856 ) ;
#130473=CARTESIAN_POINT ( 'NONE',  ( -18.79999999999999716, 7.973296578895943121, 1.410778198689825347 ) ) ;
#130502=EDGE_LOOP ( 'NONE', ( #129592, #161994, #216404, #101403 ) ) ;
#130531=CARTESIAN_POINT ( 'NONE',  ( -18.79999999999999716, -11.65000000000000036, 32.89999999999999858 ) ) ;
#130536=CARTESIAN_POINT ( 'NONE',  ( -18.79999999999999716, 1.901609089591594470, -11.59510167572422112 ) ) ;
#130546=AXIS2_PLACEMENT_3D ( 'NONE', #89342, #35824, #210590 ) ;
#130626=CARTESIAN_POINT ( 'NONE',  ( -19.89999999999999858, 4.611773100472912112, 22.11686199900910665 ) ) ;
#130633=DIRECTION ( 'NONE',  ( -1.000000000000000000, 0.000000000000000000, 0.000000000000000000 ) ) ;
#130641=CIRCLE ( 'NONE', #243069, 0.09999999999999939493 ) ;
#130652=ORIENTED_EDGE ( 'NONE', *, *, #124131, .F. ) ;
#130656=DIRECTION ( 'NONE',  ( 0.000000000000000000, -1.000000000000000000, 0.000000000000000000 ) ) ;
#130698=AXIS2_PLACEMENT_3D ( 'NONE', #152107, #172971, #132524 ) ;
#130706=DIRECTION ( 'NONE',  ( -0.000000000000000000, 0.1335171055202901413, 0.9910465087640860649 ) ) ;
#130711=AXIS2_PLACEMENT_3D ( 'NONE', #236869, #179492, #139016 ) ;
#130715=AXIS2_PLACEMENT_3D ( 'NONE', #62576, #123837, #198222 ) ;
#130808=VECTOR ( 'NONE', #125696, 1000.000000000000000 ) ;
#130816=ORIENTED_EDGE ( 'NONE', *, *, #118085, .T. ) ;
#130825=VERTEX_POINT ( 'NONE', #139356 ) ;
#130918=ORIENTED_EDGE ( 'NONE', *, *, #195070, .T. ) ;
#131008=EDGE_CURVE ( 'NONE', #48243, #93865, #213139, .T. ) ;
#131021=ORIENTED_EDGE ( 'NONE', *, *, #114815, .T. ) ;
#131058=EDGE_CURVE ( 'NONE', #41292, #5669, #183262, .T. ) ;
#131060=CIRCLE ( 'NONE', #51351, 0.09999999999999939493 ) ;
#131121=DIRECTION ( 'NONE',  ( 0.000000000000000000, 0.000000000000000000, -1.000000000000000000 ) ) ;
#131136=DIRECTION ( 'NONE',  ( 0.000000000000000000, 0.000000000000000000, -1.000000000000000000 ) ) ;
#131184=DIRECTION ( 'NONE',  ( 0.000000000000000000, 0.000000000000000000, 1.000000000000000000 ) ) ;
#131185=CARTESIAN_POINT ( 'NONE',  ( -18.59999999999999787, -14.35849056603774976, -0.4952830188679671064 ) ) ;
#131272=VECTOR ( 'NONE', #13593, 1000.000000000000000 ) ;
#131274=LINE ( 'NONE', #53013, #80290 ) ;
#131296=EDGE_LOOP ( 'NONE', ( #179723, #22914, #62623, #154343 ) ) ;
#131302=LINE ( 'NONE', #231709, #37981 ) ;
#131316=ORIENTED_EDGE ( 'NONE', *, *, #6288, .T. ) ;
#131356=ORIENTED_EDGE ( 'NONE', *, *, #197187, .T. ) ;
#131374=VERTEX_POINT ( 'NONE', #132019 ) ;
#131394=AXIS2_PLACEMENT_3D ( 'NONE', #236790, #2023, #38610 ) ;
#131454=CIRCLE ( 'NONE', #247972, 0.1000000000000000472 ) ;
#131467=AXIS2_PLACEMENT_3D ( 'NONE', #48402, #147514, #49696 ) ;
#131473=DIRECTION ( 'NONE',  ( 0.000000000000000000, -1.000000000000000000, 0.000000000000000000 ) ) ;
#131494=CARTESIAN_POINT ( 'NONE',  ( -18.79999999999999716, -11.75000000000000000, 30.09999999999999787 ) ) ;
#131505=CIRCLE ( 'NONE', #19074, 3.900000000000000355 ) ;
#131528=FACE_OUTER_BOUND ( 'NONE', #177384, .T. ) ;
#131563=DIRECTION ( 'NONE',  ( 1.000000000000000000, -0.000000000000000000, -0.000000000000000000 ) ) ;
#131568=ORIENTED_EDGE ( 'NONE', *, *, #191230, .T. ) ;
#131575=CARTESIAN_POINT ( 'NONE',  ( -19.99999999999999645, 11.61130914238355771, 16.50000000000000000 ) ) ;
#131587=LINE ( 'NONE', #209854, #172809 ) ;
#131589=VERTEX_POINT ( 'NONE', #82289 ) ;
#131604=CARTESIAN_POINT ( 'NONE',  ( -11.60000000000000320, -8.250000000000007105, 15.00000000000000355 ) ) ;
#131614=EDGE_CURVE ( 'NONE', #77088, #208877, #21094, .T. ) ;
#131635=ORIENTED_EDGE ( 'NONE', *, *, #64339, .T. ) ;
#131696=SPHERICAL_SURFACE ( 'NONE', #161906, 0.1000000000000000056 ) ;
#131700=CARTESIAN_POINT ( 'NONE',  ( 13.40000000000000036, -11.65000000000000036, 15.00000000000000355 ) ) ;
#131702=CARTESIAN_POINT ( 'NONE',  ( -20.90000000000000213, 6.356682116888462630, 11.91686199900910381 ) ) ;
#131754=EDGE_CURVE ( 'NONE', #102722, #156184, #206125, .T. ) ;
#131771=ADVANCED_FACE ( 'NONE', ( #47024 ), #134266, .F. ) ;
#131783=AXIS2_PLACEMENT_3D ( 'NONE', #200095, #20180, #237926 ) ;
#131818=DIRECTION ( 'NONE',  ( -0.000000000000000000, 0.000000000000000000, 1.000000000000000000 ) ) ;
#131908=AXIS2_PLACEMENT_3D ( 'NONE', #195055, #239301, #157221 ) ;
#131914=CARTESIAN_POINT ( 'NONE',  ( -13.40000000000000213, -8.250000000000007105, 12.40000000000000391 ) ) ;
#131982=DIRECTION ( 'NONE',  ( -1.000000000000000000, 0.000000000000000000, 0.000000000000000000 ) ) ;
#132019=CARTESIAN_POINT ( 'NONE',  ( -20.90000000000000213, 1.212568896937007645, -7.900000000000000355 ) ) ;
#132027=CARTESIAN_POINT ( 'NONE',  ( -22.10000000000000142, -11.65000000000000036, -15.00000000000000000 ) ) ;
#132038=CARTESIAN_POINT ( 'NONE',  ( 0.8999999999999993561, -8.279289321881350361, 29.97071067811866030 ) ) ;
#132048=ORIENTED_EDGE ( 'NONE', *, *, #124434, .T. ) ;
#132073=ADVANCED_FACE ( 'NONE', ( #108003 ), #233531, .T. ) ;
#132097=VERTEX_POINT ( 'NONE', #127565 ) ;
#132131=EDGE_CURVE ( 'NONE', #248722, #137467, #246232, .T. ) ;
#132144=CARTESIAN_POINT ( 'NONE',  ( -20.90000000000000213, 0.000000000000000000, 0.000000000000000000 ) ) ;
#132175=EDGE_CURVE ( 'NONE', #248318, #57247, #229602, .T. ) ;
#132212=CIRCLE ( 'NONE', #78229, 0.2000000000000005107 ) ;
#132244=CARTESIAN_POINT ( 'NONE',  ( -18.60000000000000142, -8.150000000000005684, 32.89999999999999858 ) ) ;
#132288=ORIENTED_EDGE ( 'NONE', *, *, #24096, .F. ) ;
#132306=VERTEX_POINT ( 'NONE', #185793 ) ;
#132411=ORIENTED_EDGE ( 'NONE', *, *, #69293, .F. ) ;
#132413=ADVANCED_FACE ( 'NONE', ( #33111 ), #153057, .F. ) ;
#132464=EDGE_LOOP ( 'NONE', ( #165224, #150950, #193025, #89794 ) ) ;
#132472=DIRECTION ( 'NONE',  ( 1.000000000000000000, -0.000000000000000000, -0.000000000000000000 ) ) ;
#132501=EDGE_CURVE ( 'NONE', #254397, #138780, #233873, .T. ) ;
#132503=AXIS2_PLACEMENT_3D ( 'NONE', #61693, #122960, #202489 ) ;
#132510=DIRECTION ( 'NONE',  ( 1.000000000000000000, -0.000000000000000000, -0.000000000000000000 ) ) ;
#132524=DIRECTION ( 'NONE',  ( -1.000000000000000000, 0.000000000000000000, 0.000000000000000000 ) ) ;
#132555=FACE_OUTER_BOUND ( 'NONE', #62236, .T. ) ;
#132669=CARTESIAN_POINT ( 'NONE',  ( -18.69999999999999929, 1.885425182446137438, -11.49641995933507843 ) ) ;
#132688=CARTESIAN_POINT ( 'NONE',  ( -19.99999999999999645, 5.645774302107834153, 15.47947886955507890 ) ) ;
#132705=CARTESIAN_POINT ( 'NONE',  ( -18.79999999999999716, 1.212568896937007645, -8.000000000000000000 ) ) ;
#132749=VECTOR ( 'NONE', #121141, 1000.000000000000000 ) ;
#132765=PRODUCT_DEFINITION_SHAPE ( 'NONE', 'NONE',  #5427 ) ;
#132769=AXIS2_PLACEMENT_3D ( 'NONE', #2588, #202093, #82108 ) ;
#132797=CARTESIAN_POINT ( 'NONE',  ( 18.69999999999999929, -9.849999999999996092, 31.39999999999999858 ) ) ;
#132801=AXIS2_PLACEMENT_3D ( 'NONE', #230216, #51542, #213203 ) ;
#132834=DIRECTION ( 'NONE',  ( -0.000000000000000000, 1.000000000000000000, -0.000000000000000000 ) ) ;
#132842=DIRECTION ( 'NONE',  ( 0.000000000000000000, 0.000000000000000000, 1.000000000000000000 ) ) ;
#132856=CARTESIAN_POINT ( 'NONE',  ( 18.79999999999999716, 6.742993295648862961, 9.658650260582458458 ) ) ;
#132913=CARTESIAN_POINT ( 'NONE',  ( 18.79999999999999716, 0.000000000000000000, 0.000000000000000000 ) ) ;
#132961=VERTEX_POINT ( 'NONE', #56148 ) ;
#132983=CARTESIAN_POINT ( 'NONE',  ( 18.79999999999999716, 1.350000000000000089, 16.40000000000000213 ) ) ;
#133008=VECTOR ( 'NONE', #187344, 1000.000000000000000 ) ;
#133020=CARTESIAN_POINT ( 'NONE',  ( 19.90000000000000924, 4.611773100472912112, 22.11686199900910665 ) ) ;
#133023=FACE_OUTER_BOUND ( 'NONE', #210870, .T. ) ;
#133032=ORIENTED_EDGE ( 'NONE', *, *, #38254, .T. ) ;
#133037=DIRECTION ( 'NONE',  ( -1.000000000000000000, 0.000000000000000000, 0.000000000000000000 ) ) ;
#133055=DIRECTION ( 'NONE',  ( 0.000000000000000000, -1.000000000000000000, 0.000000000000000000 ) ) ;
#133082=ORIENTED_EDGE ( 'NONE', *, *, #104855, .F. ) ;
#133083=CARTESIAN_POINT ( 'NONE',  ( 5.999999999999997335, -11.65000000000000036, 13.90000000000000213 ) ) ;
#133108=DIRECTION ( 'NONE',  ( 0.000000000000000000, 0.000000000000000000, -1.000000000000000000 ) ) ;
#133120=ORIENTED_EDGE ( 'NONE', *, *, #62322, .F. ) ;
#133144=EDGE_CURVE ( 'NONE', #98368, #149939, #192550, .T. ) ;
#133215=EDGE_CURVE ( 'NONE', #243888, #9700, #84150, .T. ) ;
#133223=ORIENTED_EDGE ( 'NONE', *, *, #201061, .F. ) ;
#133239=LINE ( 'NONE', #112403, #211674 ) ;
#133248=CARTESIAN_POINT ( 'NONE',  ( -13.40000000000000036, -9.650000000000005684, 17.60000000000000497 ) ) ;
#133249=EDGE_LOOP ( 'NONE', ( #12991, #105372, #172507, #163012 ) ) ;
#133277=DIRECTION ( 'NONE',  ( 0.000000000000000000, 0.000000000000000000, 1.000000000000000000 ) ) ;
#133287=CIRCLE ( 'NONE', #99378, 5.000000000000000888 ) ;
#133323=CARTESIAN_POINT ( 'NONE',  ( 18.59999999999999787, -11.75000000000000000, 6.100000000000001421 ) ) ;
#133328=EDGE_CURVE ( 'NONE', #81824, #122006, #18002, .T. ) ;
#133334=CARTESIAN_POINT ( 'NONE',  ( 19.90000000000000568, 1.350000000000000089, 0.000000000000000000 ) ) ;
#133360=EDGE_CURVE ( 'NONE', #69468, #74968, #216195, .T. ) ;
#133455=DIRECTION ( 'NONE',  ( -1.000000000000000000, 0.000000000000000000, 0.000000000000000000 ) ) ;
#133476=DIRECTION ( 'NONE',  ( 0.000000000000000000, 0.9910465087640861759, -0.1335171055202901691 ) ) ;
#133507=EDGE_LOOP ( 'NONE', ( #95395, #204224, #55686, #88058 ) ) ;
#133552=AXIS2_PLACEMENT_3D ( 'NONE', #254216, #33955, #76870 ) ;
#133554=EDGE_LOOP ( 'NONE', ( #152457, #187427, #30459, #62539 ) ) ;
#133590=EDGE_CURVE ( 'NONE', #255181, #99209, #196823, .T. ) ;
#133591=CARTESIAN_POINT ( 'NONE',  ( -13.40000000000000213, -8.350000000000003197, 10.95857864376269042 ) ) ;
#133596=EDGE_LOOP ( 'NONE', ( #4282, #129580, #239954, #207939 ) ) ;
#133599=CARTESIAN_POINT ( 'NONE',  ( 18.79999999999999716, 11.49641995933507843, 1.885425182446133885 ) ) ;
#133600=DIRECTION ( 'NONE',  ( 0.000000000000000000, -0.5773469543544729188, -0.8164989248600478255 ) ) ;
#133631=EDGE_CURVE ( 'NONE', #15770, #129072, #38608, .T. ) ;
#133655=EDGE_CURVE ( 'NONE', #101761, #83713, #30429, .T. ) ;
#133667=ADVANCED_FACE ( 'NONE', ( #75141 ), #130363, .F. ) ;
#133677=CIRCLE ( 'NONE', #42122, 0.09999999999999939493 ) ;
#133710=DIRECTION ( 'NONE',  ( 1.000000000000000000, 0.000000000000000000, 0.000000000000000000 ) ) ;
#133715=CYLINDRICAL_SURFACE ( 'NONE', #38224, 0.09999999999999939493 ) ;
#133734=ORIENTED_EDGE ( 'NONE', *, *, #200081, .T. ) ;
#133803=FACE_OUTER_BOUND ( 'NONE', #159738, .T. ) ;
#133810=VECTOR ( 'NONE', #205199, 1000.000000000000000 ) ;
#133830=CYLINDRICAL_SURFACE ( 'NONE', #185833, 0.09999999999999933942 ) ;
#133846=ORIENTED_EDGE ( 'NONE', *, *, #246388, .T. ) ;
#133899=DIRECTION ( 'NONE',  ( -0.000000000000000000, 0.1686199900910312910, -0.9856811345164826488 ) ) ;
#133937=LINE ( 'NONE', #176958, #50446 ) ;
#133954=EDGE_CURVE ( 'NONE', #176884, #159030, #105396, .T. ) ;
#134008=LINE ( 'NONE', #34953, #76067 ) ;
#134065=DIRECTION ( 'NONE',  ( 1.000000000000000000, 0.000000000000000000, 0.000000000000000000 ) ) ;
#134112=FACE_OUTER_BOUND ( 'NONE', #218410, .T. ) ;
#134118=DIRECTION ( 'NONE',  ( 0.000000000000000000, 0.000000000000000000, 1.000000000000000000 ) ) ;
#134145=EDGE_CURVE ( 'NONE', #219183, #121041, #72312, .T. ) ;
#134151=EDGE_LOOP ( 'NONE', ( #245482, #252550, #38490, #239778 ) ) ;
#134154=DIRECTION ( 'NONE',  ( -1.000000000000000000, 0.000000000000000000, 0.000000000000000000 ) ) ;
#134162=EDGE_CURVE ( 'NONE', #88008, #77088, #43082, .T. ) ;
#134169=VERTEX_POINT ( 'NONE', #126448 ) ;
#134185=CARTESIAN_POINT ( 'NONE',  ( 0.8999999999999992450, -8.350000000000004974, 21.95857864376269220 ) ) ;
#134188=DIRECTION ( 'NONE',  ( 0.000000000000000000, 0.000000000000000000, -1.000000000000000000 ) ) ;
#134252=ORIENTED_EDGE ( 'NONE', *, *, #54897, .T. ) ;
#134266=CYLINDRICAL_SURFACE ( 'NONE', #133552, 0.1000000000000002554 ) ;
#134289=CARTESIAN_POINT ( 'NONE',  ( 18.69999999999999929, -8.350000000000004974, 10.95857864376269575 ) ) ;
#134298=EDGE_LOOP ( 'NONE', ( #216924, #41125, #210688, #9474 ) ) ;
#134379=DIRECTION ( 'NONE',  ( 0.000000000000000000, -1.445602896647342861E-16, 1.000000000000000000 ) ) ;
#134397=ORIENTED_EDGE ( 'NONE', *, *, #70003, .T. ) ;
#134416=DIRECTION ( 'NONE',  ( -1.000000000000000000, 0.000000000000000000, -0.000000000000000000 ) ) ;
#134437=EDGE_LOOP ( 'NONE', ( #143478, #94284, #111594, #113327 ) ) ;
#134455=ORIENTED_EDGE ( 'NONE', *, *, #141554, .T. ) ;
#134556=DIRECTION ( 'NONE',  ( 0.000000000000000000, -0.1686199900910857752, 0.9856811345164735449 ) ) ;
#134586=FACE_OUTER_BOUND ( 'NONE', #230931, .T. ) ;
#134603=EDGE_CURVE ( 'NONE', #221804, #120003, #55868, .T. ) ;
#134605=LINE ( 'NONE', #235024, #119077 ) ;
#134647=CARTESIAN_POINT ( 'NONE',  ( 18.59999999999999787, -9.849999999999994316, 30.09999999999999787 ) ) ;
#134652=ORIENTED_EDGE ( 'NONE', *, *, #124131, .T. ) ;
#134654=EDGE_CURVE ( 'NONE', #113056, #236459, #163495, .T. ) ;
#134709=VECTOR ( 'NONE', #890, 1000.000000000000000 ) ;
#134731=CARTESIAN_POINT ( 'NONE',  ( -20.90000000000000213, -1.300000000000000044, -7.800000000000000711 ) ) ;
#134748=EDGE_LOOP ( 'NONE', ( #72008, #7276, #22561, #76024 ) ) ;
#134799=VECTOR ( 'NONE', #6499, 1000.000000000000000 ) ;
#134800=ORIENTED_EDGE ( 'NONE', *, *, #191258, .F. ) ;
#134811=CIRCLE ( 'NONE', #76573, 5.000000000000004441 ) ;
#134821=FACE_OUTER_BOUND ( 'NONE', #40698, .T. ) ;
#134824=CARTESIAN_POINT ( 'NONE',  ( -19.95857864376268864, 5.488301202077012775, 16.50000000000000000 ) ) ;
#134845=AXIS2_PLACEMENT_3D ( 'NONE', #150924, #152235, #229185 ) ;
#134871=AXIS2_PLACEMENT_3D ( 'NONE', #210486, #206622, #107514 ) ;
#134914=VECTOR ( 'NONE', #181259, 1000.000000000000000 ) ;
#134915=DIRECTION ( 'NONE',  ( 0.000000000000000000, -1.000000000000000000, 0.000000000000000000 ) ) ;
#134954=DIRECTION ( 'NONE',  ( 0.000000000000000000, 1.000000000000000000, -0.000000000000000000 ) ) ;
#134976=EDGE_CURVE ( 'NONE', #97541, #23890, #73901, .T. ) ;
#134984=EDGE_CURVE ( 'NONE', #159030, #36331, #238063, .T. ) ;
#135103=ORIENTED_EDGE ( 'NONE', *, *, #225875, .T. ) ;
#135117=EDGE_CURVE ( 'NONE', #105944, #129607, #8461, .T. ) ;
#135160=DIRECTION ( 'NONE',  ( 0.000000000000000000, 0.000000000000000000, 1.000000000000000000 ) ) ;
#135179=TOROIDAL_SURFACE ( 'NONE', #110062, 4.041421356237307805, 0.1000000000000000056 ) ;
#135278=CARTESIAN_POINT ( 'NONE',  ( -20.90000000000000213, 6.356682116888462630, 11.91686199900910381 ) ) ;
#135285=CARTESIAN_POINT ( 'NONE',  ( 18.69999999999999929, 7.800000000000000711, -15.00000000000000000 ) ) ;
#135286=CYLINDRICAL_SURFACE ( 'NONE', #34269, 0.1000000000000001443 ) ;
#135292=EDGE_CURVE ( 'NONE', #67059, #150585, #176354, .T. ) ;
#135297=ADVANCED_FACE ( 'NONE', ( #199950 ), #62984, .T. ) ;
#135304=FACE_OUTER_BOUND ( 'NONE', #42016, .T. ) ;
#135323=LINE ( 'NONE', #234426, #187622 ) ;
#135397=EDGE_LOOP ( 'NONE', ( #257950, #229776, #217820, #109826 ) ) ;
#135411=LINE ( 'NONE', #177152, #47701 ) ;
#135421=CARTESIAN_POINT ( 'NONE',  ( -20.90000000000000213, 11.49641995933507843, 1.885425182446133885 ) ) ;
#135424=CARTESIAN_POINT ( 'NONE',  ( -21.00000000000000000, 0.000000000000000000, -7.800000000000000711 ) ) ;
#135477=ORIENTED_EDGE ( 'NONE', *, *, #95903, .F. ) ;
#135500=ORIENTED_EDGE ( 'NONE', *, *, #94194, .T. ) ;
#135505=CARTESIAN_POINT ( 'NONE',  ( -21.10000000000000142, 0.000000000000000000, 0.000000000000000000 ) ) ;
#135523=EDGE_CURVE ( 'NONE', #228920, #77088, #222264, .T. ) ;
#135547=VERTEX_POINT ( 'NONE', #12024 ) ;
#135557=CIRCLE ( 'NONE', #114731, 0.09999999999999939493 ) ;
#135566=CARTESIAN_POINT ( 'NONE',  ( 0.8999999999999993561, -11.75000000000000000, 28.70000000000000284 ) ) ;
#135576=DIRECTION ( 'NONE',  ( 0.000000000000000000, 0.000000000000000000, 1.000000000000000000 ) ) ;
#135577=CIRCLE ( 'NONE', #160570, 4.041421356237310469 ) ;
#135618=SPHERICAL_SURFACE ( 'NONE', #124541, 0.1000000000000000056 ) ;
#135630=CIRCLE ( 'NONE', #23239, 11.65000000000000036 ) ;
#135680=ORIENTED_EDGE ( 'NONE', *, *, #202062, .T. ) ;
#135689=EDGE_LOOP ( 'NONE', ( #193529, #133734, #183939, #240259 ) ) ;
#135718=CARTESIAN_POINT ( 'NONE',  ( -18.69999999999999929, 1.350000000000000089, 22.10000000000000142 ) ) ;
#135729=EDGE_CURVE ( 'NONE', #1224, #176884, #84434, .T. ) ;
#135732=CARTESIAN_POINT ( 'NONE',  ( 0.8999999999999993561, -11.65000000000000036, 28.70000000000000284 ) ) ;
#135736=AXIS2_PLACEMENT_3D ( 'NONE', #55090, #216758, #62826 ) ;
#135764=VECTOR ( 'NONE', #198059, 1000.000000000000000 ) ;
#135824=FACE_OUTER_BOUND ( 'NONE', #184217, .T. ) ;
#135834=CYLINDRICAL_SURFACE ( 'NONE', #123634, 0.09999999999999939493 ) ;
#135842=ORIENTED_EDGE ( 'NONE', *, *, #104091, .F. ) ;
#135843=EDGE_LOOP ( 'NONE', ( #126797, #82734, #104957 ) ) ;
#135852=CARTESIAN_POINT ( 'NONE',  ( 20.90000000000000213, -1.885425182446133885, -11.59641995933507808 ) ) ;
#135865=DIRECTION ( 'NONE',  ( 0.000000000000000000, 0.1335171055202867274, -0.9910465087640866200 ) ) ;
#135868=AXIS2_PLACEMENT_3D ( 'NONE', #192886, #152495, #91216 ) ;
#135890=AXIS2_PLACEMENT_3D ( 'NONE', #237049, #19285, #257838 ) ;
#135891=CARTESIAN_POINT ( 'NONE',  ( -19.99999999999999645, 5.454087299794354138, 16.60000000000000142 ) ) ;
#136002=FACE_OUTER_BOUND ( 'NONE', #193393, .T. ) ;
#136056=AXIS2_PLACEMENT_3D ( 'NONE', #77177, #233706, #55030 ) ;
#136069=VERTEX_POINT ( 'NONE', #144007 ) ;
#136106=AXIS2_PLACEMENT_3D ( 'NONE', #164437, #243954, #182720 ) ;
#136135=ORIENTED_EDGE ( 'NONE', *, *, #56859, .T. ) ;
#136139=CARTESIAN_POINT ( 'NONE',  ( -18.69999999999999929, 5.488301202077016328, 16.39999999999999858 ) ) ;
#136146=CARTESIAN_POINT ( 'NONE',  ( -18.79999999999999716, -1.885425182446132997, -11.49641995933507843 ) ) ;
#136229=CARTESIAN_POINT ( 'NONE',  ( 0.8999999999999993561, -11.65000000000000036, 23.30000000000000426 ) ) ;
#136235=AXIS2_PLACEMENT_3D ( 'NONE', #162920, #121245, #142039 ) ;
#136277=ORIENTED_EDGE ( 'NONE', *, *, #29178, .T. ) ;
#136313=DIRECTION ( 'NONE',  ( 0.000000000000000000, 0.000000000000000000, 1.000000000000000000 ) ) ;
#136390=VECTOR ( 'NONE', #132510, 1000.000000000000000 ) ;
#136404=DIRECTION ( 'NONE',  ( 0.000000000000000000, 0.000000000000000000, -1.000000000000000000 ) ) ;
#136410=TOROIDAL_SURFACE ( 'NONE', #169814, 4.041421356237307805, 0.1000000000000000056 ) ;
#136467=DIRECTION ( 'NONE',  ( 0.000000000000000000, 0.000000000000000000, -1.000000000000000000 ) ) ;
#136470=CARTESIAN_POINT ( 'NONE',  ( -18.70000000000000284, -1.311673547813416718, -7.986648289447971116 ) ) ;
#136479=CIRCLE ( 'NONE', #61672, 3.900000000000000355 ) ;
#136581=ADVANCED_FACE ( 'NONE', ( #102607 ), #26984, .T. ) ;
#136603=CYLINDRICAL_SURFACE ( 'NONE', #195999, 0.09999999999999939493 ) ;
#136640=VERTEX_POINT ( 'NONE', #162627 ) ;
#136642=CIRCLE ( 'NONE', #215921, 0.1000000000000001860 ) ;
#136670=AXIS2_PLACEMENT_3D ( 'NONE', #10771, #150294, #207700 ) ;
#136688=EDGE_CURVE ( 'NONE', #248699, #59743, #106292, .T. ) ;
#136710=ORIENTED_EDGE ( 'NONE', *, *, #57290, .F. ) ;
#136717=AXIS2_PLACEMENT_3D ( 'NONE', #138467, #218007, #36865 ) ;
#136731=VERTEX_POINT ( 'NONE', #243429 ) ;
#136749=EDGE_LOOP ( 'NONE', ( #49608, #249970, #120562, #28424 ) ) ;
#136754=ORIENTED_EDGE ( 'NONE', *, *, #135292, .T. ) ;
#136790=FACE_OUTER_BOUND ( 'NONE', #73354, .T. ) ;
#136852=EDGE_CURVE ( 'NONE', #163445, #198523, #68729, .T. ) ;
#136957=DIRECTION ( 'NONE',  ( 0.000000000000000000, 0.000000000000000000, -1.000000000000000000 ) ) ;
#136962=ORIENTED_EDGE ( 'NONE', *, *, #217459, .F. ) ;
#136964=CARTESIAN_POINT ( 'NONE',  ( 5.899999999999996803, -11.75000000000000000, 14.00000000000000178 ) ) ;
#136968=DIRECTION ( 'NONE',  ( -1.000000000000000000, -0.000000000000000000, -0.000000000000000000 ) ) ;
#137004=VERTEX_POINT ( 'NONE', #220693 ) ;
#137038=DIRECTION ( 'NONE',  ( -0.000000000000000000, 0.000000000000000000, -1.000000000000000000 ) ) ;
#137040=CARTESIAN_POINT ( 'NONE',  ( 18.79999999999999716, -1.467286812112899463, 32.89999999999999858 ) ) ;
#137083=DIRECTION ( 'NONE',  ( 0.000000000000000000, 0.000000000000000000, -1.000000000000000000 ) ) ;
#137092=EDGE_CURVE ( 'NONE', #245477, #103483, #131454, .T. ) ;
#137120=EDGE_CURVE ( 'NONE', #56541, #252739, #194018, .T. ) ;
#137147=DIRECTION ( 'NONE',  ( 0.000000000000000000, 0.000000000000000000, -1.000000000000000000 ) ) ;
#137190=CARTESIAN_POINT ( 'NONE',  ( -20.90000000000000213, 1.901609089591594470, -11.59510167572422112 ) ) ;
#137194=CARTESIAN_POINT ( 'NONE',  ( -0.8999999999999993561, -11.75000000000000000, 28.70000000000000284 ) ) ;
#137216=CARTESIAN_POINT ( 'NONE',  ( -22.10000000000000142, -11.65000000000000036, 32.89999999999999858 ) ) ;
#137218=VECTOR ( 'NONE', #94600, 1000.000000000000000 ) ;
#137248=ORIENTED_EDGE ( 'NONE', *, *, #211260, .T. ) ;
#137249=SPHERICAL_SURFACE ( 'NONE', #121946, 0.1000000000000000056 ) ;
#137266=EDGE_LOOP ( 'NONE', ( #154300, #130103, #182948, #225225 ) ) ;
#137291=CARTESIAN_POINT ( 'NONE',  ( -18.59999999999999787, 11.75000000000000000, 31.39999999999999858 ) ) ;
#137304=ORIENTED_EDGE ( 'NONE', *, *, #63427, .F. ) ;
#137305=DIRECTION ( 'NONE',  ( -1.000000000000000000, 0.000000000000000000, 0.000000000000000000 ) ) ;
#137310=CARTESIAN_POINT ( 'NONE',  ( 18.79999999999999716, 13.48082180182240819, -2.152770446119436354 ) ) ;
#137318=SPHERICAL_SURFACE ( 'NONE', #169978, 0.1000000000000000056 ) ;
#137335=AXIS2_PLACEMENT_3D ( 'NONE', #177308, #93879, #74359 ) ;
#137346=ORIENTED_EDGE ( 'NONE', *, *, #44767, .T. ) ;
#137367=ORIENTED_EDGE ( 'NONE', *, *, #118417, .F. ) ;
#137403=DIRECTION ( 'NONE',  ( 0.000000000000000000, 0.000000000000000000, 1.000000000000000000 ) ) ;
#137405=DIRECTION ( 'NONE',  ( 0.000000000000000000, 0.000000000000000000, 1.000000000000000000 ) ) ;
#137406=CARTESIAN_POINT ( 'NONE',  ( 20.90000000000000213, 6.742993295648862961, 9.658650260582458458 ) ) ;
#137431=DIRECTION ( 'NONE',  ( -0.000000000000000000, -1.000000000000000000, 0.000000000000000000 ) ) ;
#137443=VECTOR ( 'NONE', #114028, 1000.000000000000000 ) ;
#137467=VERTEX_POINT ( 'NONE', #168156 ) ;
#137477=ORIENTED_EDGE ( 'NONE', *, *, #98510, .T. ) ;
#137478=DIRECTION ( 'NONE',  ( 0.000000000000000000, 0.000000000000000000, 1.000000000000000000 ) ) ;
#137507=LINE ( 'NONE', #217042, #163507 ) ;
#137519=ORIENTED_EDGE ( 'NONE', *, *, #255596, .T. ) ;
#137541=CARTESIAN_POINT ( 'NONE',  ( -18.59999999999999787, -10.84999999999999076, 33.00000000000000000 ) ) ;
#137543=EDGE_CURVE ( 'NONE', #113056, #78387, #254047, .T. ) ;
#137555=DIRECTION ( 'NONE',  ( 0.000000000000000000, 1.000000000000000000, 0.000000000000000000 ) ) ;
#137559=DIRECTION ( 'NONE',  ( 0.000000000000000000, -0.000000000000000000, -1.000000000000000000 ) ) ;
#137560=DIRECTION ( 'NONE',  ( 0.000000000000000000, 0.000000000000000000, 1.000000000000000000 ) ) ;
#137641=DIRECTION ( 'NONE',  ( 0.000000000000000000, 0.1618390714546066034, -0.9868171638914225996 ) ) ;
#137657=EDGE_CURVE ( 'NONE', #239783, #80656, #141801, .T. ) ;
#137668=DIRECTION ( 'NONE',  ( 0.000000000000000000, 0.000000000000000000, -1.000000000000000000 ) ) ;
#137695=CIRCLE ( 'NONE', #125266, 0.1000000000000000472 ) ;
#137696=DIRECTION ( 'NONE',  ( -1.000000000000000000, 0.000000000000000000, 0.000000000000000000 ) ) ;
#137709=CIRCLE ( 'NONE', #87827, 2.600000000000000089 ) ;
#137743=CIRCLE ( 'NONE', #29476, 0.1000000000000028644 ) ;
#137762=LINE ( 'NONE', #136470, #30424 ) ;
#137788=CARTESIAN_POINT ( 'NONE',  ( 13.39999999999999858, -11.75000000000000000, 17.70000000000000639 ) ) ;
#137821=EDGE_LOOP ( 'NONE', ( #53016, #177077, #118049, #197031 ) ) ;
#137878=EDGE_CURVE ( 'NONE', #10010, #99209, #165226, .T. ) ;
#137882=DIRECTION ( 'NONE',  ( -1.000000000000000000, 0.000000000000000000, 0.000000000000000000 ) ) ;
#137931=DIRECTION ( 'NONE',  ( 0.000000000000000000, 1.000000000000000000, 0.000000000000000000 ) ) ;
#137934=DIRECTION ( 'NONE',  ( 0.000000000000000000, 0.000000000000000000, 1.000000000000000000 ) ) ;
#137942=AXIS2_PLACEMENT_3D ( 'NONE', #162216, #217010, #38392 ) ;
#137945=LINE ( 'NONE', #217479, #76894 ) ;
#137964=AXIS2_PLACEMENT_3D ( 'NONE', #178190, #182019, #257631 ) ;
#137987=EDGE_LOOP ( 'NONE', ( #4630, #175991, #164677, #216902 ) ) ;
#138065=DIRECTION ( 'NONE',  ( -1.000000000000000000, -0.000000000000000000, -0.000000000000000000 ) ) ;
#138070=ORIENTED_EDGE ( 'NONE', *, *, #111451, .F. ) ;
#138084=CARTESIAN_POINT ( 'NONE',  ( 21.00000000000000000, 8.058024882095860875, 1.378482379536266178 ) ) ;
#138185=ORIENTED_EDGE ( 'NONE', *, *, #86847, .T. ) ;
#138279=FACE_BOUND ( 'NONE', #53913, .T. ) ;
#138295=EDGE_LOOP ( 'NONE', ( #253454, #131316, #210945, #70542 ) ) ;
#138326=DIRECTION ( 'NONE',  ( 0.000000000000000000, 0.000000000000000000, 1.000000000000000000 ) ) ;
#138342=ORIENTED_EDGE ( 'NONE', *, *, #207675, .F. ) ;
#138382=CYLINDRICAL_SURFACE ( 'NONE', #47380, 0.1000000000000028644 ) ;
#138412=AXIS2_PLACEMENT_3D ( 'NONE', #19135, #256395, #16594 ) ;
#138452=DIRECTION ( 'NONE',  ( -1.000000000000000000, 0.000000000000000000, 0.000000000000000000 ) ) ;
#138467=CARTESIAN_POINT ( 'NONE',  ( -13.40000000000000213, -11.75000000000000000, 15.00000000000000355 ) ) ;
#138485=ORIENTED_EDGE ( 'NONE', *, *, #98559, .F. ) ;
#138511=EDGE_CURVE ( 'NONE', #207660, #190676, #25125, .T. ) ;
#138530=CARTESIAN_POINT ( 'NONE',  ( -20.90000000000000213, -1.300000000000000044, -7.900000000000000355 ) ) ;
#138546=DIRECTION ( 'NONE',  ( 0.000000000000000000, -1.000000000000000000, 0.000000000000000000 ) ) ;
#138564=EDGE_LOOP ( 'NONE', ( #8168, #12788, #173336, #250883 ) ) ;
#138573=DIRECTION ( 'NONE',  ( 0.000000000000000000, 0.000000000000000000, 1.000000000000000000 ) ) ;
#138580=ORIENTED_EDGE ( 'NONE', *, *, #9516, .F. ) ;
#138581=CARTESIAN_POINT ( 'NONE',  ( -18.79999999999999716, 1.885425182446133885, -11.49641995933507843 ) ) ;
#138596=EDGE_CURVE ( 'NONE', #208096, #128297, #209721, .T. ) ;
#138651=ADVANCED_FACE ( 'NONE', ( #32531 ), #54610, .T. ) ;
#138668=DIRECTION ( 'NONE',  ( 0.000000000000000000, 0.000000000000000000, -1.000000000000000000 ) ) ;
#138678=CARTESIAN_POINT ( 'NONE',  ( 18.69999999999999929, 11.75000000000000000, -15.00000000000000000 ) ) ;
#138682=AXIS2_PLACEMENT_3D ( 'NONE', #14318, #54694, #55957 ) ;
#138721=EDGE_CURVE ( 'NONE', #257982, #223175, #147353, .T. ) ;
#138743=AXIS2_PLACEMENT_3D ( 'NONE', #255506, #155211, #13112 ) ;
#138751=AXIS2_PLACEMENT_3D ( 'NONE', #222719, #100191, #198030 ) ;
#138780=VERTEX_POINT ( 'NONE', #101392 ) ;
#138799=EDGE_CURVE ( 'NONE', #141175, #128297, #79294, .T. ) ;
#138812=EDGE_CURVE ( 'NONE', #195790, #22117, #22488, .T. ) ;
#138816=EDGE_LOOP ( 'NONE', ( #21409, #163817, #32182, #143522 ) ) ;
#138900=EDGE_LOOP ( 'NONE', ( #143791, #176627, #167452 ) ) ;
#138926=AXIS2_PLACEMENT_3D ( 'NONE', #177200, #80603, #97593 ) ;
#138932=ORIENTED_EDGE ( 'NONE', *, *, #57736, .F. ) ;
#138937=AXIS2_PLACEMENT_3D ( 'NONE', #235814, #173339, #71635 ) ;
#138983=ORIENTED_EDGE ( 'NONE', *, *, #225875, .F. ) ;
#139014=DIRECTION ( 'NONE',  ( 0.000000000000000000, -1.000000000000000000, 0.000000000000000000 ) ) ;
#139016=DIRECTION ( 'NONE',  ( 0.000000000000000000, 0.000000000000000000, 1.000000000000000000 ) ) ;
#139037=ORIENTED_EDGE ( 'NONE', *, *, #231964, .T. ) ;
#139046=EDGE_CURVE ( 'NONE', #60346, #224623, #131274, .T. ) ;
#139098=CARTESIAN_POINT ( 'NONE',  ( -21.00000000000000000, 8.000000000000000000, 1.212568896937007867 ) ) ;
#139145=CARTESIAN_POINT ( 'NONE',  ( -21.00000000000000000, -1.410778198689825347, -7.973296578895943121 ) ) ;
#139155=VERTEX_POINT ( 'NONE', #81537 ) ;
#139201=CARTESIAN_POINT ( 'NONE',  ( 18.59999999999999787, -9.849999999999996092, 31.39999999999999858 ) ) ;
#139223=EDGE_LOOP ( 'NONE', ( #125813, #3271, #208874, #93857 ) ) ;
#139237=DIRECTION ( 'NONE',  ( 1.000000000000000000, -0.000000000000000000, 0.000000000000000000 ) ) ;
#139260=LINE ( 'NONE', #244791, #2234 ) ;
#139356=CARTESIAN_POINT ( 'NONE',  ( 19.90000000000000924, 4.513204987021263825, 22.00000000000000355 ) ) ;
#139383=ORIENTED_EDGE ( 'NONE', *, *, #67992, .F. ) ;
#139401=CARTESIAN_POINT ( 'NONE',  ( 13.40000000000000036, -9.650000000000002132, 17.60000000000000497 ) ) ;
#139409=AXIS2_PLACEMENT_3D ( 'NONE', #107857, #8769, #49170 ) ;
#139445=SHAPE_DEFINITION_REPRESENTATION ( #132765, #205135 ) ;
#139449=ORIENTED_EDGE ( 'NONE', *, *, #138511, .T. ) ;
#139527=ORIENTED_EDGE ( 'NONE', *, *, #34931, .T. ) ;
#139535=ORIENTED_EDGE ( 'NONE', *, *, #48190, .F. ) ;
#139556=VERTEX_POINT ( 'NONE', #54002 ) ;
#139668=DIRECTION ( 'NONE',  ( 0.000000000000000000, 0.000000000000000000, -1.000000000000000000 ) ) ;
#139672=VECTOR ( 'NONE', #52041, 1000.000000000000000 ) ;
#139674=EDGE_LOOP ( 'NONE', ( #87634, #37595, #33123, #162048 ) ) ;
#139680=DIRECTION ( 'NONE',  ( 0.000000000000000000, 0.000000000000000000, 1.000000000000000000 ) ) ;
#139722=EDGE_LOOP ( 'NONE', ( #224885, #49877, #70051, #51283 ) ) ;
#139728=EDGE_CURVE ( 'NONE', #127870, #163992, #9958, .T. ) ;
#139736=AXIS2_PLACEMENT_3D ( 'NONE', #150734, #92035, #16378 ) ;
#139743=ORIENTED_EDGE ( 'NONE', *, *, #53020, .F. ) ;
#139759=ORIENTED_EDGE ( 'NONE', *, *, #94616, .F. ) ;
#139777=EDGE_CURVE ( 'NONE', #67059, #69468, #14085, .T. ) ;
#139790=CARTESIAN_POINT ( 'NONE',  ( 18.59999999999999787, -8.150000000000005684, 10.52591260281975138 ) ) ;
#139792=CARTESIAN_POINT ( 'NONE',  ( -22.19999999999999929, -11.75000000000000000, 32.89999999999999858 ) ) ;
#139802=AXIS2_PLACEMENT_3D ( 'NONE', #21610, #221066, #137668 ) ;
#139823=CYLINDRICAL_SURFACE ( 'NONE', #186662, 0.09999999999999939493 ) ;
#139855=CIRCLE ( 'NONE', #218970, 0.09999999999999939493 ) ;
#139859=ORIENTED_EDGE ( 'NONE', *, *, #233784, .T. ) ;
#139873=LINE ( 'NONE', #19964, #180721 ) ;
#139886=EDGE_CURVE ( 'NONE', #166883, #195496, #176577, .T. ) ;
#139892=AXIS2_PLACEMENT_3D ( 'NONE', #250718, #249462, #109919 ) ;
#139909=CARTESIAN_POINT ( 'NONE',  ( -20.90000000000000213, -1.212568896937008089, -7.800000000000000711 ) ) ;
#139912=DIRECTION ( 'NONE',  ( 0.000000000000000000, 0.000000000000000000, 1.000000000000000000 ) ) ;
#139926=ADVANCED_FACE ( 'NONE', ( #224539 ), #109548, .T. ) ;
#139936=ORIENTED_EDGE ( 'NONE', *, *, #223611, .F. ) ;
#140004=DIRECTION ( 'NONE',  ( 0.000000000000000000, 1.000000000000000000, 0.000000000000000000 ) ) ;
#140046=ORIENTED_EDGE ( 'NONE', *, *, #133360, .F. ) ;
#140064=ORIENTED_EDGE ( 'NONE', *, *, #137092, .F. ) ;
#140073=FACE_OUTER_BOUND ( 'NONE', #65560, .T. ) ;
#140091=VERTEX_POINT ( 'NONE', #255611 ) ;
#140096=AXIS2_PLACEMENT_3D ( 'NONE', #255464, #174747, #54741 ) ;
#140130=CYLINDRICAL_SURFACE ( 'NONE', #76298, 0.09999999999999939493 ) ;
#140138=CIRCLE ( 'NONE', #235821, 0.09999999999999939493 ) ;
#140191=ORIENTED_EDGE ( 'NONE', *, *, #171175, .T. ) ;
#140218=DIRECTION ( 'NONE',  ( -1.000000000000000000, 0.000000000000000000, 0.000000000000000000 ) ) ;
#140227=ORIENTED_EDGE ( 'NONE', *, *, #16982, .T. ) ;
#140324=LINE ( 'NONE', #239451, #35148 ) ;
#140359=DIRECTION ( 'NONE',  ( -0.000000000000000000, 0.000000000000000000, 1.000000000000000000 ) ) ;
#140368=ORIENTED_EDGE ( 'NONE', *, *, #44778, .T. ) ;
#140370=CARTESIAN_POINT ( 'NONE',  ( -20.90000000000000213, 11.61130914238355771, -1.800000000000000044 ) ) ;
#140382=DIRECTION ( 'NONE',  ( 0.000000000000000000, 1.000000000000000000, 0.000000000000000000 ) ) ;
#140383=CARTESIAN_POINT ( 'NONE',  ( -22.94999999999999929, 1.800000000000000044, -11.61130914238355771 ) ) ;
#140445=CARTESIAN_POINT ( 'NONE',  ( 5.999999999999995559, -11.34999999999999964, 10.10000000000000142 ) ) ;
#140459=CARTESIAN_POINT ( 'NONE',  ( 11.60000000000000142, -8.279289321881350361, 15.00000000000000355 ) ) ;
#140516=DIRECTION ( 'NONE',  ( -0.000000000000000000, 1.000000000000000000, -0.000000000000000000 ) ) ;
#140536=PLANE ( 'NONE',  #221004 ) ;
#140562=ADVANCED_FACE ( 'NONE', ( #101033 ), #80206, .F. ) ;
#140571=CARTESIAN_POINT ( 'NONE',  ( 13.40000000000000036, -8.250000000000005329, 15.00000000000000355 ) ) ;
#140626=CARTESIAN_POINT ( 'NONE',  ( -22.94999999999999929, 1.885425182446134107, -11.49641995933507843 ) ) ;
#140657=DIRECTION ( 'NONE',  ( -1.000000000000000000, 0.000000000000000000, 0.000000000000000000 ) ) ;
#140823=ORIENTED_EDGE ( 'NONE', *, *, #161606, .F. ) ;
#140826=DIRECTION ( 'NONE',  ( 1.000000000000000000, 0.000000000000000000, -2.168404344971008868E-16 ) ) ;
#140856=VECTOR ( 'NONE', #83921, 1000.000000000000114 ) ;
#140870=AXIS2_PLACEMENT_3D ( 'NONE', #67205, #103731, #204133 ) ;
#140904=CARTESIAN_POINT ( 'NONE',  ( 18.79999999999999716, 7.800000000000000711, -15.00000000000000000 ) ) ;
#140934=ORIENTED_EDGE ( 'NONE', *, *, #1141, .F. ) ;
#141047=DIRECTION ( 'NONE',  ( -0.000000000000000000, -0.000000000000000000, 1.000000000000000000 ) ) ;
#141091=CARTESIAN_POINT ( 'NONE',  ( 18.69999999999999929, -11.74999999999999289, 30.09999999999999787 ) ) ;
#141150=AXIS2_PLACEMENT_3D ( 'NONE', #69064, #148591, #237103 ) ;
#141168=ADVANCED_FACE ( 'NONE', ( #90188 ), #52347, .T. ) ;
#141175=VERTEX_POINT ( 'NONE', #171081 ) ;
#141231=ORIENTED_EDGE ( 'NONE', *, *, #7442, .F. ) ;
#141256=DIRECTION ( 'NONE',  ( -0.000000000000000000, 1.000000000000000000, -0.000000000000000000 ) ) ;
#141266=DIRECTION ( 'NONE',  ( -1.000000000000000000, 0.000000000000000000, 0.000000000000000000 ) ) ;
#141275=DIRECTION ( 'NONE',  ( 0.000000000000000000, 0.000000000000000000, -1.000000000000000000 ) ) ;
#141285=ADVANCED_FACE ( 'NONE', ( #160487 ), #61355, .T. ) ;
#141302=CARTESIAN_POINT ( 'NONE',  ( 20.10000000000000497, 5.572697453181475247, 16.49970471148372297 ) ) ;
#141340=ORIENTED_EDGE ( 'NONE', *, *, #13954, .T. ) ;
#141346=CARTESIAN_POINT ( 'NONE',  ( -18.79999999999999716, 1.212568896937007645, -8.000000000000000000 ) ) ;
#141349=EDGE_LOOP ( 'NONE', ( #148233, #218941, #119300 ) ) ;
#141359=VECTOR ( 'NONE', #234454, 1000.000000000000000 ) ;
#141361=VERTEX_POINT ( 'NONE', #83457 ) ;
#141362=DIRECTION ( 'NONE',  ( 0.000000000000000000, 1.000000000000000000, 0.000000000000000000 ) ) ;
#141376=EDGE_LOOP ( 'NONE', ( #42876, #72293, #6172, #255362 ) ) ;
#141389=ORIENTED_EDGE ( 'NONE', *, *, #169202, .T. ) ;
#141403=DIRECTION ( 'NONE',  ( 0.000000000000000000, -1.000000000000000000, 0.000000000000000000 ) ) ;
#141461=VECTOR ( 'NONE', #80019, 1000.000000000000000 ) ;
#141554=EDGE_CURVE ( 'NONE', #26765, #171566, #172050, .T. ) ;
#141583=ADVANCED_FACE ( 'NONE', ( #15531 ), #106344, .T. ) ;
#141694=CARTESIAN_POINT ( 'NONE',  ( 22.84999999999999787, 4.776122516674678272E-16, 3.900000000000000355 ) ) ;
#141699=DIRECTION ( 'NONE',  ( -1.000000000000000000, -0.000000000000000000, -0.000000000000000000 ) ) ;
#141720=EDGE_CURVE ( 'NONE', #188417, #254397, #65049, .T. ) ;
#141725=CARTESIAN_POINT ( 'NONE',  ( 18.79999999999999716, 1.350000000000000089, 21.90000000000000213 ) ) ;
#141743=ORIENTED_EDGE ( 'NONE', *, *, #87625, .T. ) ;
#141781=CARTESIAN_POINT ( 'NONE',  ( -18.79999999999999716, 6.742993295648862961, 9.658650260582458458 ) ) ;
#141801=LINE ( 'NONE', #235772, #176063 ) ;
#141846=DIRECTION ( 'NONE',  ( 1.000000000000000000, 0.000000000000000000, 0.000000000000000000 ) ) ;
#141929=DIRECTION ( 'NONE',  ( 0.000000000000000000, 0.000000000000000000, -1.000000000000000000 ) ) ;
#141995=DIRECTION ( 'NONE',  ( 1.284434275755705296E-16, -0.7071067811865471286, -0.7071067811865479058 ) ) ;
#142002=EDGE_CURVE ( 'NONE', #60954, #199798, #152378, .T. ) ;
#142039=DIRECTION ( 'NONE',  ( 0.000000000000000000, 0.000000000000000000, -1.000000000000000000 ) ) ;
#142067=DIRECTION ( 'NONE',  ( 0.000000000000000000, 0.000000000000000000, 1.000000000000000000 ) ) ;
#142092=ORIENTED_EDGE ( 'NONE', *, *, #111236, .T. ) ;
#142134=DIRECTION ( 'NONE',  ( 1.000000000000000000, -0.000000000000000000, -0.000000000000000000 ) ) ;
#142150=DIRECTION ( 'NONE',  ( 0.000000000000000000, 0.000000000000000000, 1.000000000000000000 ) ) ;
#142179=VERTEX_POINT ( 'NONE', #200252 ) ;
#142252=DIRECTION ( 'NONE',  ( 0.000000000000000000, -8.673617379884087537E-15, -1.000000000000000000 ) ) ;
#142289=CARTESIAN_POINT ( 'NONE',  ( 22.10000000000000497, -11.65000000000000036, 32.89999999999999858 ) ) ;
#142310=DIRECTION ( 'NONE',  ( -1.000000000000000000, 0.000000000000000000, 0.000000000000000000 ) ) ;
#142387=ORIENTED_EDGE ( 'NONE', *, *, #96767, .F. ) ;
#142423=EDGE_CURVE ( 'NONE', #114614, #80656, #119222, .T. ) ;
#142474=DIRECTION ( 'NONE',  ( 1.000000000000000000, 0.000000000000000000, 0.000000000000000000 ) ) ;
#142517=EDGE_LOOP ( 'NONE', ( #38753, #209592, #99361, #214724 ) ) ;
#142559=CARTESIAN_POINT ( 'NONE',  ( 18.79999999999999716, -1.885425182446133663, -11.49641995933507665 ) ) ;
#142569=DIRECTION ( 'NONE',  ( -1.000000000000000000, 0.000000000000000000, 0.000000000000000000 ) ) ;
#142579=DIRECTION ( 'NONE',  ( 0.000000000000000000, 0.000000000000000000, -1.000000000000000000 ) ) ;
#142600=DIRECTION ( 'NONE',  ( 0.000000000000000000, -1.000000000000000000, 0.000000000000000000 ) ) ;
#142634=ADVANCED_FACE ( 'NONE', ( #32581 ), #73635, .T. ) ;
#142652=LINE ( 'NONE', #83931, #133810 ) ;
#142667=CARTESIAN_POINT ( 'NONE',  ( 0.8999999999999993561, -11.75000000000000000, 26.00000000000000355 ) ) ;
#142680=AXIS2_PLACEMENT_3D ( 'NONE', #48183, #11652, #151157 ) ;
#142682=AXIS2_PLACEMENT_3D ( 'NONE', #127783, #245158, #246439 ) ;
#142732=DIRECTION ( 'NONE',  ( 0.000000000000000000, -1.000000000000000000, 0.000000000000000000 ) ) ;
#142765=ORIENTED_EDGE ( 'NONE', *, *, #182195, .T. ) ;
#142858=DIRECTION ( 'NONE',  ( 1.000000000000000000, -0.000000000000000000, -0.000000000000000000 ) ) ;
#142931=EDGE_CURVE ( 'NONE', #21663, #23059, #48837, .T. ) ;
#143005=CARTESIAN_POINT ( 'NONE',  ( -11.60000000000000320, -12.25000000000000178, 15.00000000000000355 ) ) ;
#143024=ORIENTED_EDGE ( 'NONE', *, *, #68088, .T. ) ;
#143099=DIRECTION ( 'NONE',  ( 0.000000000000000000, 1.000000000000000000, -0.000000000000000000 ) ) ;
#143130=CIRCLE ( 'NONE', #197305, 11.75000000000000000 ) ;
#143168=EDGE_CURVE ( 'NONE', #234077, #14935, #78243, .T. ) ;
#143181=ORIENTED_EDGE ( 'NONE', *, *, #227790, .T. ) ;
#143200=EDGE_CURVE ( 'NONE', #46601, #45320, #36095, .T. ) ;
#143208=ADVANCED_FACE ( 'NONE', ( #255060 ), #58182, .F. ) ;
#143284=ORIENTED_EDGE ( 'NONE', *, *, #11936, .F. ) ;
#143285=ADVANCED_FACE ( 'NONE', ( #197711 ), #19077, .T. ) ;
#143289=DIRECTION ( 'NONE',  ( -0.000000000000000000, -0.1335171055202901413, 0.9910465087640860649 ) ) ;
#143292=SPHERICAL_SURFACE ( 'NONE', #89717, 0.1000000000000000056 ) ;
#143304=FACE_OUTER_BOUND ( 'NONE', #754, .T. ) ;
#143314=AXIS2_PLACEMENT_3D ( 'NONE', #46838, #147238, #70307 ) ;
#143315=DIRECTION ( 'NONE',  ( -1.000000000000000000, 0.000000000000000000, 0.000000000000000000 ) ) ;
#143450=VECTOR ( 'NONE', #47094, 1000.000000000000114 ) ;
#143477=CARTESIAN_POINT ( 'NONE',  ( 18.79999999999999716, -11.65000000000000036, 5.900000000000001243 ) ) ;
#143478=ORIENTED_EDGE ( 'NONE', *, *, #176486, .T. ) ;
#143522=ORIENTED_EDGE ( 'NONE', *, *, #100875, .F. ) ;
#143573=CARTESIAN_POINT ( 'NONE',  ( 13.40000000000000036, -8.250000000000005329, 10.95857864376269575 ) ) ;
#143619=LINE ( 'NONE', #83611, #158534 ) ;
#143632=CYLINDRICAL_SURFACE ( 'NONE', #103466, 0.09999999999999939493 ) ;
#143699=CARTESIAN_POINT ( 'NONE',  ( 18.69999999999999929, -1.885425182446134107, -11.49641995933507843 ) ) ;
#143715=DIRECTION ( 'NONE',  ( 0.000000000000000000, -1.000000000000000000, 0.000000000000000000 ) ) ;
#143719=CARTESIAN_POINT ( 'NONE',  ( 21.00000000000000000, 0.3305886640091971196, 0.04453801223857078301 ) ) ;
#143725=VECTOR ( 'NONE', #59615, 1000.000000000000227 ) ;
#143732=ORIENTED_EDGE ( 'NONE', *, *, #207675, .T. ) ;
#143791=ORIENTED_EDGE ( 'NONE', *, *, #208992, .T. ) ;
#143805=FACE_OUTER_BOUND ( 'NONE', #137821, .T. ) ;
#143806=AXIS2_PLACEMENT_3D ( 'NONE', #173991, #33189, #213056 ) ;
#143875=CARTESIAN_POINT ( 'NONE',  ( 20.90000000000000213, -1.899104650876408451, -11.59795743183152972 ) ) ;
#143878=ADVANCED_FACE ( 'NONE', ( #122328 ), #238419, .F. ) ;
#143888=CARTESIAN_POINT ( 'NONE',  ( -20.90000000000000213, -1.901609089591594470, -11.59510167572422112 ) ) ;
#143917=TOROIDAL_SURFACE ( 'NONE', #227310, 0.2000000000000000111, 0.1000000000000000056 ) ;
#143921=CARTESIAN_POINT ( 'NONE',  ( -18.79999999999999716, 11.50977166988710820, 1.786320531569725478 ) ) ;
#143928=CARTESIAN_POINT ( 'NONE',  ( 20.90000000000000213, 1.311673547813416718, -7.986648289447971116 ) ) ;
#143930=AXIS2_PLACEMENT_3D ( 'NONE', #27605, #105786, #47104 ) ;
#143948=LINE ( 'NONE', #241767, #38169 ) ;
#143960=ADVANCED_FACE ( 'NONE', ( #49202 ), #148310, .T. ) ;
#143979=DIRECTION ( 'NONE',  ( 1.000000000000000000, -0.000000000000000000, 0.000000000000000000 ) ) ;
#143992=ORIENTED_EDGE ( 'NONE', *, *, #37285, .T. ) ;
#144007=CARTESIAN_POINT ( 'NONE',  ( 22.10000000000000142, -1.467286812112899463, 33.00000000000000000 ) ) ;
#144010=ADVANCED_FACE ( 'NONE', ( #243549 ), #123857, .T. ) ;
#144011=DIRECTION ( 'NONE',  ( 0.000000000000000000, 1.000000000000000000, 0.000000000000000000 ) ) ;
#144040=CARTESIAN_POINT ( 'NONE',  ( -20.90000000000000213, -1.786320531569725478, -11.50977166988710820 ) ) ;
#144153=DIRECTION ( 'NONE',  ( 0.000000000000000000, 0.000000000000000000, -1.000000000000000000 ) ) ;
#144181=ORIENTED_EDGE ( 'NONE', *, *, #171755, .F. ) ;
#144184=PRESENTATION_STYLE_ASSIGNMENT (( #64663 ) ) ;
#144252=VERTEX_POINT ( 'NONE', #236817 ) ;
#144272=CARTESIAN_POINT ( 'NONE',  ( -13.40000000000000213, -8.250000000000007105, 17.60000000000000497 ) ) ;
#144294=AXIS2_PLACEMENT_3D ( 'NONE', #193818, #95972, #56829 ) ;
#144349=CARTESIAN_POINT ( 'NONE',  ( -21.00000000000000000, -11.75000000000000000, 12.09999999999999609 ) ) ;
#144377=FACE_OUTER_BOUND ( 'NONE', #101140, .T. ) ;
#144393=DIRECTION ( 'NONE',  ( -0.000000000000000000, 1.000000000000000000, -0.000000000000000000 ) ) ;
#144506=ADVANCED_FACE ( 'NONE', ( #119153 ), #160858, .F. ) ;
#144507=DIRECTION ( 'NONE',  ( 0.000000000000000000, 0.9910465087640861759, 0.1335171055202901691 ) ) ;
#144512=DIRECTION ( 'NONE',  ( -1.000000000000000000, -0.000000000000000000, -0.000000000000000000 ) ) ;
#144514=DIRECTION ( 'NONE',  ( -0.000000000000000000, 0.9910465087640869530, 0.1335171055202841461 ) ) ;
#144570=EDGE_CURVE ( 'NONE', #190789, #245573, #182296, .T. ) ;
#144624=EDGE_CURVE ( 'NONE', #221991, #239783, #124045, .T. ) ;
#144632=EDGE_CURVE ( 'NONE', #1729, #73021, #132212, .T. ) ;
#144696=AXIS2_PLACEMENT_3D ( 'NONE', #126180, #7531, #4929 ) ;
#144700=FACE_OUTER_BOUND ( 'NONE', #208939, .T. ) ;
#144800=ORIENTED_EDGE ( 'NONE', *, *, #81555, .F. ) ;
#144810=ORIENTED_EDGE ( 'NONE', *, *, #68840, .T. ) ;
#144814=ADVANCED_BREP_SHAPE_REPRESENTATION ( '', ( #108017, #2425 ), #231390 ) ;
#144845=CARTESIAN_POINT ( 'NONE',  ( 18.59999999999999787, -9.849999999999990763, 31.39999999999999858 ) ) ;
#144847=DIRECTION ( 'NONE',  ( 0.000000000000000000, 1.000000000000000000, 0.000000000000000000 ) ) ;
#144860=EDGE_CURVE ( 'NONE', #203964, #209282, #31635, .T. ) ;
#144904=ADVANCED_FACE ( 'NONE', ( #212818 ), #151581, .T. ) ;
#144942=EDGE_LOOP ( 'NONE', ( #93316, #163701, #203052, #18127 ) ) ;
#144956=AXIS2_PLACEMENT_3D ( 'NONE', #42146, #160820, #179109 ) ;
#144975=VERTEX_POINT ( 'NONE', #19762 ) ;
#144978=CIRCLE ( 'NONE', #211823, 11.65000000000000036 ) ;
#144997=TOROIDAL_SURFACE ( 'NONE', #149137, 0.2000000000000000111, 0.1000000000000000056 ) ;
#145009=CARTESIAN_POINT ( 'NONE',  ( -19.89999999999999858, 5.586869315528661062, 16.41686199900910736 ) ) ;
#145018=AXIS2_PLACEMENT_3D ( 'NONE', #2318, #24493, #197963 ) ;
#145044=VERTEX_POINT ( 'NONE', #23633 ) ;
#145093=CIRCLE ( 'NONE', #220126, 0.1000000000000028644 ) ;
#145094=EDGE_CURVE ( 'NONE', #10423, #130825, #99242, .T. ) ;
#145128=EDGE_CURVE ( 'NONE', #47140, #223175, #46986, .T. ) ;
#145146=EDGE_CURVE ( 'NONE', #169815, #171633, #99430, .T. ) ;
#145169=EDGE_CURVE ( 'NONE', #8100, #49507, #257597, .T. ) ;
#145202=ORIENTED_EDGE ( 'NONE', *, *, #4267, .T. ) ;
#145331=AXIS2_PLACEMENT_3D ( 'NONE', #11082, #213124, #191025 ) ;
#145344=AXIS2_PLACEMENT_3D ( 'NONE', #162286, #113196, #14118 ) ;
#145418=CARTESIAN_POINT ( 'NONE',  ( 11.60000000000000142, -8.279289321881348584, 18.97071067811865674 ) ) ;
#145479=EDGE_CURVE ( 'NONE', #42394, #192176, #175337, .T. ) ;
#145492=DIRECTION ( 'NONE',  ( -1.000000000000000000, 0.000000000000000000, 0.000000000000000000 ) ) ;
#145510=AXIS2_PLACEMENT_3D ( 'NONE', #207213, #84633, #102937 ) ;
#145541=DIRECTION ( 'NONE',  ( -0.000000000000000000, 1.000000000000000000, -0.000000000000000000 ) ) ;
#145583=AXIS2_PLACEMENT_3D ( 'NONE', #9487, #69492, #249404 ) ;
#145603=AXIS2_PLACEMENT_3D ( 'NONE', #108885, #249691, #128457 ) ;
#145657=CARTESIAN_POINT ( 'NONE',  ( -20.09999999999999787, 4.547418889303922462, 21.90000000000000213 ) ) ;
#145664=PLANE ( 'NONE',  #186020 ) ;
#145686=ORIENTED_EDGE ( 'NONE', *, *, #231013, .F. ) ;
#145723=CYLINDRICAL_SURFACE ( 'NONE', #165562, 0.09999999999999939493 ) ;
#145740=FACE_OUTER_BOUND ( 'NONE', #186201, .T. ) ;
#145745=ORIENTED_EDGE ( 'NONE', *, *, #90536, .F. ) ;
#145750=DIRECTION ( 'NONE',  ( 0.000000000000000000, 0.000000000000000000, -1.000000000000000000 ) ) ;
#145870=EDGE_CURVE ( 'NONE', #49052, #173202, #33047, .T. ) ;
#145893=CARTESIAN_POINT ( 'NONE',  ( -20.90000000000000213, -1.212568896937008089, -8.000000000000000000 ) ) ;
#145920=AXIS2_PLACEMENT_3D ( 'NONE', #229840, #51169, #208990 ) ;
#145933=ADVANCED_FACE ( 'NONE', ( #14682 ), #13375, .T. ) ;
#145987=ORIENTED_EDGE ( 'NONE', *, *, #134984, .F. ) ;
#146012=EDGE_CURVE ( 'NONE', #25360, #89072, #214140, .T. ) ;
#146044=( BOUNDED_CURVE ( )  B_SPLINE_CURVE ( 3, ( #80977, #45720, #240080, #224354 ),
 .UNSPECIFIED., .F., .F. ) 
 B_SPLINE_CURVE_WITH_KNOTS ( ( 4, 4 ),
 ( 1.570796326794896558, 3.141592653589793116 ),
 .UNSPECIFIED. ) 
 CURVE ( )  GEOMETRIC_REPRESENTATION_ITEM ( )  RATIONAL_B_SPLINE_CURVE ( ( 1.000000000000000000, 0.8047378541243649375, 0.8047378541243649375, 1.000000000000000000 ) ) 
 REPRESENTATION_ITEM ( '' )  );
#146137=FACE_OUTER_BOUND ( 'NONE', #223210, .T. ) ;
#146140=ORIENTED_EDGE ( 'NONE', *, *, #194888, .T. ) ;
#146182=PLANE ( 'NONE',  #189731 ) ;
#146261=CIRCLE ( 'NONE', #230033, 0.1000000000000028644 ) ;
#146285=DIRECTION ( 'NONE',  ( 1.000000000000000000, -0.000000000000000000, -0.000000000000000000 ) ) ;
#146347=ORIENTED_EDGE ( 'NONE', *, *, #112902, .F. ) ;
#146374=ORIENTED_EDGE ( 'NONE', *, *, #136852, .F. ) ;
#146381=DIRECTION ( 'NONE',  ( 0.000000000000000000, 0.000000000000000000, -1.000000000000000000 ) ) ;
#146420=DIRECTION ( 'NONE',  ( -1.000000000000000000, -0.000000000000000000, 0.000000000000000000 ) ) ;
#146470=EDGE_CURVE ( 'NONE', #248444, #29621, #74901, .T. ) ;
#146495=ORIENTED_EDGE ( 'NONE', *, *, #134162, .F. ) ;
#146535=LINE ( 'NONE', #48734, #40757 ) ;
#146593=AXIS2_PLACEMENT_3D ( 'NONE', #95328, #54899, #157921 ) ;
#146622=AXIS2_PLACEMENT_3D ( 'NONE', #145657, #27042, #49131 ) ;
#146662=ORIENTED_EDGE ( 'NONE', *, *, #134654, .T. ) ;
#146682=CARTESIAN_POINT ( 'NONE',  ( 18.79999999999999716, 0.000000000000000000, 0.000000000000000000 ) ) ;
#146708=DIRECTION ( 'NONE',  ( -0.000000000000000000, -0.000000000000000000, 1.000000000000000000 ) ) ;
#146713=DIRECTION ( 'NONE',  ( 0.000000000000000000, -1.000000000000000000, 0.000000000000000000 ) ) ;
#146754=CARTESIAN_POINT ( 'NONE',  ( -18.59999999999999787, -10.74999999999999289, 31.59999999999999787 ) ) ;
#146793=ORIENTED_EDGE ( 'NONE', *, *, #36546, .T. ) ;
#146865=ADVANCED_FACE ( 'NONE', ( #130126 ), #31075, .T. ) ;
#146894=EDGE_CURVE ( 'NONE', #187034, #186207, #166857, .T. ) ;
#146946=DIRECTION ( 'NONE',  ( 0.000000000000000000, 0.000000000000000000, 1.000000000000000000 ) ) ;
#146996=EDGE_CURVE ( 'NONE', #104540, #129072, #201499, .T. ) ;
#147003=CARTESIAN_POINT ( 'NONE',  ( -18.79999999999999716, 0.000000000000000000, 0.000000000000000000 ) ) ;
#147010=AXIS2_PLACEMENT_3D ( 'NONE', #189021, #152490, #93760 ) ;
#147073=ORIENTED_EDGE ( 'NONE', *, *, #172509, .T. ) ;
#147074=VERTEX_POINT ( 'NONE', #52696 ) ;
#147096=AXIS2_PLACEMENT_3D ( 'NONE', #244173, #119119, #81243 ) ;
#147104=CIRCLE ( 'NONE', #63726, 0.09999999999999939493 ) ;
#147134=ADVANCED_FACE ( 'NONE', ( #214354 ), #100775, .T. ) ;
#147155=DIRECTION ( 'NONE',  ( -1.000000000000000000, -0.000000000000000000, 0.000000000000000000 ) ) ;
#147217=ORIENTED_EDGE ( 'NONE', *, *, #229644, .F. ) ;
#147222=CYLINDRICAL_SURFACE ( 'NONE', #30830, 2.599999999999998312 ) ;
#147238=DIRECTION ( 'NONE',  ( 0.000000000000000000, 1.000000000000000000, 0.000000000000000000 ) ) ;
#147251=ORIENTED_EDGE ( 'NONE', *, *, #186447, .F. ) ;
#147295=DIRECTION ( 'NONE',  ( -1.000000000000000000, 0.000000000000000000, -0.000000000000000000 ) ) ;
#147308=LINE ( 'NONE', #71645, #80609 ) ;
#147338=ORIENTED_EDGE ( 'NONE', *, *, #114043, .T. ) ;
#147353=CIRCLE ( 'NONE', #64163, 0.1000000000000002554 ) ;
#147381=CARTESIAN_POINT ( 'NONE',  ( -18.79999999999999716, 11.61130914238355771, 16.50000000000000000 ) ) ;
#147449=ADVANCED_FACE ( 'NONE', ( #209812 ), #210552, .T. ) ;
#147514=DIRECTION ( 'NONE',  ( -0.000000000000000000, 1.000000000000000000, -0.000000000000000000 ) ) ;
#147517=AXIS2_PLACEMENT_3D ( 'NONE', #236258, #34242, #212854 ) ;
#147524=ORIENTED_EDGE ( 'NONE', *, *, #237264, .F. ) ;
#147538=DIRECTION ( 'NONE',  ( 0.000000000000000000, 0.000000000000000000, 1.000000000000000000 ) ) ;
#147559=AXIS2_PLACEMENT_3D ( 'NONE', #2050, #164996, #180720 ) ;
#147573=CARTESIAN_POINT ( 'NONE',  ( 21.10000000000000142, 6.322468214605804882, 12.11686199900910310 ) ) ;
#147592=DIRECTION ( 'NONE',  ( 0.000000000000000000, -0.9910465087640866200, 0.1335171055202867274 ) ) ;
#147600=FACE_OUTER_BOUND ( 'NONE', #247557, .T. ) ;
#147630=CYLINDRICAL_SURFACE ( 'NONE', #205620, 0.09999999999999939493 ) ;
#147661=AXIS2_PLACEMENT_3D ( 'NONE', #63192, #142732, #43657 ) ;
#147704=EDGE_CURVE ( 'NONE', #182680, #168528, #218912, .T. ) ;
#147749=CARTESIAN_POINT ( 'NONE',  ( 5.899999999999991473, -11.25000000000000000, -2.558717127065786914E-15 ) ) ;
#147764=EDGE_CURVE ( 'NONE', #139155, #78394, #77431, .T. ) ;
#147765=ORIENTED_EDGE ( 'NONE', *, *, #21477, .F. ) ;
#147856=DIRECTION ( 'NONE',  ( 0.000000000000000000, -0.000000000000000000, 1.000000000000000000 ) ) ;
#147872=AXIS2_PLACEMENT_3D ( 'NONE', #60689, #158553, #62007 ) ;
#147893=CIRCLE ( 'NONE', #43650, 0.09999999999999939493 ) ;
#147921=AXIS2_PLACEMENT_3D ( 'NONE', #37585, #117110, #54556 ) ;
#147940=CARTESIAN_POINT ( 'NONE',  ( 0.9000000000000000222, -12.25000000000000355, 26.00000000000000355 ) ) ;
#147946=DIRECTION ( 'NONE',  ( 0.000000000000000000, 0.000000000000000000, 1.000000000000000000 ) ) ;
#147967=ORIENTED_EDGE ( 'NONE', *, *, #112716, .F. ) ;
#147987=AXIS2_PLACEMENT_3D ( 'NONE', #100081, #6126, #158830 ) ;
#148002=DIRECTION ( 'NONE',  ( 0.000000000000000000, 0.000000000000000000, 1.000000000000000000 ) ) ;
#148065=ORIENTED_EDGE ( 'NONE', *, *, #45110, .T. ) ;
#148078=DIRECTION ( 'NONE',  ( 0.000000000000000000, -0.000000000000000000, 1.000000000000000000 ) ) ;
#148079=DIRECTION ( 'NONE',  ( -1.000000000000000000, -0.000000000000000000, -0.000000000000000000 ) ) ;
#148086=VECTOR ( 'NONE', #193250, 1000.000000000000000 ) ;
#148175=FACE_OUTER_BOUND ( 'NONE', #128818, .T. ) ;
#148211=CIRCLE ( 'NONE', #135736, 0.09999999999999990841 ) ;
#148233=ORIENTED_EDGE ( 'NONE', *, *, #134145, .T. ) ;
#148237=AXIS2_PLACEMENT_3D ( 'NONE', #151821, #192223, #147946 ) ;
#148263=EDGE_LOOP ( 'NONE', ( #122597, #252536, #68136, #212785 ) ) ;
#148310=CYLINDRICAL_SURFACE ( 'NONE', #119583, 0.09999999999999939493 ) ;
#148312=CIRCLE ( 'NONE', #35908, 0.09999999999999993616 ) ;
#148366=ORIENTED_EDGE ( 'NONE', *, *, #95333, .F. ) ;
#148376=( LENGTH_UNIT ( ) NAMED_UNIT ( * ) SI_UNIT ( .MILLI., .METRE. ) );
#148387=DIRECTION ( 'NONE',  ( -1.000000000000000000, -0.000000000000000000, -0.000000000000000000 ) ) ;
#148427=DIRECTION ( 'NONE',  ( 0.000000000000000000, -0.1618390714546045217, -0.9868171638914230437 ) ) ;
#148509=ORIENTED_EDGE ( 'NONE', *, *, #196893, .T. ) ;
#148560=ADVANCED_FACE ( 'NONE', ( #18686 ), #201173, .T. ) ;
#148591=DIRECTION ( 'NONE',  ( -0.000000000000000000, -0.1618390714546045217, 0.9868171638914230437 ) ) ;
#148614=ORIENTED_EDGE ( 'NONE', *, *, #38500, .F. ) ;
#148622=ADVANCED_FACE ( 'NONE', ( #193189 ), #14557, .T. ) ;
#148652=ORIENTED_EDGE ( 'NONE', *, *, #108514, .F. ) ;
#148654=CARTESIAN_POINT ( 'NONE',  ( 18.59999999999999787, -10.84999999999999076, 32.89999999999999858 ) ) ;
#148673=EDGE_CURVE ( 'NONE', #87211, #101761, #85692, .T. ) ;
#148685=DIRECTION ( 'NONE',  ( -1.000000000000000000, 0.000000000000000000, 0.000000000000000000 ) ) ;
#148757=FACE_OUTER_BOUND ( 'NONE', #117446, .T. ) ;
#148782=CARTESIAN_POINT ( 'NONE',  ( -5.900000000000002132, -11.34999999999999964, 13.90000000000000213 ) ) ;
#148809=SPHERICAL_SURFACE ( 'NONE', #143930, 0.1000000000000000056 ) ;
#148816=AXIS2_PLACEMENT_3D ( 'NONE', #144845, #185275, #204816 ) ;
#148833=CARTESIAN_POINT ( 'NONE',  ( 18.79999999999999716, 3.461118860469513336, 28.84309995045515507 ) ) ;
#148834=FACE_OUTER_BOUND ( 'NONE', #72184, .T. ) ;
#148862=CIRCLE ( 'NONE', #36445, 0.09999999999999990841 ) ;
#148882=ORIENTED_EDGE ( 'NONE', *, *, #241288, .F. ) ;
#148893=DIRECTION ( 'NONE',  ( 0.000000000000000000, 0.000000000000000000, -1.000000000000000000 ) ) ;
#148926=CIRCLE ( 'NONE', #244578, 0.1000000000000001860 ) ;
#148956=CARTESIAN_POINT ( 'NONE',  ( -18.79999999999999716, -1.212568896937008089, -7.900000000000000355 ) ) ;
#148982=ORIENTED_EDGE ( 'NONE', *, *, #60668, .F. ) ;
#149009=ORIENTED_EDGE ( 'NONE', *, *, #194888, .F. ) ;
#149054=ORIENTED_EDGE ( 'NONE', *, *, #134976, .T. ) ;
#149087=DIRECTION ( 'NONE',  ( 1.000000000000000000, -0.000000000000000000, -0.000000000000000000 ) ) ;
#149134=ORIENTED_EDGE ( 'NONE', *, *, #184384, .T. ) ;
#149137=AXIS2_PLACEMENT_3D ( 'NONE', #176227, #197033, #255693 ) ;
#149173=DIRECTION ( 'NONE',  ( 0.000000000000000000, -0.7071067811865479058, 0.7071067811865472397 ) ) ;
#149210=ORIENTED_EDGE ( 'NONE', *, *, #54077, .T. ) ;
#149265=DIRECTION ( 'NONE',  ( 0.000000000000000000, 1.000000000000000000, -1.224646799147353207E-16 ) ) ;
#149267=DIRECTION ( 'NONE',  ( 0.000000000000000000, 0.1686199900910313187, -0.9856811345164828708 ) ) ;
#149270=CARTESIAN_POINT ( 'NONE',  ( -18.69999999999999929, -10.74999999999999289, 32.89999999999999858 ) ) ;
#149279=ORIENTED_EDGE ( 'NONE', *, *, #54973, .F. ) ;
#149285=VECTOR ( 'NONE', #40749, 1000.000000000000000 ) ;
#149305=SPHERICAL_SURFACE ( 'NONE', #165210, 0.1000000000000000056 ) ;
#149338=ORIENTED_EDGE ( 'NONE', *, *, #165111, .F. ) ;
#149370=VERTEX_POINT ( 'NONE', #252192 ) ;
#149431=DIRECTION ( 'NONE',  ( -0.000000000000000000, 0.1335171055202867274, -0.9910465087640865089 ) ) ;
#149434=DIRECTION ( 'NONE',  ( -0.000000000000000000, 0.000000000000000000, 1.000000000000000000 ) ) ;
#149447=CARTESIAN_POINT ( 'NONE',  ( -11.60000000000000320, -8.350000000000004974, 10.95857864376268864 ) ) ;
#149468=DIRECTION ( 'NONE',  ( 1.000000000000000000, 0.000000000000000000, 0.000000000000000000 ) ) ;
#149477=ORIENTED_EDGE ( 'NONE', *, *, #77889, .F. ) ;
#149508=CARTESIAN_POINT ( 'NONE',  ( 18.79999999999999361, -11.75000000000000000, 32.89999999999999858 ) ) ;
#149513=EDGE_LOOP ( 'NONE', ( #183890, #47558, #152301, #103546 ) ) ;
#149574=ADVANCED_FACE ( 'NONE', ( #126821 ), #61624, .T. ) ;
#149603=DIRECTION ( 'NONE',  ( -1.000000000000000000, 0.000000000000000000, 0.000000000000000000 ) ) ;
#149621=ORIENTED_EDGE ( 'NONE', *, *, #82486, .F. ) ;
#149638=VERTEX_POINT ( 'NONE', #208923 ) ;
#149664=CIRCLE ( 'NONE', #216081, 0.09999999999999939493 ) ;
#149688=CARTESIAN_POINT ( 'NONE',  ( -18.79999999999999716, -8.250000000000005329, 16.39999999999999858 ) ) ;
#149730=DIRECTION ( 'NONE',  ( -1.000000000000000000, 0.000000000000000000, 0.000000000000000000 ) ) ;
#149758=EDGE_CURVE ( 'NONE', #82204, #169606, #133239, .T. ) ;
#149772=ORIENTED_EDGE ( 'NONE', *, *, #91235, .F. ) ;
#149867=AXIS2_PLACEMENT_3D ( 'NONE', #12437, #148079, #48966 ) ;
#149899=AXIS2_PLACEMENT_3D ( 'NONE', #66505, #164330, #168210 ) ;
#149920=DIRECTION ( 'NONE',  ( 0.000000000000000000, 0.000000000000000000, 1.000000000000000000 ) ) ;
#149938=DIRECTION ( 'NONE',  ( 1.000000000000000000, -0.000000000000000000, -0.000000000000000000 ) ) ;
#149939=VERTEX_POINT ( 'NONE', #62694 ) ;
#149941=CIRCLE ( 'NONE', #112341, 11.75000000000000000 ) ;
#150016=ORIENTED_EDGE ( 'NONE', *, *, #202652, .T. ) ;
#150048=VECTOR ( 'NONE', #95525, 1000.000000000000000 ) ;
#150088=FACE_OUTER_BOUND ( 'NONE', #16198, .T. ) ;
#150119=CARTESIAN_POINT ( 'NONE',  ( 21.00000000000000000, 6.356682116888462630, 11.91686199900910381 ) ) ;
#150132=DIRECTION ( 'NONE',  ( 1.000000000000000000, 0.000000000000000000, 0.000000000000000000 ) ) ;
#150252=VERTEX_POINT ( 'NONE', #23281 ) ;
#150288=CIRCLE ( 'NONE', #237, 0.09999999999999939493 ) ;
#150294=DIRECTION ( 'NONE',  ( -3.712277463076317983E-14, -0.1686199900910448357, 0.9856811345164804283 ) ) ;
#150296=CARTESIAN_POINT ( 'NONE',  ( 18.79999999999999716, -1.800000000000000044, -11.61130914238355771 ) ) ;
#150303=ORIENTED_EDGE ( 'NONE', *, *, #102329, .T. ) ;
#150323=DIRECTION ( 'NONE',  ( 0.000000000000000000, 0.000000000000000000, 1.000000000000000000 ) ) ;
#150493=ORIENTED_EDGE ( 'NONE', *, *, #133590, .T. ) ;
#150529=VERTEX_POINT ( 'NONE', #55291 ) ;
#150539=AXIS2_PLACEMENT_3D ( 'NONE', #229069, #50392, #152114 ) ;
#150579=AXIS2_PLACEMENT_3D ( 'NONE', #202642, #25320, #160970 ) ;
#150585=VERTEX_POINT ( 'NONE', #257319 ) ;
#150632=TOROIDAL_SURFACE ( 'NONE', #250402, 0.2000000000000000111, 0.1000000000000000056 ) ;
#150719=CARTESIAN_POINT ( 'NONE',  ( -20.90000000000000213, -1.885425182446133885, -11.49641995933507843 ) ) ;
#150734=CARTESIAN_POINT ( 'NONE',  ( -22.10000000000000142, -1.467286812112899463, 28.00000000000000000 ) ) ;
#150778=ORIENTED_EDGE ( 'NONE', *, *, #145169, .F. ) ;
#150796=FACE_OUTER_BOUND ( 'NONE', #121104, .T. ) ;
#150816=EDGE_LOOP ( 'NONE', ( #39867, #168900, #201601, #137304 ) ) ;
#150901=DIRECTION ( 'NONE',  ( 0.000000000000000000, 0.000000000000000000, 1.000000000000000000 ) ) ;
#150924=CARTESIAN_POINT ( 'NONE',  ( -18.79999999999999716, -6.162641848847272286, 0.4936627796039583793 ) ) ;
#150930=CIRCLE ( 'NONE', #217538, 0.09999999999999939493 ) ;
#150936=ORIENTED_EDGE ( 'NONE', *, *, #251827, .T. ) ;
#150944=CARTESIAN_POINT ( 'NONE',  ( -18.79999999999999716, 6.841561409100513025, 9.675512259591560138 ) ) ;
#150950=ORIENTED_EDGE ( 'NONE', *, *, #172973, .T. ) ;
#150962=DIRECTION ( 'NONE',  ( 0.000000000000000000, -0.1686199900910312910, 0.9856811345164826488 ) ) ;
#150968=ADVANCED_FACE ( 'NONE', ( #36876 ), #118958, .T. ) ;
#150987=DIRECTION ( 'NONE',  ( 0.000000000000000000, -1.000000000000000000, 0.000000000000000000 ) ) ;
#150990=DIRECTION ( 'NONE',  ( 0.000000000000000000, 0.000000000000000000, -1.000000000000000000 ) ) ;
#151006=CARTESIAN_POINT ( 'NONE',  ( -11.60000000000000320, -9.650000000000005684, 17.60000000000000497 ) ) ;
#151030=DIRECTION ( 'NONE',  ( 0.000000000000000000, 0.000000000000000000, -1.000000000000000000 ) ) ;
#151032=ORIENTED_EDGE ( 'NONE', *, *, #26937, .F. ) ;
#151141=ADVANCED_FACE ( 'NONE', ( #211325 ), #67954, .F. ) ;
#151148=CIRCLE ( 'NONE', #147010, 4.100000000000000533 ) ;
#151157=DIRECTION ( 'NONE',  ( 0.000000000000000000, 0.000000000000000000, -1.000000000000000000 ) ) ;
#151293=ORIENTED_EDGE ( 'NONE', *, *, #97871, .T. ) ;
#151312=DIRECTION ( 'NONE',  ( 0.000000000000000000, 0.000000000000000000, -1.000000000000000000 ) ) ;
#151454=DIRECTION ( 'NONE',  ( 0.000000000000000000, 0.000000000000000000, 1.000000000000000000 ) ) ;
#151484=CARTESIAN_POINT ( 'NONE',  ( -18.79999999999999716, -1.885425182446133885, -11.49641995933507843 ) ) ;
#151485=EDGE_CURVE ( 'NONE', #244339, #47140, #207174, .T. ) ;
#151500=AXIS2_PLACEMENT_3D ( 'NONE', #196059, #73567, #237743 ) ;
#151505=ORIENTED_EDGE ( 'NONE', *, *, #7808, .T. ) ;
#151581=CYLINDRICAL_SURFACE ( 'NONE', #186592, 0.09999999999999939493 ) ;
#151603=AXIS2_PLACEMENT_3D ( 'NONE', #121643, #64215, #83733 ) ;
#151634=LINE ( 'NONE', #132038, #52778 ) ;
#151654=CARTESIAN_POINT ( 'NONE',  ( 22.84999999999999787, 0.000000000000000000, 4.000000000000000000 ) ) ;
#151674=CARTESIAN_POINT ( 'NONE',  ( -18.59999999999999787, -11.65000000000000036, 5.900000000000001243 ) ) ;
#151681=EDGE_CURVE ( 'NONE', #150529, #132306, #191172, .T. ) ;
#151749=AXIS2_PLACEMENT_3D ( 'NONE', #238387, #233286, #58443 ) ;
#151769=DIRECTION ( 'NONE',  ( 0.000000000000000000, 0.000000000000000000, -1.000000000000000000 ) ) ;
#151770=ADVANCED_FACE ( 'NONE', ( #166160 ), #124437, .T. ) ;
#151785=VECTOR ( 'NONE', #3219, 1000.000000000000114 ) ;
#151799=ORIENTED_EDGE ( 'NONE', *, *, #94090, .T. ) ;
#151808=CARTESIAN_POINT ( 'NONE',  ( 0.8999999999999993561, -8.350000000000004974, 26.00000000000000355 ) ) ;
#151809=EDGE_CURVE ( 'NONE', #74968, #232547, #87074, .T. ) ;
#151821=CARTESIAN_POINT ( 'NONE',  ( 18.79999999999999716, 11.49641995933507843, -1.885425182446133885 ) ) ;
#151824=EDGE_CURVE ( 'NONE', #188417, #49823, #149664, .T. ) ;
#151825=AXIS2_PLACEMENT_3D ( 'NONE', #253864, #175643, #156099 ) ;
#151919=CARTESIAN_POINT ( 'NONE',  ( -20.90000000000000213, 7.900000000000000355, -1.300000000000000044 ) ) ;
#151942=EDGE_LOOP ( 'NONE', ( #129661, #95175, #248849, #161388 ) ) ;
#152010=VECTOR ( 'NONE', #204359, 1000.000000000000000 ) ;
#152076=LINE ( 'NONE', #206892, #188714 ) ;
#152107=CARTESIAN_POINT ( 'NONE',  ( 20.90000000000000213, 7.800000000000000711, -1.212568896937008089 ) ) ;
#152114=DIRECTION ( 'NONE',  ( 1.476360405086644309E-16, 1.000000000000000000, 0.000000000000000000 ) ) ;
#152135=CARTESIAN_POINT ( 'NONE',  ( 11.60000000000000142, -8.350000000000004974, 15.00000000000000355 ) ) ;
#152153=EDGE_CURVE ( 'NONE', #129607, #10810, #233052, .T. ) ;
#152222=LINE ( 'NONE', #153526, #257493 ) ;
#152235=DIRECTION ( 'NONE',  ( 0.000000000000000000, -0.9910465087640861759, 0.1335171055202901691 ) ) ;
#152252=PRESENTATION_STYLE_ASSIGNMENT (( #229205 ) ) ;
#152283=CARTESIAN_POINT ( 'NONE',  ( 21.10000000000000142, -11.65000000000000036, 12.09999999999999609 ) ) ;
#152295=ADVANCED_FACE ( 'NONE', ( #249213 ), #203797, .T. ) ;
#152301=ORIENTED_EDGE ( 'NONE', *, *, #165471, .F. ) ;
#152304=EDGE_CURVE ( 'NONE', #156269, #25377, #13170, .T. ) ;
#152332=CARTESIAN_POINT ( 'NONE',  ( 18.59999999999999787, -9.749999999999994671, 30.00000000000000000 ) ) ;
#152373=DIRECTION ( 'NONE',  ( 0.000000000000000000, 0.000000000000000000, -1.000000000000000000 ) ) ;
#152378=CIRCLE ( 'NONE', #202420, 0.1000000000000002554 ) ;
#152429=EDGE_CURVE ( 'NONE', #57698, #186207, #174821, .T. ) ;
#152457=ORIENTED_EDGE ( 'NONE', *, *, #125913, .T. ) ;
#152460=CARTESIAN_POINT ( 'NONE',  ( 22.10000000000000497, 11.99999999999999822, 12.00000000000000000 ) ) ;
#152466=EDGE_CURVE ( 'NONE', #103588, #219544, #62530, .T. ) ;
#152487=ORIENTED_EDGE ( 'NONE', *, *, #245743, .T. ) ;
#152490=DIRECTION ( 'NONE',  ( -1.000000000000000000, -0.000000000000000000, -0.000000000000000000 ) ) ;
#152492=VERTEX_POINT ( 'NONE', #199521 ) ;
#152495=DIRECTION ( 'NONE',  ( 2.933373889701419960E-15, -0.8164989248600479366, 0.5773469543544730298 ) ) ;
#152518=AXIS2_PLACEMENT_3D ( 'NONE', #63980, #183925, #84785 ) ;
#152551=DIRECTION ( 'NONE',  ( 0.000000000000000000, 0.000000000000000000, -1.000000000000000000 ) ) ;
#152578=CARTESIAN_POINT ( 'NONE',  ( -22.94999999999999929, 6.322468214605804882, 12.11686199900910488 ) ) ;
#152619=DIRECTION ( 'NONE',  ( 0.000000000000000000, 0.000000000000000000, -1.000000000000000000 ) ) ;
#152625=CARTESIAN_POINT ( 'NONE',  ( 21.04142135623731136, 6.223900101154154818, 12.00000000000000000 ) ) ;
#152630=CARTESIAN_POINT ( 'NONE',  ( 21.10000000000000142, 0.000000000000000000, 0.000000000000000000 ) ) ;
#152645=CYLINDRICAL_SURFACE ( 'NONE', #215039, 0.09999999999999939493 ) ;
#152674=LINE ( 'NONE', #69268, #224148 ) ;
#152707=CARTESIAN_POINT ( 'NONE',  ( -20.90000000000000213, 1.212568896937007645, -8.000000000000000000 ) ) ;
#152724=ORIENTED_EDGE ( 'NONE', *, *, #195482, .T. ) ;
#152771=AXIS2_PLACEMENT_3D ( 'NONE', #25963, #88463, #168078 ) ;
#152774=DIRECTION ( 'NONE',  ( 0.000000000000000000, 0.000000000000000000, -1.000000000000000000 ) ) ;
#152792=EDGE_CURVE ( 'NONE', #103483, #3738, #74142, .T. ) ;
#152803=EDGE_LOOP ( 'NONE', ( #1243, #229335, #117795, #161615 ) ) ;
#152804=DIRECTION ( 'NONE',  ( -1.000000000000000000, -0.000000000000000000, -0.000000000000000000 ) ) ;
#152805=ORIENTED_EDGE ( 'NONE', *, *, #221632, .T. ) ;
#152816=PLANE ( 'NONE',  #71813 ) ;
#152843=EDGE_CURVE ( 'NONE', #166926, #71198, #71096, .T. ) ;
#152953=AXIS2_PLACEMENT_3D ( 'NONE', #187816, #148685, #112135 ) ;
#152974=CARTESIAN_POINT ( 'NONE',  ( 18.79999999999999361, -11.75000000000000000, 30.00000000000000000 ) ) ;
#152988=DIRECTION ( 'NONE',  ( 1.000000000000000000, 0.000000000000000000, 0.000000000000000000 ) ) ;
#153025=CARTESIAN_POINT ( 'NONE',  ( 18.79999999999999716, 3.362550747017865493, 28.82623795144604983 ) ) ;
#153049=AXIS2_PLACEMENT_3D ( 'NONE', #72552, #112950, #213313 ) ;
#153057=CYLINDRICAL_SURFACE ( 'NONE', #67096, 0.09999999999999939493 ) ;
#153074=DIRECTION ( 'NONE',  ( -0.000000000000000000, 1.000000000000000000, -0.000000000000000000 ) ) ;
#153098=AXIS2_PLACEMENT_3D ( 'NONE', #254469, #75865, #97966 ) ;
#153175=DIRECTION ( 'NONE',  ( 0.000000000000000000, 0.1335171055202901413, -0.9910465087640860649 ) ) ;
#153176=EDGE_CURVE ( 'NONE', #160025, #245624, #25305, .T. ) ;
#153206=CARTESIAN_POINT ( 'NONE',  ( -20.90000000000000213, 6.726092018229619107, 9.512212474619550662 ) ) ;
#153227=EDGE_CURVE ( 'NONE', #12989, #209609, #191743, .T. ) ;
#153260=AXIS2_PLACEMENT_3D ( 'NONE', #180444, #140004, #81300 ) ;
#153345=DIRECTION ( 'NONE',  ( 0.000000000000000000, -0.000000000000000000, -1.000000000000000000 ) ) ;
#153370=EDGE_LOOP ( 'NONE', ( #3619, #1677, #143732, #239583 ) ) ;
#153383=FACE_OUTER_BOUND ( 'NONE', #141376, .T. ) ;
#153395=DIRECTION ( 'NONE',  ( -1.000000000000000000, 0.000000000000000000, 0.000000000000000000 ) ) ;
#153397=CIRCLE ( 'NONE', #128416, 0.09999999999999939493 ) ;
#153448=ORIENTED_EDGE ( 'NONE', *, *, #182700, .T. ) ;
#153509=ORIENTED_EDGE ( 'NONE', *, *, #91939, .T. ) ;
#153513=CARTESIAN_POINT ( 'NONE',  ( 0.000000000000000000, 0.000000000000000000, 0.000000000000000000 ) ) ;
#153526=CARTESIAN_POINT ( 'NONE',  ( -20.09999999999999787, 3.461118860469513336, 28.84309995045515507 ) ) ;
#153528=EDGE_LOOP ( 'NONE', ( #19897, #27792, #185592, #57131 ) ) ;
#153530=ORIENTED_EDGE ( 'NONE', *, *, #190122, .T. ) ;
#153562=AXIS2_PLACEMENT_3D ( 'NONE', #133591, #253530, #254778 ) ;
#153630=AXIS2_PLACEMENT_3D ( 'NONE', #70470, #165701, #50836 ) ;
#153642=CARTESIAN_POINT ( 'NONE',  ( -19.89999999999999858, 4.631764625546179737, 22.00000000000000355 ) ) ;
#153678=DIRECTION ( 'NONE',  ( 0.000000000000000000, -1.000000000000000000, 0.000000000000000000 ) ) ;
#153757=EDGE_LOOP ( 'NONE', ( #212545, #140227, #147251 ) ) ;
#153759=SPHERICAL_SURFACE ( 'NONE', #189397, 0.1000000000000000056 ) ;
#153783=EDGE_LOOP ( 'NONE', ( #196092, #109237, #28197, #77112 ) ) ;
#153792=EDGE_CURVE ( 'NONE', #139556, #166926, #225493, .T. ) ;
#153875=LINE ( 'NONE', #209957, #206560 ) ;
#153882=EDGE_CURVE ( 'NONE', #19574, #29111, #192827, .T. ) ;
#153931=VECTOR ( 'NONE', #229038, 1000.000000000000000 ) ;
#153988=DIRECTION ( 'NONE',  ( 0.000000000000000000, 0.000000000000000000, 1.000000000000000000 ) ) ;
#153993=CARTESIAN_POINT ( 'NONE',  ( 18.69999999999999929, -11.65000000000000036, 0.000000000000000000 ) ) ;
#154004=EDGE_CURVE ( 'NONE', #60346, #98150, #225537, .T. ) ;
#154020=DIRECTION ( 'NONE',  ( -1.000000000000000000, 0.000000000000000000, 0.000000000000000000 ) ) ;
#154045=CIRCLE ( 'NONE', #4146, 0.1000000000000000472 ) ;
#154077=DIRECTION ( 'NONE',  ( 1.000000000000000000, 0.000000000000000000, 0.000000000000000000 ) ) ;
#154092=DIRECTION ( 'NONE',  ( 1.000000000000000000, 0.000000000000000000, 0.000000000000000000 ) ) ;
#154132=ORIENTED_EDGE ( 'NONE', *, *, #62343, .F. ) ;
#154142=CARTESIAN_POINT ( 'NONE',  ( 18.79999999999999716, 1.410778198689825125, -7.973296578895943121 ) ) ;
#154179=EDGE_CURVE ( 'NONE', #37930, #73948, #13201, .T. ) ;
#154197=DIRECTION ( 'NONE',  ( 1.000000000000000000, -0.000000000000000000, -0.000000000000000000 ) ) ;
#154225=AXIS2_PLACEMENT_3D ( 'NONE', #107418, #85252, #70896 ) ;
#154260=ORIENTED_EDGE ( 'NONE', *, *, #151485, .T. ) ;
#154268=ADVANCED_FACE ( 'NONE', ( #133803 ), #246419, .T. ) ;
#154293=LINE ( 'NONE', #215493, #211685 ) ;
#154300=ORIENTED_EDGE ( 'NONE', *, *, #28789, .T. ) ;
#154308=DIRECTION ( 'NONE',  ( 0.000000000000000000, -1.000000000000000000, 0.000000000000000000 ) ) ;
#154314=DIRECTION ( 'NONE',  ( -1.000000000000000000, -0.000000000000000000, -0.000000000000000000 ) ) ;
#154321=FACE_OUTER_BOUND ( 'NONE', #134298, .T. ) ;
#154336=CARTESIAN_POINT ( 'NONE',  ( 11.60000000000000320, -12.24999999999999822, 15.00000000000000355 ) ) ;
#154343=ORIENTED_EDGE ( 'NONE', *, *, #171769, .F. ) ;
#154393=CARTESIAN_POINT ( 'NONE',  ( 18.79999999999999716, -1.467286812112899463, 33.00000000000000000 ) ) ;
#154452=CARTESIAN_POINT ( 'NONE',  ( -22.10000000000000142, -1.467286812112899463, 32.89999999999999858 ) ) ;
#154482=FACE_OUTER_BOUND ( 'NONE', #185007, .T. ) ;
#154588=ORIENTED_EDGE ( 'NONE', *, *, #36224, .T. ) ;
#154593=DIRECTION ( 'NONE',  ( 1.000000000000000000, 0.000000000000000000, 0.000000000000000000 ) ) ;
#154604=DIRECTION ( 'NONE',  ( 1.000000000000000000, 0.000000000000000000, 0.000000000000000000 ) ) ;
#154659=CIRCLE ( 'NONE', #63029, 0.1000000000000000472 ) ;
#154676=VERTEX_POINT ( 'NONE', #50241 ) ;
#154704=ADVANCED_FACE ( 'NONE', ( #17534 ), #34569, .T. ) ;
#154758=EDGE_CURVE ( 'NONE', #224002, #126102, #117922, .T. ) ;
#154781=DIRECTION ( 'NONE',  ( 5.850181106597693140E-15, -0.1686199900910279881, 0.9856811345164833149 ) ) ;
#154815=CYLINDRICAL_SURFACE ( 'NONE', #200157, 4.000000000000000000 ) ;
#154821=EDGE_LOOP ( 'NONE', ( #225828, #98031, #156610, #54356 ) ) ;
#154842=CARTESIAN_POINT ( 'NONE',  ( 0.8999999999999993561, -9.650000000000003908, 28.60000000000000142 ) ) ;
#154879=CARTESIAN_POINT ( 'NONE',  ( 5.899999999999995914, -11.65000000000000036, 10.10000000000000142 ) ) ;
#154896=CARTESIAN_POINT ( 'NONE',  ( -21.10000000000000142, 6.322468214605803993, 12.11686199900910488 ) ) ;
#154900=LINE ( 'NONE', #210998, #92995 ) ;
#154925=DIRECTION ( 'NONE',  ( -1.000000000000000000, 0.000000000000000000, 0.000000000000000000 ) ) ;
#154938=ORIENTED_EDGE ( 'NONE', *, *, #181279, .F. ) ;
#154979=AXIS2_PLACEMENT_3D ( 'NONE', #4438, #576, #64433 ) ;
#155051=FACE_OUTER_BOUND ( 'NONE', #257773, .T. ) ;
#155054=AXIS2_PLACEMENT_3D ( 'NONE', #209374, #13747, #251056 ) ;
#155056=VERTEX_POINT ( 'NONE', #137190 ) ;
#155107=DIRECTION ( 'NONE',  ( 1.158076286952576634E-15, -0.1335171055202867274, -0.9910465087640865089 ) ) ;
#155115=CARTESIAN_POINT ( 'NONE',  ( 22.94999999999999929, 0.000000000000000000, 0.000000000000000000 ) ) ;
#155145=AXIS2_PLACEMENT_3D ( 'NONE', #203218, #44161, #220235 ) ;
#155210=ORIENTED_EDGE ( 'NONE', *, *, #29398, .T. ) ;
#155211=DIRECTION ( 'NONE',  ( 1.000000000000000000, -0.000000000000000000, -0.000000000000000000 ) ) ;
#155226=DIRECTION ( 'NONE',  ( -8.673617379884087537E-15, -1.000000000000000000, 0.000000000000000000 ) ) ;
#155256=FACE_OUTER_BOUND ( 'NONE', #123156, .T. ) ;
#155286=LINE ( 'NONE', #136964, #30215 ) ;
#155302=ORIENTED_EDGE ( 'NONE', *, *, #193313, .F. ) ;
#155328=DIRECTION ( 'NONE',  ( 1.000000000000000000, 0.000000000000000000, 0.000000000000000000 ) ) ;
#155343=DIRECTION ( 'NONE',  ( 1.000000000000000000, -0.000000000000000000, -0.000000000000000000 ) ) ;
#155357=CIRCLE ( 'NONE', #226191, 0.1000000000000000472 ) ;
#155430=ORIENTED_EDGE ( 'NONE', *, *, #173357, .T. ) ;
#155498=DIRECTION ( 'NONE',  ( 0.000000000000000000, -0.000000000000000000, 1.000000000000000000 ) ) ;
#155516=CARTESIAN_POINT ( 'NONE',  ( 18.79999999999999716, 1.885425182446133885, -11.49641995933507843 ) ) ;
#155522=ORIENTED_EDGE ( 'NONE', *, *, #168222, .T. ) ;
#155530=EDGE_LOOP ( 'NONE', ( #59633, #251490, #3657, #116813 ) ) ;
#155553=ADVANCED_FACE ( 'NONE', ( #173511 ), #4754, .T. ) ;
#155628=CIRCLE ( 'NONE', #180544, 0.09999999999999939493 ) ;
#155646=CARTESIAN_POINT ( 'NONE',  ( 18.69999999999999929, 1.410778198689825125, -7.973296578895943121 ) ) ;
#155651=CYLINDRICAL_SURFACE ( 'NONE', #107558, 0.09999999999999939493 ) ;
#155660=CIRCLE ( 'NONE', #247195, 0.2000000000000005107 ) ;
#155666=ADVANCED_FACE ( 'NONE', ( #101579 ), #18234, .F. ) ;
#155685=AXIS2_PLACEMENT_3D ( 'NONE', #226453, #189929, #73865 ) ;
#155686=ORIENTED_EDGE ( 'NONE', *, *, #145169, .T. ) ;
#155708=VERTEX_POINT ( 'NONE', #68932 ) ;
#155731=FACE_OUTER_BOUND ( 'NONE', #252213, .T. ) ;
#155762=EDGE_CURVE ( 'NONE', #203870, #171566, #17605, .T. ) ;
#155773=ADVANCED_FACE ( 'NONE', ( #143304 ), #227985, .T. ) ;
#155840=EDGE_CURVE ( 'NONE', #154676, #47981, #42567, .T. ) ;
#155858=AXIS2_PLACEMENT_3D ( 'NONE', #10671, #221023, #204985 ) ;
#155859=ORIENTED_EDGE ( 'NONE', *, *, #26730, .T. ) ;
#155865=DIRECTION ( 'NONE',  ( 1.000000000000000000, 0.000000000000000000, 0.000000000000000000 ) ) ;
#155878=DIRECTION ( 'NONE',  ( 1.000000000000000000, -0.000000000000000000, 0.000000000000000000 ) ) ;
#155887=ORIENTED_EDGE ( 'NONE', *, *, #44573, .F. ) ;
#155913=EDGE_CURVE ( 'NONE', #78593, #194417, #134008, .T. ) ;
#155921=ADVANCED_FACE ( 'NONE', ( #253943 ), #43303, .T. ) ;
#155955=DIRECTION ( 'NONE',  ( 0.000000000000000000, 0.000000000000000000, 1.000000000000000000 ) ) ;
#156099=DIRECTION ( 'NONE',  ( 0.000000000000000000, -0.9910465087640866200, -0.1335171055202867274 ) ) ;
#156104=CIRCLE ( 'NONE', #127033, 0.09999999999999939493 ) ;
#156123=ORIENTED_EDGE ( 'NONE', *, *, #130147, .T. ) ;
#156171=CARTESIAN_POINT ( 'NONE',  ( 18.79999999999999716, -1.901609089591594470, -11.59510167572422112 ) ) ;
#156181=ADVANCED_FACE ( 'NONE', ( #205526 ), #66027, .T. ) ;
#156184=VERTEX_POINT ( 'NONE', #25625 ) ;
#156190=EDGE_CURVE ( 'NONE', #98368, #256387, #165132, .T. ) ;
#156213=CIRCLE ( 'NONE', #160490, 0.1999999999999996503 ) ;
#156214=ORIENTED_EDGE ( 'NONE', *, *, #79383, .T. ) ;
#156216=DIRECTION ( 'NONE',  ( 0.000000000000000000, 0.000000000000000000, 1.000000000000000000 ) ) ;
#156268=CARTESIAN_POINT ( 'NONE',  ( 5.899999999999995914, -11.34999999999999964, 10.10000000000000142 ) ) ;
#156269=VERTEX_POINT ( 'NONE', #188543 ) ;
#156319=ORIENTED_EDGE ( 'NONE', *, *, #68840, .F. ) ;
#156404=CARTESIAN_POINT ( 'NONE',  ( 0.8999999999999993561, -8.250000000000005329, 28.60000000000000142 ) ) ;
#156417=DIRECTION ( 'NONE',  ( 0.000000000000000000, -1.000000000000000000, 0.000000000000000000 ) ) ;
#156430=CARTESIAN_POINT ( 'NONE',  ( -18.59999999999999787, -9.849999999999994316, 30.09999999999999076 ) ) ;
#156595=ORIENTED_EDGE ( 'NONE', *, *, #95248, .T. ) ;
#156610=ORIENTED_EDGE ( 'NONE', *, *, #63052, .F. ) ;
#156701=ORIENTED_EDGE ( 'NONE', *, *, #111257, .F. ) ;
#156742=CARTESIAN_POINT ( 'NONE',  ( -20.90000000000000213, -11.75000000000000000, -15.00000000000000000 ) ) ;
#156771=ORIENTED_EDGE ( 'NONE', *, *, #237569, .F. ) ;
#156794=FACE_OUTER_BOUND ( 'NONE', #99552, .T. ) ;
#156837=LINE ( 'NONE', #199805, #87070 ) ;
#156872=VERTEX_POINT ( 'NONE', #50645 ) ;
#156915=DIRECTION ( 'NONE',  ( 0.000000000000000000, 0.000000000000000000, -1.000000000000000000 ) ) ;
#156960=VECTOR ( 'NONE', #254509, 1000.000000000000000 ) ;
#156964=DIRECTION ( 'NONE',  ( -1.000000000000000000, 0.000000000000000000, 0.000000000000000000 ) ) ;
#156989=ORIENTED_EDGE ( 'NONE', *, *, #139728, .T. ) ;
#157054=EDGE_CURVE ( 'NONE', #237894, #69570, #251436, .T. ) ;
#157086=CARTESIAN_POINT ( 'NONE',  ( 22.10000000000000142, -11.65000000000000036, 12.09999999999999787 ) ) ;
#157107=FACE_OUTER_BOUND ( 'NONE', #161935, .T. ) ;
#157121=EDGE_CURVE ( 'NONE', #223778, #57698, #257795, .T. ) ;
#157122=CARTESIAN_POINT ( 'NONE',  ( 20.00000000000000355, 5.645774302107834153, 15.47947886955507890 ) ) ;
#157123=DIRECTION ( 'NONE',  ( 0.000000000000000000, 0.000000000000000000, -1.000000000000000000 ) ) ;
#157148=CARTESIAN_POINT ( 'NONE',  ( 18.79999999999999716, 6.644425182197215562, 9.641788261573355001 ) ) ;
#157180=ORIENTED_EDGE ( 'NONE', *, *, #36304, .T. ) ;
#157206=CARTESIAN_POINT ( 'NONE',  ( -22.94999999999999929, 3.461118860469513336, 28.84309995045515507 ) ) ;
#157221=DIRECTION ( 'NONE',  ( 0.000000000000000000, 0.000000000000000000, -1.000000000000000000 ) ) ;
#157234=CARTESIAN_POINT ( 'NONE',  ( -22.10000000000000497, 6.322468214605804882, 12.11686199900910310 ) ) ;
#157239=CARTESIAN_POINT ( 'NONE',  ( 18.79999999999999716, -1.885425182446133885, -11.49641995933507843 ) ) ;
#157254=CARTESIAN_POINT ( 'NONE',  ( -18.69999999999999929, -8.250000000000005329, 31.39999999999999858 ) ) ;
#157255=DIRECTION ( 'NONE',  ( 1.000000000000000000, 0.000000000000000000, 0.000000000000000000 ) ) ;
#157281=EDGE_LOOP ( 'NONE', ( #18013, #113086, #64495, #66727 ) ) ;
#157333=DIRECTION ( 'NONE',  ( 0.000000000000000000, -1.000000000000000000, 0.000000000000000000 ) ) ;
#157342=ORIENTED_EDGE ( 'NONE', *, *, #42817, .F. ) ;
#157354=LINE ( 'NONE', #97305, #495 ) ;
#157369=LINE ( 'NONE', #80325, #210800 ) ;
#157376=FACE_OUTER_BOUND ( 'NONE', #192591, .T. ) ;
#157377=DIRECTION ( 'NONE',  ( 0.000000000000000000, 0.000000000000000000, 1.000000000000000000 ) ) ;
#157385=ORIENTED_EDGE ( 'NONE', *, *, #168943, .T. ) ;
#157431=CARTESIAN_POINT ( 'NONE',  ( 20.00000000000000355, 1.350000000000000089, 16.50000000000000000 ) ) ;
#157498=DIRECTION ( 'NONE',  ( 0.000000000000000000, 0.000000000000000000, 1.000000000000000000 ) ) ;
#157505=EDGE_CURVE ( 'NONE', #15770, #254139, #193602, .T. ) ;
#157511=FACE_OUTER_BOUND ( 'NONE', #124570, .T. ) ;
#157537=DIRECTION ( 'NONE',  ( 0.000000000000000000, -0.9868171638914230437, -0.1618390714546045217 ) ) ;
#157541=CARTESIAN_POINT ( 'NONE',  ( 18.79999999999999716, 4.513204987021263825, 22.10000000000000142 ) ) ;
#157545=VERTEX_POINT ( 'NONE', #161023 ) ;
#157564=VERTEX_POINT ( 'NONE', #80150 ) ;
#157578=DIRECTION ( 'NONE',  ( 1.000000000000000000, 0.000000000000000000, 0.000000000000000000 ) ) ;
#157589=EDGE_LOOP ( 'NONE', ( #119430, #30062, #132411 ) ) ;
#157627=CARTESIAN_POINT ( 'NONE',  ( -19.99999999999999645, 4.513204987021263825, 22.00000000000000355 ) ) ;
#157666=DIRECTION ( 'NONE',  ( 0.000000000000000000, 0.000000000000000000, -1.000000000000000000 ) ) ;
#157696=FACE_OUTER_BOUND ( 'NONE', #155530, .T. ) ;
#157725=DIRECTION ( 'NONE',  ( 4.336808689942043611E-14, -1.000000000000000000, -0.000000000000000000 ) ) ;
#157791=DIRECTION ( 'NONE',  ( 0.000000000000000000, -1.000000000000000000, -1.445602896647339410E-16 ) ) ;
#157810=CARTESIAN_POINT ( 'NONE',  ( 11.60000000000000320, -9.650000000000002132, 17.60000000000000497 ) ) ;
#157820=ORIENTED_EDGE ( 'NONE', *, *, #95333, .T. ) ;
#157863=ORIENTED_EDGE ( 'NONE', *, *, #130128, .T. ) ;
#157883=CARTESIAN_POINT ( 'NONE',  ( 20.90000000000000213, 1.212568896937007645, -7.900000000000000355 ) ) ;
#157921=DIRECTION ( 'NONE',  ( 0.000000000000000000, 0.000000000000000000, -1.000000000000000000 ) ) ;
#158009=VERTEX_POINT ( 'NONE', #143573 ) ;
#158023=CARTESIAN_POINT ( 'NONE',  ( -22.19999999999999929, -11.65000000000000036, 6.100000000000001421 ) ) ;
#158027=ORIENTED_EDGE ( 'NONE', *, *, #18943, .F. ) ;
#158031=ORIENTED_EDGE ( 'NONE', *, *, #87441, .T. ) ;
#158034=EDGE_CURVE ( 'NONE', #60346, #120003, #156213, .T. ) ;
#158097=PLANE ( 'NONE',  #18975 ) ;
#158098=DIRECTION ( 'NONE',  ( 0.000000000000000000, 0.000000000000000000, 1.000000000000000000 ) ) ;
#158132=DIRECTION ( 'NONE',  ( 0.000000000000000000, 1.000000000000000000, 0.000000000000000000 ) ) ;
#158178=CARTESIAN_POINT ( 'NONE',  ( -18.79999999999999716, 1.350000000000000089, 21.90000000000000213 ) ) ;
#158211=ORIENTED_EDGE ( 'NONE', *, *, #144632, .F. ) ;
#158304=CARTESIAN_POINT ( 'NONE',  ( 0.8999999999999993561, -8.279289321881350361, 26.00000000000000355 ) ) ;
#158310=DIRECTION ( 'NONE',  ( 1.000000000000000000, 0.000000000000000000, 0.000000000000000000 ) ) ;
#158336=CARTESIAN_POINT ( 'NONE',  ( 18.69999999999999929, -11.75000000000000000, 6.100000000000001421 ) ) ;
#158380=DIRECTION ( 'NONE',  ( 8.673617379884087537E-15, 1.000000000000000000, 0.000000000000000000 ) ) ;
#158490=CARTESIAN_POINT ( 'NONE',  ( -19.89999999999999858, 1.250000000000000000, 21.90000000000000213 ) ) ;
#158534=VECTOR ( 'NONE', #16315, 1000.000000000000000 ) ;
#158539=EDGE_CURVE ( 'NONE', #45068, #105564, #256432, .T. ) ;
#158553=DIRECTION ( 'NONE',  ( -1.000000000000000000, 0.000000000000000000, 0.000000000000000000 ) ) ;
#158564=ORIENTED_EDGE ( 'NONE', *, *, #143168, .F. ) ;
#158566=VERTEX_POINT ( 'NONE', #174651 ) ;
#158591=AXIS2_PLACEMENT_3D ( 'NONE', #98037, #78492, #158098 ) ;
#158600=DIRECTION ( 'NONE',  ( 0.000000000000000000, 0.000000000000000000, 1.000000000000000000 ) ) ;
#158603=LINE ( 'NONE', #213401, #201713 ) ;
#158611=DIRECTION ( 'NONE',  ( 0.000000000000000000, 1.000000000000000000, 1.224646799147353207E-16 ) ) ;
#158621=DIRECTION ( 'NONE',  ( 0.000000000000000000, 0.000000000000000000, 1.000000000000000000 ) ) ;
#158626=EDGE_LOOP ( 'NONE', ( #213891, #10555, #140368 ) ) ;
#158630=CARTESIAN_POINT ( 'NONE',  ( 20.99999999999998934, 7.900000000000000355, 1.212568896937007867 ) ) ;
#158652=VECTOR ( 'NONE', #124552, 1000.000000000000000 ) ;
#158688=DIRECTION ( 'NONE',  ( 0.000000000000000000, 1.000000000000000000, 0.000000000000000000 ) ) ;
#158700=CIRCLE ( 'NONE', #225267, 4.000000000000000000 ) ;
#158706=CARTESIAN_POINT ( 'NONE',  ( 20.00889983613310719, 5.561941060815491333, 16.56258203121810268 ) ) ;
#158715=VECTOR ( 'NONE', #26216, 1000.000000000000000 ) ;
#158737=LINE ( 'NONE', #77869, #221426 ) ;
#158748=ORIENTED_EDGE ( 'NONE', *, *, #215515, .F. ) ;
#158755=VECTOR ( 'NONE', #252293, 1000.000000000000000 ) ;
#158830=DIRECTION ( 'NONE',  ( 0.000000000000000000, 0.000000000000000000, -1.000000000000000000 ) ) ;
#158839=CARTESIAN_POINT ( 'NONE',  ( 18.79999999999999716, 5.488301202077013663, 16.39999999999999858 ) ) ;
#158884=EDGE_CURVE ( 'NONE', #215604, #137004, #87019, .T. ) ;
#158899=EDGE_CURVE ( 'NONE', #221804, #131374, #85772, .T. ) ;
#159023=LINE ( 'NONE', #199423, #99357 ) ;
#159030=VERTEX_POINT ( 'NONE', #145418 ) ;
#159116=AXIS2_PLACEMENT_3D ( 'NONE', #169467, #108176, #186433 ) ;
#159133=ORIENTED_EDGE ( 'NONE', *, *, #136688, .F. ) ;
#159169=ORIENTED_EDGE ( 'NONE', *, *, #110517, .F. ) ;
#159177=ORIENTED_EDGE ( 'NONE', *, *, #229119, .T. ) ;
#159181=CARTESIAN_POINT ( 'NONE',  ( 22.10000000000000497, -11.75000000000000000, 12.09999999999999609 ) ) ;
#159192=ADVANCED_FACE ( 'NONE', ( #224947 ), #198428, .T. ) ;
#159204=ORIENTED_EDGE ( 'NONE', *, *, #206297, .T. ) ;
#159206=ORIENTED_EDGE ( 'NONE', *, *, #117720, .F. ) ;
#159213=EDGE_CURVE ( 'NONE', #106026, #66961, #56732, .T. ) ;
#159278=AXIS2_PLACEMENT_3D ( 'NONE', #190381, #112130, #230792 ) ;
#159328=AXIS2_PLACEMENT_3D ( 'NONE', #96903, #61670, #79909 ) ;
#159386=DIRECTION ( 'NONE',  ( 0.000000000000000000, -0.000000000000000000, 1.000000000000000000 ) ) ;
#159398=FACE_OUTER_BOUND ( 'NONE', #194439, .T. ) ;
#159462=AXIS2_PLACEMENT_3D ( 'NONE', #172224, #174790, #14410 ) ;
#159480=LINE ( 'NONE', #35700, #93071 ) ;
#159487=AXIS2_PLACEMENT_3D ( 'NONE', #97231, #77693, #59393 ) ;
#159514=DIRECTION ( 'NONE',  ( -0.000000000000000000, 1.000000000000000000, 0.000000000000000000 ) ) ;
#159534=CIRCLE ( 'NONE', #26263, 0.1999999999999987899 ) ;
#159540=AXIS2_PLACEMENT_3D ( 'NONE', #218381, #39802, #180569 ) ;
#159549=ORIENTED_EDGE ( 'NONE', *, *, #216849, .T. ) ;
#159561=DIRECTION ( 'NONE',  ( 1.000000000000000000, 0.000000000000000000, 0.000000000000000000 ) ) ;
#159573=ORIENTED_EDGE ( 'NONE', *, *, #57963, .F. ) ;
#159580=ADVANCED_FACE ( 'NONE', ( #157696 ), #255408, .T. ) ;
#159582=AXIS2_PLACEMENT_3D ( 'NONE', #174182, #35930, #115436 ) ;
#159599=AXIS2_PLACEMENT_3D ( 'NONE', #178674, #79512, #153988 ) ;
#159602=DIRECTION ( 'NONE',  ( -1.000000000000000000, 0.000000000000000000, 0.000000000000000000 ) ) ;
#159603=VECTOR ( 'NONE', #110262, 1000.000000000000000 ) ;
#159607=CARTESIAN_POINT ( 'NONE',  ( 6.099999999999998757, -11.75000000000000000, 10.10000000000000142 ) ) ;
#159723=DIRECTION ( 'NONE',  ( 1.000000000000000000, -0.000000000000000000, -0.000000000000000000 ) ) ;
#159724=DIRECTION ( 'NONE',  ( 0.000000000000000000, 0.000000000000000000, -1.000000000000000000 ) ) ;
#159733=ORIENTED_EDGE ( 'NONE', *, *, #54897, .F. ) ;
#159738=EDGE_LOOP ( 'NONE', ( #211460, #53742, #85270, #61907 ) ) ;
#159824=PLANE ( 'NONE',  #24285 ) ;
#159886=AXIS2_PLACEMENT_3D ( 'NONE', #217184, #38571, #63251 ) ;
#159918=ORIENTED_EDGE ( 'NONE', *, *, #68146, .F. ) ;
#159945=AXIS2_PLACEMENT_3D ( 'NONE', #181278, #200824, #24781 ) ;
#159989=DIRECTION ( 'NONE',  ( 0.000000000000000000, -0.9910465087640860649, -0.1335171055202901413 ) ) ;
#160004=FACE_OUTER_BOUND ( 'NONE', #157281, .T. ) ;
#160009=AXIS2_PLACEMENT_3D ( 'NONE', #28930, #150132, #168446 ) ;
#160025=VERTEX_POINT ( 'NONE', #180756 ) ;
#160089=ORIENTED_EDGE ( 'NONE', *, *, #183764, .F. ) ;
#160097=DIRECTION ( 'NONE',  ( -1.000000000000000000, -0.000000000000000000, -0.000000000000000000 ) ) ;
#160149=DIRECTION ( 'NONE',  ( 0.000000000000000000, -1.000000000000000000, 0.000000000000000000 ) ) ;
#160152=ORIENTED_EDGE ( 'NONE', *, *, #51416, .T. ) ;
#160167=CARTESIAN_POINT ( 'NONE',  ( -21.00000000000000000, 6.841561409100513025, 9.675512259591560138 ) ) ;
#160210=ORIENTED_EDGE ( 'NONE', *, *, #190122, .F. ) ;
#160242=ORIENTED_EDGE ( 'NONE', *, *, #244998, .T. ) ;
#160244=AXIS2_PLACEMENT_3D ( 'NONE', #186500, #189060, #6562 ) ;
#160292=AXIS2_PLACEMENT_3D ( 'NONE', #120364, #19960, #199883 ) ;
#160310=AXIS2_PLACEMENT_3D ( 'NONE', #83691, #163288, #64180 ) ;
#160468=DIRECTION ( 'NONE',  ( -1.000000000000000000, 0.000000000000000000, -0.000000000000000000 ) ) ;
#160487=FACE_OUTER_BOUND ( 'NONE', #36708, .T. ) ;
#160490=AXIS2_PLACEMENT_3D ( 'NONE', #45754, #186571, #26211 ) ;
#160514=CARTESIAN_POINT ( 'NONE',  ( 20.90000000000000213, 11.59510167572422112, -1.901609089591594470 ) ) ;
#160524=ORIENTED_EDGE ( 'NONE', *, *, #233549, .F. ) ;
#160570=AXIS2_PLACEMENT_3D ( 'NONE', #55515, #37298, #38565 ) ;
#160587=DIRECTION ( 'NONE',  ( 1.000000000000000000, 0.000000000000000000, 0.000000000000000000 ) ) ;
#160667=DIRECTION ( 'NONE',  ( 0.000000000000000000, 0.000000000000000000, -1.000000000000000000 ) ) ;
#160772=DIRECTION ( 'NONE',  ( -0.000000000000000000, 1.000000000000000000, 0.000000000000000000 ) ) ;
#160820=DIRECTION ( 'NONE',  ( 1.476360405086644309E-16, -1.000000000000000000, -1.445602896647339410E-16 ) ) ;
#160844=AXIS2_PLACEMENT_3D ( 'NONE', #15722, #208769, #193054 ) ;
#160858=SPHERICAL_SURFACE ( 'NONE', #7312, 0.1000000000000000056 ) ;
#160906=ORIENTED_EDGE ( 'NONE', *, *, #253646, .T. ) ;
#160911=VERTEX_POINT ( 'NONE', #208716 ) ;
#160925=FACE_OUTER_BOUND ( 'NONE', #209979, .T. ) ;
#160947=SPHERICAL_SURFACE ( 'NONE', #246963, 0.1000000000000000056 ) ;
#160970=DIRECTION ( 'NONE',  ( 0.000000000000000000, 0.9856811345164829818, 0.1686199900910294314 ) ) ;
#160987=CARTESIAN_POINT ( 'NONE',  ( -22.94999999999999929, 11.59510167572422112, -1.901609089591594692 ) ) ;
#161004=CARTESIAN_POINT ( 'NONE',  ( 20.89999999999999503, 8.000000000000000000, 1.212568896937007867 ) ) ;
#161013=DIRECTION ( 'NONE',  ( 1.000000000000000000, 0.000000000000000000, 0.000000000000000000 ) ) ;
#161023=CARTESIAN_POINT ( 'NONE',  ( 18.79999999999999716, 1.786320531569725478, -11.50977166988710820 ) ) ;
#161141=EDGE_CURVE ( 'NONE', #245477, #207912, #159023, .T. ) ;
#161179=DIRECTION ( 'NONE',  ( 0.000000000000000000, -1.000000000000000000, 0.000000000000000000 ) ) ;
#161215=CARTESIAN_POINT ( 'NONE',  ( -21.00000000000000000, 6.258114003436814343, 11.90000000000000036 ) ) ;
#161222=VECTOR ( 'NONE', #64044, 1000.000000000000000 ) ;
#161267=AXIS2_PLACEMENT_3D ( 'NONE', #25203, #104677, #166010 ) ;
#161315=CARTESIAN_POINT ( 'NONE',  ( 20.90000000000000213, -1.885425182446133885, -11.49641995933507843 ) ) ;
#161345=CARTESIAN_POINT ( 'NONE',  ( -22.94999999999999929, 1.901609089591594692, -11.59510167572422112 ) ) ;
#161346=CARTESIAN_POINT ( 'NONE',  ( 18.79999999999999716, -11.65000000000000036, 32.89999999999999858 ) ) ;
#161364=ORIENTED_EDGE ( 'NONE', *, *, #56704, .T. ) ;
#161388=ORIENTED_EDGE ( 'NONE', *, *, #230794, .F. ) ;
#161391=LINE ( 'NONE', #119696, #72464 ) ;
#161419=AXIS2_PLACEMENT_3D ( 'NONE', #60108, #40605, #1419 ) ;
#161437=VERTEX_POINT ( 'NONE', #95791 ) ;
#161442=SPHERICAL_SURFACE ( 'NONE', #43568, 0.1000000000000000056 ) ;
#161443=CARTESIAN_POINT ( 'NONE',  ( 18.69999999999999929, 11.75000000000000000, 32.89999999999999858 ) ) ;
#161465=CARTESIAN_POINT ( 'NONE',  ( -20.90000000000000213, -1.885425182446134107, -11.59641995933507808 ) ) ;
#161524=CARTESIAN_POINT ( 'NONE',  ( 21.00000000000000000, -1.212568896937008089, -8.000000000000000000 ) ) ;
#161550=LINE ( 'NONE', #184940, #88438 ) ;
#161554=VERTEX_POINT ( 'NONE', #201333 ) ;
#161606=EDGE_CURVE ( 'NONE', #208096, #192900, #243714, .T. ) ;
#161615=ORIENTED_EDGE ( 'NONE', *, *, #92015, .F. ) ;
#161619=CARTESIAN_POINT ( 'NONE',  ( -22.94999999999999929, 11.99999999999999822, 12.00000000000000000 ) ) ;
#161623=DIRECTION ( 'NONE',  ( -0.000000000000000000, 0.9910465087640865089, 0.1335171055202867274 ) ) ;
#161633=ORIENTED_EDGE ( 'NONE', *, *, #226193, .T. ) ;
#161654=CARTESIAN_POINT ( 'NONE',  ( 11.60000000000000142, -8.250000000000003553, 15.00000000000000355 ) ) ;
#161727=LINE ( 'NONE', #117442, #173863 ) ;
#161738=CIRCLE ( 'NONE', #32753, 0.09999999999999990841 ) ;
#161768=VECTOR ( 'NONE', #232598, 1000.000000000000000 ) ;
#161770=ORIENTED_EDGE ( 'NONE', *, *, #70003, .F. ) ;
#161780=VECTOR ( 'NONE', #118957, 1000.000000000000000 ) ;
#161809=CIRCLE ( 'NONE', #145018, 0.09999999999999939493 ) ;
#161886=CARTESIAN_POINT ( 'NONE',  ( -21.00000000000000000, 6.223900101154156594, 12.00000000000000000 ) ) ;
#161906=AXIS2_PLACEMENT_3D ( 'NONE', #50846, #211234, #113419 ) ;
#161935=EDGE_LOOP ( 'NONE', ( #185858, #217069, #138485, #157180 ) ) ;
#161969=VECTOR ( 'NONE', #217714, 1000.000000000000000 ) ;
#161994=ORIENTED_EDGE ( 'NONE', *, *, #42561, .T. ) ;
#162045=DIRECTION ( 'NONE',  ( -1.000000000000000000, 0.000000000000000000, 0.000000000000000000 ) ) ;
#162048=ORIENTED_EDGE ( 'NONE', *, *, #245877, .F. ) ;
#162114=EDGE_LOOP ( 'NONE', ( #101619, #134397, #149772 ) ) ;
#162127=AXIS2_PLACEMENT_3D ( 'NONE', #139790, #177684, #96797 ) ;
#162166=EDGE_CURVE ( 'NONE', #76531, #219544, #29524, .T. ) ;
#162187=DIRECTION ( 'NONE',  ( 1.000000000000000000, -0.000000000000000000, -0.000000000000000000 ) ) ;
#162195=AXIS2_PLACEMENT_3D ( 'NONE', #132027, #92889, #53774 ) ;
#162216=CARTESIAN_POINT ( 'NONE',  ( 18.69999999999999929, 8.000000000000000000, 1.212568896937007867 ) ) ;
#162286=CARTESIAN_POINT ( 'NONE',  ( -18.59999999999999787, -10.63400887967554986, 6.002871413764276909 ) ) ;
#162293=ORIENTED_EDGE ( 'NONE', *, *, #111160, .F. ) ;
#162299=AXIS2_PLACEMENT_3D ( 'NONE', #246805, #212842, #113727 ) ;
#162316=ORIENTED_EDGE ( 'NONE', *, *, #58498, .F. ) ;
#162377=CIRCLE ( 'NONE', #74907, 0.09999999999999939493 ) ;
#162392=DIRECTION ( 'NONE',  ( 0.000000000000000000, 1.000000000000000000, 0.000000000000000000 ) ) ;
#162410=FACE_OUTER_BOUND ( 'NONE', #173415, .T. ) ;
#162415=VERTEX_POINT ( 'NONE', #8035 ) ;
#162578=AXIS2_PLACEMENT_3D ( 'NONE', #124014, #43187, #243938 ) ;
#162616=ORIENTED_EDGE ( 'NONE', *, *, #99045, .T. ) ;
#162627=CARTESIAN_POINT ( 'NONE',  ( -18.79999999999999716, 7.986648289447971116, 1.311673547813416718 ) ) ;
#162656=LINE ( 'NONE', #199215, #40088 ) ;
#162677=ORIENTED_EDGE ( 'NONE', *, *, #137878, .F. ) ;
#162692=ORIENTED_EDGE ( 'NONE', *, *, #152792, .F. ) ;
#162782=DIRECTION ( 'NONE',  ( 1.000000000000000000, -0.000000000000000000, -0.000000000000000000 ) ) ;
#162801=ADVANCED_FACE ( 'NONE', ( #46814 ), #187238, .T. ) ;
#162811=VERTEX_POINT ( 'NONE', #166821 ) ;
#162920=CARTESIAN_POINT ( 'NONE',  ( -22.94999999999999929, 0.000000000000000000, 0.000000000000000000 ) ) ;
#162949=CIRCLE ( 'NONE', #25562, 0.09999999999999990841 ) ;
#162963=DIRECTION ( 'NONE',  ( -1.000000000000000000, 0.000000000000000000, 0.000000000000000000 ) ) ;
#162985=AXIS2_PLACEMENT_3D ( 'NONE', #166494, #244697, #226407 ) ;
#163001=ADVANCED_FACE ( 'NONE', ( #194070 ), #109354, .T. ) ;
#163012=ORIENTED_EDGE ( 'NONE', *, *, #13795, .F. ) ;
#163015=CYLINDRICAL_SURFACE ( 'NONE', #69407, 0.09999999999999939493 ) ;
#163023=PLANE ( 'NONE',  #180333 ) ;
#163055=CIRCLE ( 'NONE', #50585, 0.09999999999999990841 ) ;
#163106=CARTESIAN_POINT ( 'NONE',  ( -18.59999999999999787, -10.64999999999999325, 31.59999999999999787 ) ) ;
#163162=CARTESIAN_POINT ( 'NONE',  ( 20.90000000000000213, 1.885425182446133885, -11.49641995933507843 ) ) ;
#163216=FACE_OUTER_BOUND ( 'NONE', #49076, .T. ) ;
#163225=ADVANCED_FACE ( 'NONE', ( #63505 ), #64795, .T. ) ;
#163279=DIRECTION ( 'NONE',  ( -0.000000000000000000, 1.000000000000000000, -0.000000000000000000 ) ) ;
#163288=DIRECTION ( 'NONE',  ( 0.000000000000000000, 0.9910465087640865089, -0.1335171055202867274 ) ) ;
#163302=LINE ( 'NONE', #207572, #14628 ) ;
#163334=AXIS2_PLACEMENT_3D ( 'NONE', #104256, #22196, #183815 ) ;
#163347=EDGE_CURVE ( 'NONE', #150529, #29621, #209441, .T. ) ;
#163412=CARTESIAN_POINT ( 'NONE',  ( 18.69999999999999929, 9.511171963237318394, 1.617965922123942191 ) ) ;
#163435=ORIENTED_EDGE ( 'NONE', *, *, #241156, .F. ) ;
#163444=CARTESIAN_POINT ( 'NONE',  ( 18.59999999999999787, -10.64999999999999325, 32.89999999999999858 ) ) ;
#163445=VERTEX_POINT ( 'NONE', #76334 ) ;
#163453=CARTESIAN_POINT ( 'NONE',  ( -18.79999999999999716, 1.885425182446133885, -11.49641995933507843 ) ) ;
#163461=ORIENTED_EDGE ( 'NONE', *, *, #200132, .F. ) ;
#163469=AXIS2_PLACEMENT_3D ( 'NONE', #188530, #11186, #26923 ) ;
#163472=CARTESIAN_POINT ( 'NONE',  ( -18.59999999999999787, 11.75000000000000000, 30.00000000000000000 ) ) ;
#163484=VERTEX_POINT ( 'NONE', #219708 ) ;
#163495=CIRCLE ( 'NONE', #67631, 0.1999999999999987899 ) ;
#163507=VECTOR ( 'NONE', #214489, 1000.000000000000227 ) ;
#163509=AXIS2_PLACEMENT_3D ( 'NONE', #79364, #155107, #257969 ) ;
#163570=DIRECTION ( 'NONE',  ( 1.000000000000000000, 0.000000000000000000, 0.000000000000000000 ) ) ;
#163598=CARTESIAN_POINT ( 'NONE',  ( -18.79999999999999716, -1.467286812112899463, 32.89999999999999858 ) ) ;
#163601=VECTOR ( 'NONE', #100427, 1000.000000000000000 ) ;
#163646=EDGE_LOOP ( 'NONE', ( #197011, #169092, #230193, #50652 ) ) ;
#163656=VERTEX_POINT ( 'NONE', #41110 ) ;
#163661=AXIS2_PLACEMENT_3D ( 'NONE', #53282, #187674, #208519 ) ;
#163669=CARTESIAN_POINT ( 'NONE',  ( 18.69999999999999929, 6.841561409100513025, 9.675512259591560138 ) ) ;
#163683=DIRECTION ( 'NONE',  ( 0.000000000000000000, 1.000000000000000000, 0.000000000000000000 ) ) ;
#163701=ORIENTED_EDGE ( 'NONE', *, *, #96461, .T. ) ;
#163747=CYLINDRICAL_SURFACE ( 'NONE', #140870, 0.1000000000000000472 ) ;
#163777=VERTEX_POINT ( 'NONE', #171358 ) ;
#163817=ORIENTED_EDGE ( 'NONE', *, *, #135523, .F. ) ;
#163868=ORIENTED_EDGE ( 'NONE', *, *, #46105, .F. ) ;
#163886=DIRECTION ( 'NONE',  ( 0.000000000000000000, 1.000000000000000000, 0.000000000000000000 ) ) ;
#163945=ORIENTED_EDGE ( 'NONE', *, *, #233241, .F. ) ;
#163949=CIRCLE ( 'NONE', #134871, 0.09999999999999939493 ) ;
#163954=DIRECTION ( 'NONE',  ( -0.000000000000000000, 0.000000000000000000, 1.000000000000000000 ) ) ;
#163966=DIRECTION ( 'NONE',  ( 0.000000000000000000, 0.1335171055202901413, 0.9910465087640860649 ) ) ;
#163967=CIRCLE ( 'NONE', #159328, 0.09999999999999939493 ) ;
#163992=VERTEX_POINT ( 'NONE', #180299 ) ;
#164090=CIRCLE ( 'NONE', #5833, 0.09999999999999993616 ) ;
#164220=AXIS2_PLACEMENT_3D ( 'NONE', #94002, #118734, #174894 ) ;
#164252=DIRECTION ( 'NONE',  ( 0.000000000000000000, 0.9856811345164800953, 0.1686199900910462790 ) ) ;
#164253=AXIS2_PLACEMENT_3D ( 'NONE', #179704, #16789, #200533 ) ;
#164262=EDGE_CURVE ( 'NONE', #8702, #163445, #24467, .T. ) ;
#164325=AXIS2_PLACEMENT_3D ( 'NONE', #256657, #78066, #134188 ) ;
#164327=CIRCLE ( 'NONE', #93383, 0.1999999999999987899 ) ;
#164330=DIRECTION ( 'NONE',  ( 0.000000000000000000, -0.9910465087640861759, -0.1335171055202901691 ) ) ;
#164334=EDGE_CURVE ( 'NONE', #144252, #119824, #254552, .T. ) ;
#164418=CIRCLE ( 'NONE', #243505, 3.970710678118653636 ) ;
#164437=CARTESIAN_POINT ( 'NONE',  ( -21.00000000000000000, 0.000000000000000000, 0.000000000000000000 ) ) ;
#164476=ADVANCED_FACE ( 'NONE', ( #231639 ), #33872, .T. ) ;
#164488=CIRCLE ( 'NONE', #110297, 0.1000000000000028644 ) ;
#164491=EDGE_CURVE ( 'NONE', #118720, #86236, #154659, .T. ) ;
#164523=CARTESIAN_POINT ( 'NONE',  ( -21.00000000000000000, 6.726092018229619995, 9.512212474619552438 ) ) ;
#164609=ORIENTED_EDGE ( 'NONE', *, *, #79475, .T. ) ;
#164620=DIRECTION ( 'NONE',  ( 8.775271659896538527E-15, -0.1686199900910279881, 0.9856811345164833149 ) ) ;
#164655=VERTEX_POINT ( 'NONE', #240610 ) ;
#164656=DIRECTION ( 'NONE',  ( 0.000000000000000000, -1.000000000000000000, 0.000000000000000000 ) ) ;
#164677=ORIENTED_EDGE ( 'NONE', *, *, #91517, .F. ) ;
#164691=DIRECTION ( 'NONE',  ( -1.000000000000000000, -0.000000000000000000, -0.000000000000000000 ) ) ;
#164699=CARTESIAN_POINT ( 'NONE',  ( 20.00000000000000711, 4.645987002755569861, 21.91686199900910736 ) ) ;
#164741=DIRECTION ( 'NONE',  ( 0.000000000000000000, 0.9910465087640866200, -0.1335171055202867274 ) ) ;
#164776=DIRECTION ( 'NONE',  ( 0.000000000000000000, 0.000000000000000000, -1.000000000000000000 ) ) ;
#164781=ORIENTED_EDGE ( 'NONE', *, *, #239815, .T. ) ;
#164828=AXIS2_PLACEMENT_3D ( 'NONE', #76102, #159514, #139912 ) ;
#164840=ORIENTED_EDGE ( 'NONE', *, *, #145094, .F. ) ;
#164856=CARTESIAN_POINT ( 'NONE',  ( -18.59999999999999787, -9.749999999999994671, 30.09999999999999076 ) ) ;
#164996=DIRECTION ( 'NONE',  ( -1.000000000000000000, 0.000000000000000000, 0.000000000000000000 ) ) ;
#165000=ORIENTED_EDGE ( 'NONE', *, *, #52789, .F. ) ;
#165049=EDGE_LOOP ( 'NONE', ( #69426, #105323, #215516, #149210 ) ) ;
#165106=AXIS2_PLACEMENT_3D ( 'NONE', #188531, #205517, #67301 ) ;
#165111=EDGE_CURVE ( 'NONE', #84718, #233154, #59267, .T. ) ;
#165132=LINE ( 'NONE', #47731, #42752 ) ;
#165194=AXIS2_PLACEMENT_3D ( 'NONE', #226901, #185213, #6570 ) ;
#165210=AXIS2_PLACEMENT_3D ( 'NONE', #50164, #129715, #159561 ) ;
#165214=EDGE_CURVE ( 'NONE', #217842, #47981, #97752, .T. ) ;
#165224=ORIENTED_EDGE ( 'NONE', *, *, #256305, .T. ) ;
#165226=LINE ( 'NONE', #166543, #230372 ) ;
#165245=CARTESIAN_POINT ( 'NONE',  ( -21.00000000000000000, -11.65000000000000036, 0.000000000000000000 ) ) ;
#165275=CARTESIAN_POINT ( 'NONE',  ( -18.69999999999999929, -2.462484827400499565, -15.77971343137458682 ) ) ;
#165302=ADVANCED_FACE ( 'NONE', ( #174965 ), #152816, .T. ) ;
#165336=DIRECTION ( 'NONE',  ( -1.000000000000000000, -0.000000000000000000, -0.000000000000000000 ) ) ;
#165414=FACE_OUTER_BOUND ( 'NONE', #184329, .T. ) ;
#165427=CYLINDRICAL_SURFACE ( 'NONE', #36448, 0.09999999999999990841 ) ;
#165458=EDGE_CURVE ( 'NONE', #199798, #132306, #121871, .T. ) ;
#165471=EDGE_CURVE ( 'NONE', #239767, #160025, #226059, .T. ) ;
#165473=CARTESIAN_POINT ( 'NONE',  ( 18.79999999999999716, 1.250000000000000000, 0.000000000000000000 ) ) ;
#165512=CIRCLE ( 'NONE', #169821, 2.600000000000001421 ) ;
#165551=ORIENTED_EDGE ( 'NONE', *, *, #146012, .F. ) ;
#165553=AXIS2_PLACEMENT_3D ( 'NONE', #96968, #38337, #1745 ) ;
#165562=AXIS2_PLACEMENT_3D ( 'NONE', #205700, #220480, #21010 ) ;
#165588=CARTESIAN_POINT ( 'NONE',  ( 18.79999999999999716, 1.885425182446133885, -11.49641995933507843 ) ) ;
#165590=ORIENTED_EDGE ( 'NONE', *, *, #99118, .F. ) ;
#165591=AXIS2_PLACEMENT_3D ( 'NONE', #235387, #159723, #20216 ) ;
#165662=ORIENTED_EDGE ( 'NONE', *, *, #138596, .T. ) ;
#165701=DIRECTION ( 'NONE',  ( 0.000000000000000000, -1.000000000000000000, 0.000000000000000000 ) ) ;
#165844=ORIENTED_EDGE ( 'NONE', *, *, #117955, .F. ) ;
#165866=AXIS2_PLACEMENT_3D ( 'NONE', #79788, #117658, #95524 ) ;
#165870=DIRECTION ( 'NONE',  ( -1.000000000000000000, 0.000000000000000000, -0.000000000000000000 ) ) ;
#165900=CARTESIAN_POINT ( 'NONE',  ( -20.10000000000000142, 5.572697453181475247, 16.49970471148372297 ) ) ;
#165912=EDGE_CURVE ( 'NONE', #70728, #76759, #52726, .T. ) ;
#165931=ORIENTED_EDGE ( 'NONE', *, *, #71599, .F. ) ;
#165993=EDGE_CURVE ( 'NONE', #212664, #5080, #96960, .T. ) ;
#165997=DIRECTION ( 'NONE',  ( 1.000000000000000000, 0.000000000000000000, 0.000000000000000000 ) ) ;
#166006=CIRCLE ( 'NONE', #53554, 0.09999999999999939493 ) ;
#166010=DIRECTION ( 'NONE',  ( 0.000000000000000000, 0.000000000000000000, 1.000000000000000000 ) ) ;
#166023=VECTOR ( 'NONE', #124670, 1000.000000000000000 ) ;
#166038=EDGE_LOOP ( 'NONE', ( #216505, #80245, #26281, #36630 ) ) ;
#166060=DIRECTION ( 'NONE',  ( 1.000000000000000000, -0.000000000000000000, 0.000000000000000000 ) ) ;
#166061=ADVANCED_FACE ( 'NONE', ( #79974 ), #238750, .T. ) ;
#166069=ORIENTED_EDGE ( 'NONE', *, *, #165214, .T. ) ;
#166082=CIRCLE ( 'NONE', #182830, 0.1000000000000028644 ) ;
#166158=CARTESIAN_POINT ( 'NONE',  ( -21.10000000000000142, 0.000000000000000000, -4.000000000000000000 ) ) ;
#166160=FACE_OUTER_BOUND ( 'NONE', #199294, .T. ) ;
#166243=VERTEX_POINT ( 'NONE', #26465 ) ;
#166271=DIRECTION ( 'NONE',  ( 0.000000000000000000, -0.5773469543544729188, -0.8164989248600478255 ) ) ;
#166300=CARTESIAN_POINT ( 'NONE',  ( 18.69999999999999929, -8.150000000000007461, 10.52591260281975138 ) ) ;
#166303=ORIENTED_EDGE ( 'NONE', *, *, #158884, .F. ) ;
#166320=CARTESIAN_POINT ( 'NONE',  ( 6.099999999999987210, -11.75000000000000000, -15.00000000000001243 ) ) ;
#166399=DIRECTION ( 'NONE',  ( 0.000000000000000000, 0.000000000000000000, 1.000000000000000000 ) ) ;
#166410=PLANE ( 'NONE',  #35649 ) ;
#166443=CARTESIAN_POINT ( 'NONE',  ( -18.79999999999999716, 7.900000000000000355, 1.300000000000000044 ) ) ;
#166457=DIRECTION ( 'NONE',  ( 0.000000000000000000, 0.000000000000000000, -1.000000000000000000 ) ) ;
#166466=DIRECTION ( 'NONE',  ( 0.000000000000000000, -0.8741572761215371523, 0.4856429311786332748 ) ) ;
#166494=CARTESIAN_POINT ( 'NONE',  ( -22.94999999999999929, 3.461118860469513336, 28.84309995045515507 ) ) ;
#166517=AXIS2_PLACEMENT_3D ( 'NONE', #185433, #102007, #66774 ) ;
#166542=VECTOR ( 'NONE', #79154, 1000.000000000000000 ) ;
#166543=CARTESIAN_POINT ( 'NONE',  ( -18.69999999999999929, 7.799999999999999822, -15.00000000000000000 ) ) ;
#166591=DIRECTION ( 'NONE',  ( 0.000000000000000000, 0.000000000000000000, 1.000000000000000000 ) ) ;
#166593=ORIENTED_EDGE ( 'NONE', *, *, #227709, .F. ) ;
#166606=CIRCLE ( 'NONE', #198778, 0.09999999999999939493 ) ;
#166630=ORIENTED_EDGE ( 'NONE', *, *, #17407, .F. ) ;
#166645=ORIENTED_EDGE ( 'NONE', *, *, #233704, .T. ) ;
#166651=LINE ( 'NONE', #183619, #182469 ) ;
#166671=EDGE_LOOP ( 'NONE', ( #188735, #97781, #27839, #252852 ) ) ;
#166673=ADVANCED_FACE ( 'NONE', ( #125254 ), #106955, .T. ) ;
#166686=SURFACE_STYLE_FILL_AREA ( #72716 ) ;
#166702=EDGE_LOOP ( 'NONE', ( #61145, #212906, #201255, #1439 ) ) ;
#166706=VERTEX_POINT ( 'NONE', #123978 ) ;
#166745=EDGE_CURVE ( 'NONE', #211171, #48243, #67838, .T. ) ;
#166752=AXIS2_PLACEMENT_3D ( 'NONE', #115633, #213440, #116915 ) ;
#166757=LINE ( 'NONE', #54133, #180873 ) ;
#166783=FACE_OUTER_BOUND ( 'NONE', #95655, .T. ) ;
#166805=VERTEX_POINT ( 'NONE', #55959 ) ;
#166819=ADVANCED_FACE ( 'NONE', ( #54695 ), #242638, .T. ) ;
#166821=CARTESIAN_POINT ( 'NONE',  ( -18.79999999999999716, 4.513204987021263825, 22.00000000000000355 ) ) ;
#166857=CIRCLE ( 'NONE', #25188, 0.1000000000000000749 ) ;
#166883=VERTEX_POINT ( 'NONE', #74299 ) ;
#166914=CARTESIAN_POINT ( 'NONE',  ( -11.60000000000000320, -8.350000000000004974, 19.04142135623731491 ) ) ;
#166926=VERTEX_POINT ( 'NONE', #175959 ) ;
#166934=EDGE_CURVE ( 'NONE', #203964, #6496, #230163, .T. ) ;
#166966=ORIENTED_EDGE ( 'NONE', *, *, #210423, .T. ) ;
#167038=CARTESIAN_POINT ( 'NONE',  ( -18.79999999999999716, 7.900000000000000355, -1.212568896937008089 ) ) ;
#167045=AXIS2_PLACEMENT_3D ( 'NONE', #198637, #99510, #60403 ) ;
#167113=FACE_OUTER_BOUND ( 'NONE', #62738, .T. ) ;
#167163=VECTOR ( 'NONE', #87275, 1000.000000000000000 ) ;
#167178=CARTESIAN_POINT ( 'NONE',  ( -19.99999999999999645, 4.645987002755569861, 21.91686199900910736 ) ) ;
#167196=DIRECTION ( 'NONE',  ( 1.476360405086644309E-16, 1.000000000000000000, 1.445602896647339410E-16 ) ) ;
#167234=DIRECTION ( 'NONE',  ( 0.000000000000000000, 0.000000000000000000, -1.000000000000000000 ) ) ;
#167242=EDGE_LOOP ( 'NONE', ( #59974, #203623, #71415 ) ) ;
#167257=EDGE_CURVE ( 'NONE', #62787, #57087, #37413, .T. ) ;
#167267=ORIENTED_EDGE ( 'NONE', *, *, #133328, .F. ) ;
#167269=CARTESIAN_POINT ( 'NONE',  ( 21.00000000000000000, 5.021051876504148371E-16, 4.100000000000000533 ) ) ;
#167281=EDGE_CURVE ( 'NONE', #157564, #59508, #30948, .T. ) ;
#167314=AXIS2_PLACEMENT_3D ( 'NONE', #206817, #149434, #50289 ) ;
#167340=VECTOR ( 'NONE', #66014, 1000.000000000000000 ) ;
#167426=EDGE_LOOP ( 'NONE', ( #34307, #85353, #66639, #168537 ) ) ;
#167452=ORIENTED_EDGE ( 'NONE', *, *, #67992, .T. ) ;
#167459=CARTESIAN_POINT ( 'NONE',  ( -18.59999999999999787, -10.64999999999999325, 31.50000000000000000 ) ) ;
#167492=EDGE_LOOP ( 'NONE', ( #223754, #182963, #87584, #80368 ) ) ;
#167495=ORIENTED_EDGE ( 'NONE', *, *, #10904, .F. ) ;
#167502=CARTESIAN_POINT ( 'NONE',  ( -5.900000000000002132, -11.75000000000000000, 13.90000000000000213 ) ) ;
#167621=VECTOR ( 'NONE', #119694, 1000.000000000000000 ) ;
#167718=CARTESIAN_POINT ( 'NONE',  ( -20.90000000000000213, 1.410778198689825347, -7.973296578895943121 ) ) ;
#167731=DIRECTION ( 'NONE',  ( 1.000000000000000000, 0.000000000000000000, 0.000000000000000000 ) ) ;
#167782=ORIENTED_EDGE ( 'NONE', *, *, #16767, .F. ) ;
#167827=EDGE_CURVE ( 'NONE', #188929, #52766, #159534, .T. ) ;
#167847=VERTEX_POINT ( 'NONE', #109566 ) ;
#167853=CIRCLE ( 'NONE', #88694, 0.09999999999999939493 ) ;
#167889=FACE_OUTER_BOUND ( 'NONE', #42911, .T. ) ;
#167979=FACE_OUTER_BOUND ( 'NONE', #221366, .T. ) ;
#168001=AXIS2_PLACEMENT_3D ( 'NONE', #127995, #206243, #66737 ) ;
#168018=ORIENTED_EDGE ( 'NONE', *, *, #20406, .T. ) ;
#168022=CARTESIAN_POINT ( 'NONE',  ( 20.90000000000000213, 11.49641995933507843, -1.885425182446133885 ) ) ;
#168025=AXIS2_PLACEMENT_3D ( 'NONE', #232809, #213205, #157123 ) ;
#168032=VERTEX_POINT ( 'NONE', #80703 ) ;
#168078=DIRECTION ( 'NONE',  ( 0.000000000000000000, -0.9856811345164829818, -0.1686199900910294314 ) ) ;
#168083=VECTOR ( 'NONE', #53368, 1000.000000000000000 ) ;
#168138=CARTESIAN_POINT ( 'NONE',  ( -21.00000000000000000, -11.65000000000000036, 11.89999999999999858 ) ) ;
#168156=CARTESIAN_POINT ( 'NONE',  ( -18.69999999999999929, 3.362550747017870378, 28.82623795144604983 ) ) ;
#168189=TOROIDAL_SURFACE ( 'NONE', #168001, 4.100000000000000533, 0.1000000000000000056 ) ;
#168198=DIRECTION ( 'NONE',  ( 0.000000000000000000, 0.000000000000000000, 1.000000000000000000 ) ) ;
#168210=DIRECTION ( 'NONE',  ( 0.000000000000000000, 0.1335171055202867274, -0.9910465087640866200 ) ) ;
#168222=EDGE_CURVE ( 'NONE', #38945, #204755, #186255, .T. ) ;
#168240=CARTESIAN_POINT ( 'NONE',  ( 0.8999999999999993561, -11.65000000000000036, 28.60000000000000142 ) ) ;
#168244=VERTEX_POINT ( 'NONE', #203236 ) ;
#168250=ORIENTED_EDGE ( 'NONE', *, *, #217303, .T. ) ;
#168265=ORIENTED_EDGE ( 'NONE', *, *, #252186, .F. ) ;
#168268=CARTESIAN_POINT ( 'NONE',  ( 19.90000000000000568, 5.488301202077012775, 16.50000000000000000 ) ) ;
#168275=VECTOR ( 'NONE', #141403, 1000.000000000000000 ) ;
#168302=DIRECTION ( 'NONE',  ( 1.000000000000000000, -0.000000000000000000, -0.000000000000000000 ) ) ;
#168326=EDGE_CURVE ( 'NONE', #16903, #87211, #85820, .T. ) ;
#168416=ORIENTED_EDGE ( 'NONE', *, *, #32335, .F. ) ;
#168446=DIRECTION ( 'NONE',  ( 0.000000000000000000, 0.000000000000000000, -1.000000000000000000 ) ) ;
#168497=EDGE_LOOP ( 'NONE', ( #10247, #224123, #228927, #10387 ) ) ;
#168516=EDGE_LOOP ( 'NONE', ( #54051, #14322, #87047, #162316 ) ) ;
#168528=VERTEX_POINT ( 'NONE', #182091 ) ;
#168537=ORIENTED_EDGE ( 'NONE', *, *, #34547, .F. ) ;
#168575=DIRECTION ( 'NONE',  ( 0.000000000000000000, 1.000000000000000000, 0.000000000000000000 ) ) ;
#168654=CARTESIAN_POINT ( 'NONE',  ( 18.69999999999999929, 0.000000000000000000, 0.000000000000000000 ) ) ;
#168684=CYLINDRICAL_SURFACE ( 'NONE', #86103, 0.09999999999999939493 ) ;
#168715=DIRECTION ( 'NONE',  ( -0.000000000000000000, -1.000000000000000000, -0.000000000000000000 ) ) ;
#168739=AXIS2_PLACEMENT_3D ( 'NONE', #86268, #110998, #210114 ) ;
#168782=AXIS2_PLACEMENT_3D ( 'NONE', #108456, #105858, #107160 ) ;
#168788=AXIS2_PLACEMENT_3D ( 'NONE', #208875, #30257, #74551 ) ;
#168789=AXIS2_PLACEMENT_3D ( 'NONE', #30081, #243955, #109572 ) ;
#168795=FACE_OUTER_BOUND ( 'NONE', #117388, .T. ) ;
#168802=LINE ( 'NONE', #248287, #111448 ) ;
#168806=VECTOR ( 'NONE', #92445, 1000.000000000000000 ) ;
#168845=CARTESIAN_POINT ( 'NONE',  ( 13.40000000000000036, -8.250000000000003553, 15.00000000000000355 ) ) ;
#168900=ORIENTED_EDGE ( 'NONE', *, *, #66088, .T. ) ;
#168926=FACE_OUTER_BOUND ( 'NONE', #234000, .T. ) ;
#168943=EDGE_CURVE ( 'NONE', #39190, #253747, #151148, .T. ) ;
#169022=VERTEX_POINT ( 'NONE', #92476 ) ;
#169075=ORIENTED_EDGE ( 'NONE', *, *, #101136, .F. ) ;
#169092=ORIENTED_EDGE ( 'NONE', *, *, #193254, .T. ) ;
#169098=CARTESIAN_POINT ( 'NONE',  ( 18.79999999999999716, -1.300000000000000044, -7.900000000000000355 ) ) ;
#169146=CIRCLE ( 'NONE', #10722, 0.2000000000000005107 ) ;
#169174=ORIENTED_EDGE ( 'NONE', *, *, #211626, .T. ) ;
#169176=DIRECTION ( 'NONE',  ( -0.000000000000000000, 0.1618390714546030229, 0.9868171638914231547 ) ) ;
#169188=DIRECTION ( 'NONE',  ( -1.000000000000000000, 0.000000000000000000, 0.000000000000000000 ) ) ;
#169191=EDGE_LOOP ( 'NONE', ( #72264, #132288, #96835, #232573 ) ) ;
#169202=EDGE_CURVE ( 'NONE', #242362, #232547, #9657, .T. ) ;
#169254=CARTESIAN_POINT ( 'NONE',  ( -37.88850191057539973, -10.72142460728770352, 6.051435706882140053 ) ) ;
#169297=VERTEX_POINT ( 'NONE', #4904 ) ;
#169301=CARTESIAN_POINT ( 'NONE',  ( 18.59999999999999787, -9.849999999999994316, 30.09999999999999787 ) ) ;
#169360=CYLINDRICAL_SURFACE ( 'NONE', #234847, 0.09999999999999939493 ) ;
#169369=EDGE_LOOP ( 'NONE', ( #26429, #174708, #45275, #239246 ) ) ;
#169430=CARTESIAN_POINT ( 'NONE',  ( -20.90000000000000213, -11.65000000000000036, 11.89999999999999858 ) ) ;
#169438=CARTESIAN_POINT ( 'NONE',  ( 19.90000000000000568, 1.350000000000000089, 16.60000000000000142 ) ) ;
#169467=CARTESIAN_POINT ( 'NONE',  ( -18.69999999999999929, -10.64999999999999325, 31.59999999999999787 ) ) ;
#169479=VECTOR ( 'NONE', #143979, 1000.000000000000000 ) ;
#169513=ORIENTED_EDGE ( 'NONE', *, *, #226241, .T. ) ;
#169577=EDGE_CURVE ( 'NONE', #122251, #181466, #155628, .T. ) ;
#169606=VERTEX_POINT ( 'NONE', #106271 ) ;
#169652=DIRECTION ( 'NONE',  ( 0.000000000000000000, -1.000000000000000000, 0.000000000000000000 ) ) ;
#169705=VERTEX_POINT ( 'NONE', #241949 ) ;
#169779=ORIENTED_EDGE ( 'NONE', *, *, #187515, .F. ) ;
#169814=AXIS2_PLACEMENT_3D ( 'NONE', #253967, #217405, #101268 ) ;
#169815=VERTEX_POINT ( 'NONE', #68464 ) ;
#169821=AXIS2_PLACEMENT_3D ( 'NONE', #195726, #37931, #151454 ) ;
#169876=DIRECTION ( 'NONE',  ( 0.000000000000000000, 0.000000000000000000, 1.000000000000000000 ) ) ;
#169879=TOROIDAL_SURFACE ( 'NONE', #44934, 0.2000000000000000111, 0.1000000000000000056 ) ;
#169908=CARTESIAN_POINT ( 'NONE',  ( -18.60000000000000142, -8.350000000000004974, 33.00000000000000000 ) ) ;
#169953=FACE_OUTER_BOUND ( 'NONE', #57829, .T. ) ;
#169958=FACE_OUTER_BOUND ( 'NONE', #232968, .T. ) ;
#169969=ORIENTED_EDGE ( 'NONE', *, *, #64589, .T. ) ;
#169978=AXIS2_PLACEMENT_3D ( 'NONE', #138581, #218132, #79892 ) ;
#170052=VECTOR ( 'NONE', #10758, 1000.000000000000000 ) ;
#170066=EDGE_CURVE ( 'NONE', #60954, #119804, #59125, .T. ) ;
#170067=AXIS2_PLACEMENT_3D ( 'NONE', #201860, #218839, #40249 ) ;
#170083=ADVANCED_FACE ( 'NONE', ( #220800 ), #26472, .T. ) ;
#170085=DIRECTION ( 'NONE',  ( 1.000000000000000000, 0.000000000000000000, 0.000000000000000000 ) ) ;
#170095=FACE_OUTER_BOUND ( 'NONE', #116640, .T. ) ;
#170120=LINE ( 'NONE', #245761, #94427 ) ;
#170178=PLANE ( 'NONE',  #60966 ) ;
#170206=EDGE_LOOP ( 'NONE', ( #82449, #142765, #27313, #240647 ) ) ;
#170217=FACE_BOUND ( 'NONE', #106382, .T. ) ;
#170326=LINE ( 'NONE', #252359, #245448 ) ;
#170378=FACE_OUTER_BOUND ( 'NONE', #79700, .T. ) ;
#170387=EDGE_CURVE ( 'NONE', #163445, #206620, #34197, .T. ) ;
#170394=EDGE_LOOP ( 'NONE', ( #63944, #9309, #86333, #252659 ) ) ;
#170432=CARTESIAN_POINT ( 'NONE',  ( 21.10000000000000142, -11.75000000000000000, 12.09999999999999609 ) ) ;
#170444=DIRECTION ( 'NONE',  ( 0.000000000000000000, 1.000000000000000000, -0.000000000000000000 ) ) ;
#170491=DIRECTION ( 'NONE',  ( 1.000000000000000000, -0.000000000000000000, 0.000000000000000000 ) ) ;
#170580=LINE ( 'NONE', #132688, #198787 ) ;
#170649=CARTESIAN_POINT ( 'NONE',  ( 5.999999999999997335, -11.34999999999999964, 13.90000000000000213 ) ) ;
#170674=ORIENTED_EDGE ( 'NONE', *, *, #108785, .T. ) ;
#170772=CARTESIAN_POINT ( 'NONE',  ( 18.79999999999999716, -1.212568896937008089, -8.000000000000000000 ) ) ;
#170776=DIRECTION ( 'NONE',  ( -1.000000000000000000, 0.000000000000000000, 0.000000000000000000 ) ) ;
#170802=VECTOR ( 'NONE', #215389, 1000.000000000000000 ) ;
#170830=ORIENTED_EDGE ( 'NONE', *, *, #98558, .F. ) ;
#170835=LINE ( 'NONE', #71700, #119166 ) ;
#170851=ORIENTED_EDGE ( 'NONE', *, *, #75148, .F. ) ;
#170854=VECTOR ( 'NONE', #248840, 1000.000000000000000 ) ;
#170892=ORIENTED_EDGE ( 'NONE', *, *, #22619, .F. ) ;
#170900=AXIS2_PLACEMENT_3D ( 'NONE', #250372, #47011, #190421 ) ;
#170906=CARTESIAN_POINT ( 'NONE',  ( 18.79999999999999716, -10.84999999999999076, 32.89999999999999858 ) ) ;
#170947=DIRECTION ( 'NONE',  ( -2.605671645643297230E-15, 0.9910465087640865089, 0.1335171055202867274 ) ) ;
#170949=EDGE_LOOP ( 'NONE', ( #42232, #138932, #57474, #34783 ) ) ;
#171080=VECTOR ( 'NONE', #57056, 1000.000000000000000 ) ;
#171081=CARTESIAN_POINT ( 'NONE',  ( -0.8999999999999993561, -9.650000000000003908, 28.60000000000000142 ) ) ;
#171083=AXIS2_PLACEMENT_3D ( 'NONE', #56764, #257506, #35970 ) ;
#171091=ORIENTED_EDGE ( 'NONE', *, *, #18388, .F. ) ;
#171171=ORIENTED_EDGE ( 'NONE', *, *, #30944, .F. ) ;
#171175=EDGE_CURVE ( 'NONE', #105944, #48863, #218840, .T. ) ;
#171184=AXIS2_PLACEMENT_3D ( 'NONE', #85671, #201801, #23199 ) ;
#171206=DIRECTION ( 'NONE',  ( 1.000000000000000000, -0.000000000000000000, -0.000000000000000000 ) ) ;
#171211=LINE ( 'NONE', #194608, #76726 ) ;
#171242=CARTESIAN_POINT ( 'NONE',  ( 18.59999999999999787, -11.65000000000000036, 30.00000000000000000 ) ) ;
#171310=EDGE_CURVE ( 'NONE', #208877, #141175, #202566, .T. ) ;
#171323=VERTEX_POINT ( 'NONE', #112471 ) ;
#171353=ORIENTED_EDGE ( 'NONE', *, *, #31730, .T. ) ;
#171358=CARTESIAN_POINT ( 'NONE',  ( -20.90000000000000213, 11.50977166988710820, 1.786320531569725478 ) ) ;
#171392=DIRECTION ( 'NONE',  ( 0.000000000000000000, 0.000000000000000000, 1.000000000000000000 ) ) ;
#171414=VERTEX_POINT ( 'NONE', #251963 ) ;
#171542=DIRECTION ( 'NONE',  ( 0.000000000000000000, 0.000000000000000000, -1.000000000000000000 ) ) ;
#171556=CYLINDRICAL_SURFACE ( 'NONE', #109320, 0.09999999999999939493 ) ;
#171566=VERTEX_POINT ( 'NONE', #135852 ) ;
#171575=CARTESIAN_POINT ( 'NONE',  ( 11.60000000000000142, -12.24999999999999822, 15.00000000000000355 ) ) ;
#171627=CARTESIAN_POINT ( 'NONE',  ( -20.90000000000000213, 11.50977166988710820, -1.786320531569725478 ) ) ;
#171633=VERTEX_POINT ( 'NONE', #121479 ) ;
#171680=CARTESIAN_POINT ( 'NONE',  ( 20.10000000000000853, 3.362550747017865493, 28.82623795144604983 ) ) ;
#171697=VERTEX_POINT ( 'NONE', #65318 ) ;
#171723=DIRECTION ( 'NONE',  ( -1.000000000000000000, 0.000000000000000000, 0.000000000000000000 ) ) ;
#171730=AXIS2_PLACEMENT_3D ( 'NONE', #200098, #120581, #21478 ) ;
#171755=EDGE_CURVE ( 'NONE', #32241, #149370, #148312, .T. ) ;
#171761=ADVANCED_FACE ( 'NONE', ( #49613 ), #207423, .T. ) ;
#171769=EDGE_CURVE ( 'NONE', #239767, #172933, #87443, .T. ) ;
#171771=ORIENTED_EDGE ( 'NONE', *, *, #105931, .F. ) ;
#171785=DIRECTION ( 'NONE',  ( -1.000000000000000000, 0.000000000000000000, 0.000000000000000000 ) ) ;
#171824=DIRECTION ( 'NONE',  ( 1.000000000000000000, 0.000000000000000000, -0.000000000000000000 ) ) ;
#171825=FILL_AREA_STYLE_COLOUR ( '', #68909 ) ;
#171856=ORIENTED_EDGE ( 'NONE', *, *, #152153, .T. ) ;
#171861=FACE_OUTER_BOUND ( 'NONE', #101443, .T. ) ;
#171885=DIRECTION ( 'NONE',  ( 0.000000000000000000, -1.000000000000000000, 0.000000000000000000 ) ) ;
#171946=VERTEX_POINT ( 'NONE', #76869 ) ;
#171952=AXIS2_PLACEMENT_3D ( 'NONE', #137291, #100705, #198554 ) ;
#171957=ADVANCED_FACE ( 'NONE', ( #93871 ), #106790, .T. ) ;
#171966=EDGE_CURVE ( 'NONE', #152492, #39190, #173500, .T. ) ;
#172050=LINE ( 'NONE', #129042, #139672 ) ;
#172070=CIRCLE ( 'NONE', #67794, 0.09999999999999939493 ) ;
#172088=AXIS2_PLACEMENT_3D ( 'NONE', #92527, #73017, #152551 ) ;
#172094=DIRECTION ( 'NONE',  ( 1.000000000000000000, 0.000000000000000000, 0.000000000000000000 ) ) ;
#172106=CARTESIAN_POINT ( 'NONE',  ( -18.69999999999999929, -1.410778198689824459, -7.973296578895943121 ) ) ;
#172193=DIRECTION ( 'NONE',  ( 0.000000000000000000, 0.000000000000000000, 1.000000000000000000 ) ) ;
#172215=FACE_OUTER_BOUND ( 'NONE', #166702, .T. ) ;
#172224=CARTESIAN_POINT ( 'NONE',  ( 19.90000000000000568, 1.350000000000000089, 16.60000000000000142 ) ) ;
#172231=TOROIDAL_SURFACE ( 'NONE', #38920, 0.2000000000000000111, 0.1000000000000000056 ) ;
#172233=ORIENTED_EDGE ( 'NONE', *, *, #202378, .T. ) ;
#172329=AXIS2_PLACEMENT_3D ( 'NONE', #221599, #181242, #2564 ) ;
#172334=DIRECTION ( 'NONE',  ( 0.000000000000000000, -1.000000000000000000, 0.000000000000000000 ) ) ;
#172337=DIRECTION ( 'NONE',  ( 1.000000000000000000, -0.000000000000000000, -0.000000000000000000 ) ) ;
#172352=AXIS2_PLACEMENT_3D ( 'NONE', #238424, #257930, #220154 ) ;
#172369=AXIS2_PLACEMENT_3D ( 'NONE', #64588, #45035, #226199 ) ;
#172371=ORIENTED_EDGE ( 'NONE', *, *, #205890, .T. ) ;
#172448=EDGE_CURVE ( 'NONE', #174523, #190881, #77355, .T. ) ;
#172493=CARTESIAN_POINT ( 'NONE',  ( 18.79999999999999716, 0.000000000000000000, 0.000000000000000000 ) ) ;
#172507=ORIENTED_EDGE ( 'NONE', *, *, #248824, .F. ) ;
#172509=EDGE_CURVE ( 'NONE', #176334, #89225, #135630, .T. ) ;
#172518=ORIENTED_EDGE ( 'NONE', *, *, #194129, .T. ) ;
#172522=CARTESIAN_POINT ( 'NONE',  ( -18.79999999999999716, 4.513204987021263825, 22.10000000000000142 ) ) ;
#172534=EDGE_LOOP ( 'NONE', ( #108152, #244705, #65010, #209455 ) ) ;
#172554=LINE ( 'NONE', #152974, #150048 ) ;
#172574=FACE_OUTER_BOUND ( 'NONE', #170394, .T. ) ;
#172588=DIRECTION ( 'NONE',  ( 0.000000000000000000, -1.000000000000000000, 0.000000000000000000 ) ) ;
#172629=VERTEX_POINT ( 'NONE', #171242 ) ;
#172633=ADVANCED_FACE ( 'NONE', ( #94208 ), #10840, .F. ) ;
#172686=CARTESIAN_POINT ( 'NONE',  ( -0.8999999999999994671, -8.250000000000005329, 30.04142135623731136 ) ) ;
#172699=EDGE_CURVE ( 'NONE', #203823, #119804, #189989, .T. ) ;
#172709=VERTEX_POINT ( 'NONE', #137194 ) ;
#172730=ORIENTED_EDGE ( 'NONE', *, *, #132175, .T. ) ;
#172732=EDGE_CURVE ( 'NONE', #57247, #11158, #134605, .T. ) ;
#172746=CARTESIAN_POINT ( 'NONE',  ( 18.59999999999999787, -8.175168544775697654, 10.42878401658402510 ) ) ;
#172772=EDGE_CURVE ( 'NONE', #75809, #55862, #6645, .T. ) ;
#172786=DIRECTION ( 'NONE',  ( 0.000000000000000000, -0.1686199900910312910, 0.9856811345164826488 ) ) ;
#172788=CARTESIAN_POINT ( 'NONE',  ( -19.99999999999999645, 11.61130914238355771, 16.50000000000000000 ) ) ;
#172799=EDGE_CURVE ( 'NONE', #92855, #49052, #153875, .T. ) ;
#172809=VECTOR ( 'NONE', #211127, 1000.000000000000000 ) ;
#172811=AXIS2_PLACEMENT_3D ( 'NONE', #243876, #80939, #105629 ) ;
#172860=ORIENTED_EDGE ( 'NONE', *, *, #196890, .T. ) ;
#172882=ORIENTED_EDGE ( 'NONE', *, *, #183936, .F. ) ;
#172933=VERTEX_POINT ( 'NONE', #73036 ) ;
#172971=DIRECTION ( 'NONE',  ( -0.000000000000000000, -0.000000000000000000, 1.000000000000000000 ) ) ;
#172973=EDGE_CURVE ( 'NONE', #254080, #175526, #15109, .T. ) ;
#172977=DIRECTION ( 'NONE',  ( 0.000000000000000000, 0.000000000000000000, 1.000000000000000000 ) ) ;
#173043=ORIENTED_EDGE ( 'NONE', *, *, #143168, .T. ) ;
#173109=EDGE_LOOP ( 'NONE', ( #191347, #138185, #153509, #55288 ) ) ;
#173120=DIRECTION ( 'NONE',  ( 0.000000000000000000, 0.000000000000000000, -1.000000000000000000 ) ) ;
#173152=ORIENTED_EDGE ( 'NONE', *, *, #44573, .T. ) ;
#173156=EDGE_CURVE ( 'NONE', #45997, #207660, #244135, .T. ) ;
#173165=LINE ( 'NONE', #17875, #237698 ) ;
#173197=DIRECTION ( 'NONE',  ( -0.000000000000000000, -0.000000000000000000, 1.000000000000000000 ) ) ;
#173202=VERTEX_POINT ( 'NONE', #132669 ) ;
#173239=EDGE_CURVE ( 'NONE', #164655, #162415, #210913, .T. ) ;
#173310=ORIENTED_EDGE ( 'NONE', *, *, #1141, .T. ) ;
#173312=LINE ( 'NONE', #254062, #249913 ) ;
#173328=EDGE_CURVE ( 'NONE', #88949, #12989, #58489, .T. ) ;
#173336=ORIENTED_EDGE ( 'NONE', *, *, #224314, .F. ) ;
#173339=DIRECTION ( 'NONE',  ( 0.000000000000000000, -0.1686199900910313187, 0.9856811345164828708 ) ) ;
#173345=VERTEX_POINT ( 'NONE', #56931 ) ;
#173357=EDGE_CURVE ( 'NONE', #204919, #208058, #79074, .T. ) ;
#173393=ORIENTED_EDGE ( 'NONE', *, *, #257421, .T. ) ;
#173408=ADVANCED_FACE ( 'NONE', ( #197760 ), #65091, .T. ) ;
#173415=EDGE_LOOP ( 'NONE', ( #211671, #197550, #104632 ) ) ;
#173481=CARTESIAN_POINT ( 'NONE',  ( 20.10000000000000853, 4.547418889303921574, 21.90000000000000213 ) ) ;
#173488=CARTESIAN_POINT ( 'NONE',  ( -6.000000000000003553, -11.25000000000000000, 10.10000000000000142 ) ) ;
#173500=CIRCLE ( 'NONE', #60998, 0.1000000000000002554 ) ;
#173504=CARTESIAN_POINT ( 'NONE',  ( -13.40000000000000036, -9.650000000000005684, 12.40000000000000391 ) ) ;
#173511=FACE_OUTER_BOUND ( 'NONE', #169191, .T. ) ;
#173515=CARTESIAN_POINT ( 'NONE',  ( -18.69999999999999929, -18.98805597050104410, -9.034413349721665654 ) ) ;
#173524=VERTEX_POINT ( 'NONE', #248449 ) ;
#173541=ORIENTED_EDGE ( 'NONE', *, *, #223110, .T. ) ;
#173666=CARTESIAN_POINT ( 'NONE',  ( -22.94999999999999929, -11.64999999999999858, 12.09999999999999609 ) ) ;
#173672=ORIENTED_EDGE ( 'NONE', *, *, #18240, .F. ) ;
#173748=AXIS2_PLACEMENT_3D ( 'NONE', #252113, #232592, #197282 ) ;
#173757=ADVANCED_FACE ( 'NONE', ( #206138 ), #27540, .T. ) ;
#173820=CIRCLE ( 'NONE', #39939, 4.000000000000000000 ) ;
#173851=CARTESIAN_POINT ( 'NONE',  ( -18.69999999999999929, -8.350000000000004974, 10.52591260281975138 ) ) ;
#173857=DIRECTION ( 'NONE',  ( -0.000000000000000000, 6.938893903907270030E-14, 1.000000000000000000 ) ) ;
#173863=VECTOR ( 'NONE', #62607, 1000.000000000000000 ) ;
#173899=EDGE_CURVE ( 'NONE', #20074, #166706, #230858, .T. ) ;
#173914=EDGE_CURVE ( 'NONE', #82512, #244339, #54753, .T. ) ;
#173936=CYLINDRICAL_SURFACE ( 'NONE', #10023, 0.1000000000000001443 ) ;
#173971=DIRECTION ( 'NONE',  ( 1.000000000000000000, -0.000000000000000000, -0.000000000000000000 ) ) ;
#173984=ORIENTED_EDGE ( 'NONE', *, *, #164262, .T. ) ;
#173991=CARTESIAN_POINT ( 'NONE',  ( -18.79999999999999716, -1.885425182446133885, -11.49641995933507843 ) ) ;
#173993=ORIENTED_EDGE ( 'NONE', *, *, #98559, .T. ) ;
#174039=ORIENTED_EDGE ( 'NONE', *, *, #131008, .F. ) ;
#174047=ADVANCED_FACE ( 'NONE', ( #44200 ), #165427, .T. ) ;
#174099=CIRCLE ( 'NONE', #203089, 0.09999999999999939493 ) ;
#174115=ORIENTED_EDGE ( 'NONE', *, *, #221092, .T. ) ;
#174149=CARTESIAN_POINT ( 'NONE',  ( -20.90000000000000213, 1.899104650876408451, -11.59795743183152972 ) ) ;
#174160=CIRCLE ( 'NONE', #236462, 0.09999999999999939493 ) ;
#174182=CARTESIAN_POINT ( 'NONE',  ( 20.90000000000000213, 0.000000000000000000, 0.000000000000000000 ) ) ;
#174258=ORIENTED_EDGE ( 'NONE', *, *, #245202, .T. ) ;
#174306=CIRCLE ( 'NONE', #215924, 0.1000000000000002554 ) ;
#174312=DIRECTION ( 'NONE',  ( 0.000000000000000000, 0.000000000000000000, -1.000000000000000000 ) ) ;
#174314=CARTESIAN_POINT ( 'NONE',  ( -22.19999999999999929, -11.65000000000000036, 12.09999999999999609 ) ) ;
#174336=CARTESIAN_POINT ( 'NONE',  ( 20.90000000000000213, 7.986648289447971116, -1.311673547813416718 ) ) ;
#174358=CARTESIAN_POINT ( 'NONE',  ( 18.59999999999999787, -10.64999999999999325, 31.59999999999999787 ) ) ;
#174366=DIRECTION ( 'NONE',  ( 1.000000000000000000, 0.000000000000000000, 0.000000000000000000 ) ) ;
#174463=CYLINDRICAL_SURFACE ( 'NONE', #71403, 0.09999999999999939493 ) ;
#174476=DIRECTION ( 'NONE',  ( 0.000000000000000000, -0.1686199900910312910, 0.9856811345164826488 ) ) ;
#174484=CARTESIAN_POINT ( 'NONE',  ( -21.00983514138059860, 6.346420624576638581, 11.97684634237457502 ) ) ;
#174493=DIRECTION ( 'NONE',  ( 1.000000000000000000, -0.000000000000000000, -0.000000000000000000 ) ) ;
#174523=VERTEX_POINT ( 'NONE', #243350 ) ;
#174538=CARTESIAN_POINT ( 'NONE',  ( -18.69999999999999929, 4.513204987021268266, 22.10000000000000142 ) ) ;
#174540=ORIENTED_EDGE ( 'NONE', *, *, #221857, .F. ) ;
#174554=EDGE_LOOP ( 'NONE', ( #213707, #3921, #95585, #134252 ) ) ;
#174612=EDGE_LOOP ( 'NONE', ( #35210, #47983, #24694, #50296 ) ) ;
#174635=CARTESIAN_POINT ( 'NONE',  ( -18.79999999999999716, -1.212568896937008089, -8.000000000000000000 ) ) ;
#174648=EDGE_LOOP ( 'NONE', ( #156595, #215900, #241285, #121627 ) ) ;
#174651=CARTESIAN_POINT ( 'NONE',  ( 22.20000000000000284, 6.223900101154161923, 12.09999999999999964 ) ) ;
#174672=PLANE ( 'NONE',  #60496 ) ;
#174703=ADVANCED_FACE ( 'NONE', ( #94534 ), #29481, .F. ) ;
#174708=ORIENTED_EDGE ( 'NONE', *, *, #225856, .T. ) ;
#174747=DIRECTION ( 'NONE',  ( 1.000000000000000000, 0.000000000000000000, 0.000000000000000000 ) ) ;
#174790=DIRECTION ( 'NONE',  ( 1.000000000000000000, 0.000000000000000000, 0.000000000000000000 ) ) ;
#174812=CYLINDRICAL_SURFACE ( 'NONE', #207941, 0.09999999999999939493 ) ;
#174821=CIRCLE ( 'NONE', #249603, 0.09999999999999939493 ) ;
#174844=AXIS2_PLACEMENT_3D ( 'NONE', #110181, #245856, #210579 ) ;
#174894=DIRECTION ( 'NONE',  ( 0.000000000000000000, 0.9856811345164829818, 0.1686199900910294314 ) ) ;
#174908=EDGE_LOOP ( 'NONE', ( #222990, #198038, #124658, #224723 ) ) ;
#174965=FACE_OUTER_BOUND ( 'NONE', #207809, .T. ) ;
#174967=CARTESIAN_POINT ( 'NONE',  ( -0.8999999999999993561, -8.250000000000005329, 26.00000000000000355 ) ) ;
#174992=EDGE_CURVE ( 'NONE', #136640, #254397, #4421, .T. ) ;
#175101=VECTOR ( 'NONE', #127182, 1000.000000000000000 ) ;
#175126=LINE ( 'NONE', #141091, #248719 ) ;
#175180=ADVANCED_FACE ( 'NONE', ( #253305 ), #55083, .T. ) ;
#175186=CYLINDRICAL_SURFACE ( 'NONE', #251357, 0.1000000000000002554 ) ;
#175190=ADVANCED_FACE ( 'NONE', ( #4122 ), #41992, .F. ) ;
#175199=CIRCLE ( 'NONE', #237696, 0.09999999999999939493 ) ;
#175204=ORIENTED_EDGE ( 'NONE', *, *, #142931, .T. ) ;
#175225=EDGE_CURVE ( 'NONE', #223079, #243012, #23728, .T. ) ;
#175337=LINE ( 'NONE', #91909, #28768 ) ;
#175359=TOROIDAL_SURFACE ( 'NONE', #83712, 0.2000000000000000111, 0.1000000000000000056 ) ;
#175395=DIRECTION ( 'NONE',  ( -0.000000000000000000, -1.000000000000000000, 4.336808689942043611E-14 ) ) ;
#175422=DIRECTION ( 'NONE',  ( 0.000000000000000000, 0.000000000000000000, -1.000000000000000000 ) ) ;
#175431=DIRECTION ( 'NONE',  ( -0.000000000000000000, 0.000000000000000000, -1.000000000000000000 ) ) ;
#175434=DIRECTION ( 'NONE',  ( 0.000000000000000000, 0.000000000000000000, -1.000000000000000000 ) ) ;
#175471=ORIENTED_EDGE ( 'NONE', *, *, #172699, .T. ) ;
#175515=CARTESIAN_POINT ( 'NONE',  ( -22.10000000000000142, -11.75000000000000000, 32.89999999999999858 ) ) ;
#175516=AXIS2_PLACEMENT_3D ( 'NONE', #76994, #136968, #117416 ) ;
#175526=VERTEX_POINT ( 'NONE', #204254 ) ;
#175549=CARTESIAN_POINT ( 'NONE',  ( 21.00000000000000000, 1.410778198689825347, -7.973296578895943121 ) ) ;
#175590=AXIS2_PLACEMENT_3D ( 'NONE', #156430, #55979, #213797 ) ;
#175600=LINE ( 'NONE', #114327, #22867 ) ;
#175604=AXIS2_PLACEMENT_3D ( 'NONE', #141725, #179599, #122182 ) ;
#175623=EDGE_LOOP ( 'NONE', ( #233604, #197785, #13058, #230057 ) ) ;
#175633=CIRCLE ( 'NONE', #42511, 0.1000000000000028644 ) ;
#175637=LINE ( 'NONE', #216012, #205531 ) ;
#175643=DIRECTION ( 'NONE',  ( 0.000000000000000000, -0.1335171055202867274, 0.9910465087640865089 ) ) ;
#175675=CIRCLE ( 'NONE', #229815, 0.1000000000000000749 ) ;
#175695=EDGE_CURVE ( 'NONE', #157545, #145044, #170326, .T. ) ;
#175764=ORIENTED_EDGE ( 'NONE', *, *, #20918, .F. ) ;
#175771=LINE ( 'NONE', #96197, #171080 ) ;
#175777=CARTESIAN_POINT ( 'NONE',  ( 21.06025298249095457, 6.342459739380975847, 12.00000000173893078 ) ) ;
#175791=LINE ( 'NONE', #40143, #120189 ) ;
#175840=CARTESIAN_POINT ( 'NONE',  ( -20.90000000000000213, -1.410778198689825347, -7.973296578895943121 ) ) ;
#175843=ORIENTED_EDGE ( 'NONE', *, *, #59822, .F. ) ;
#175848=ORIENTED_EDGE ( 'NONE', *, *, #138721, .F. ) ;
#175874=EDGE_LOOP ( 'NONE', ( #141743, #45478, #13986, #99756 ) ) ;
#175917=CARTESIAN_POINT ( 'NONE',  ( -5.900000000000003020, -11.34999999999999964, 10.10000000000000142 ) ) ;
#175929=DIRECTION ( 'NONE',  ( 0.000000000000000000, -1.000000000000000000, 0.000000000000000000 ) ) ;
#175934=ORIENTED_EDGE ( 'NONE', *, *, #231964, .F. ) ;
#175959=CARTESIAN_POINT ( 'NONE',  ( 13.40000000000000036, -11.65000000000000036, 12.40000000000000391 ) ) ;
#175969=LINE ( 'NONE', #255423, #207227 ) ;
#175981=DIRECTION ( 'NONE',  ( -1.000000000000000000, 0.000000000000000000, 0.000000000000000000 ) ) ;
#175991=ORIENTED_EDGE ( 'NONE', *, *, #174992, .F. ) ;
#176008=CARTESIAN_POINT ( 'NONE',  ( 21.10000000000000142, 0.000000000000000000, -4.100000000000000533 ) ) ;
#176025=EDGE_CURVE ( 'NONE', #161437, #40449, #228869, .T. ) ;
#176051=CARTESIAN_POINT ( 'NONE',  ( -20.90000000000000213, 1.885425182446133885, -11.49641995933507843 ) ) ;
#176063=VECTOR ( 'NONE', #239638, 1000.000000000000000 ) ;
#176067=LINE ( 'NONE', #117351, #72315 ) ;
#176111=DIRECTION ( 'NONE',  ( 1.000000000000000000, 0.000000000000000000, 0.000000000000000000 ) ) ;
#176129=LINE ( 'NONE', #39187, #35036 ) ;
#176153=ORIENTED_EDGE ( 'NONE', *, *, #223110, .F. ) ;
#176170=DIRECTION ( 'NONE',  ( -1.000000000000000000, 0.000000000000000000, 0.000000000000000000 ) ) ;
#176185=CARTESIAN_POINT ( 'NONE',  ( 11.60000000000000320, -8.250000000000003553, 12.40000000000000391 ) ) ;
#176189=AXIS2_PLACEMENT_3D ( 'NONE', #113613, #51032, #211431 ) ;
#176227=CARTESIAN_POINT ( 'NONE',  ( -18.79999999999999716, 1.350000000000000089, 16.60000000000000142 ) ) ;
#176257=TOROIDAL_SURFACE ( 'NONE', #242863, 0.2000000000000000111, 0.1000000000000000056 ) ;
#176271=CARTESIAN_POINT ( 'NONE',  ( 20.99999999999998934, 7.986648289447971116, -1.311673547813416718 ) ) ;
#176280=DIRECTION ( 'NONE',  ( -1.000000000000000000, 0.000000000000000000, 0.000000000000000000 ) ) ;
#176282=VERTEX_POINT ( 'NONE', #118202 ) ;
#176283=AXIS2_PLACEMENT_3D ( 'NONE', #67424, #249918, #71301 ) ;
#176334=VERTEX_POINT ( 'NONE', #20401 ) ;
#176349=CARTESIAN_POINT ( 'NONE',  ( -19.99999999999999645, 5.552655413246002425, 16.61686199900910310 ) ) ;
#176352=EDGE_CURVE ( 'NONE', #246137, #104540, #183263, .T. ) ;
#176354=CIRCLE ( 'NONE', #147096, 11.65000000000000036 ) ;
#176482=DIRECTION ( 'NONE',  ( 1.000000000000000000, 0.000000000000000000, 0.000000000000000000 ) ) ;
#176486=EDGE_CURVE ( 'NONE', #161554, #97541, #204744, .T. ) ;
#176577=CIRCLE ( 'NONE', #26552, 0.1000000000000002554 ) ;
#176615=DIRECTION ( 'NONE',  ( 1.000000000000000000, 0.000000000000000000, 0.000000000000000000 ) ) ;
#176619=AXIS2_PLACEMENT_3D ( 'NONE', #52362, #152804, #74562 ) ;
#176625=ADVANCED_FACE ( 'NONE', ( #168926 ), #257039, .F. ) ;
#176627=ORIENTED_EDGE ( 'NONE', *, *, #145870, .T. ) ;
#176716=VERTEX_POINT ( 'NONE', #79713 ) ;
#176727=FACE_OUTER_BOUND ( 'NONE', #30794, .T. ) ;
#176777=TOROIDAL_SURFACE ( 'NONE', #255821, 2.699999999999999734, 0.1000000000000000056 ) ;
#176800=DIRECTION ( 'NONE',  ( 0.000000000000000000, 0.000000000000000000, -1.000000000000000000 ) ) ;
#176884=VERTEX_POINT ( 'NONE', #112164 ) ;
#176903=VERTEX_POINT ( 'NONE', #131702 ) ;
#176938=DIRECTION ( 'NONE',  ( 1.000000000000000000, 0.000000000000000000, 0.000000000000000000 ) ) ;
#176958=CARTESIAN_POINT ( 'NONE',  ( -22.94999999999999929, 4.611773100472912112, 22.11686199900910665 ) ) ;
#176987=CARTESIAN_POINT ( 'NONE',  ( 20.10000000000000497, 5.552655413246002425, 16.61686199900910310 ) ) ;
#177009=CARTESIAN_POINT ( 'NONE',  ( -22.19999999999999929, -11.65000000000000036, 9.900000000000002132 ) ) ;
#177040=FACE_OUTER_BOUND ( 'NONE', #188628, .T. ) ;
#177056=DIRECTION ( 'NONE',  ( -0.000000000000000000, 1.000000000000000000, -0.000000000000000000 ) ) ;
#177077=ORIENTED_EDGE ( 'NONE', *, *, #137657, .F. ) ;
#177152=CARTESIAN_POINT ( 'NONE',  ( -22.94999999999999929, -11.75000000000000178, 0.000000000000000000 ) ) ;
#177170=CIRCLE ( 'NONE', #64707, 11.75000000000000000 ) ;
#177200=CARTESIAN_POINT ( 'NONE',  ( -37.88850191057539973, -9.849999999999994316, 30.09999999999999076 ) ) ;
#177218=ORIENTED_EDGE ( 'NONE', *, *, #133215, .F. ) ;
#177266=EDGE_CURVE ( 'NONE', #132961, #175526, #170580, .T. ) ;
#177305=EDGE_CURVE ( 'NONE', #88949, #176903, #148926, .T. ) ;
#177308=CARTESIAN_POINT ( 'NONE',  ( -13.40000000000000036, -8.250000000000007105, 17.60000000000000497 ) ) ;
#177384=EDGE_LOOP ( 'NONE', ( #103980, #11688, #110124, #70899 ) ) ;
#177474=EDGE_CURVE ( 'NONE', #163992, #163656, #225025, .T. ) ;
#177494=ORIENTED_EDGE ( 'NONE', *, *, #98510, .F. ) ;
#177588=DIRECTION ( 'NONE',  ( -1.000000000000000000, 0.000000000000000000, 0.000000000000000000 ) ) ;
#177665=CARTESIAN_POINT ( 'NONE',  ( 21.00000000000000000, 0.000000000000000000, 0.000000000000000000 ) ) ;
#177668=CARTESIAN_POINT ( 'NONE',  ( -21.00000000000000000, 6.644425182197215562, 9.641788261573355001 ) ) ;
#177684=DIRECTION ( 'NONE',  ( -0.000000000000000000, -0.000000000000000000, -1.000000000000000000 ) ) ;
#177743=DIRECTION ( 'NONE',  ( -1.000000000000000000, 0.000000000000000000, 0.000000000000000000 ) ) ;
#177758=DIRECTION ( 'NONE',  ( 1.000000000000000000, 0.000000000000000000, -0.000000000000000000 ) ) ;
#177839=CARTESIAN_POINT ( 'NONE',  ( 18.59999999999999787, -11.75000000000000000, 30.09999999999999787 ) ) ;
#177878=CARTESIAN_POINT ( 'NONE',  ( 20.01715728752538936, 5.586869315528661062, 16.41686199900910736 ) ) ;
#178008=CARTESIAN_POINT ( 'NONE',  ( -6.000000000000002665, -11.34999999999999964, 14.00000000000000178 ) ) ;
#178041=VERTEX_POINT ( 'NONE', #231188 ) ;
#178081=DIRECTION ( 'NONE',  ( -1.000000000000000000, 0.000000000000000000, 0.000000000000000000 ) ) ;
#178094=DIRECTION ( 'NONE',  ( -0.000000000000000000, -0.9868171638914224886, -0.1618390714546072695 ) ) ;
#178103=ADVANCED_FACE ( 'NONE', ( #257092 ), #78489, .T. ) ;
#178173=DIRECTION ( 'NONE',  ( 0.000000000000000000, -1.224646799147353207E-16, 1.000000000000000000 ) ) ;
#178183=DIRECTION ( 'NONE',  ( -1.284434275755705296E-16, 0.7071067811865471286, 0.7071067811865479058 ) ) ;
#178190=CARTESIAN_POINT ( 'NONE',  ( 5.899999999999997691, -11.34999999999999964, 13.90000000000000213 ) ) ;
#178273=DIRECTION ( 'NONE',  ( 0.000000000000000000, 0.1335171055202901413, -0.9910465087640860649 ) ) ;
#178305=CARTESIAN_POINT ( 'NONE',  ( -20.90000000000000213, 0.000000000000000000, 0.000000000000000000 ) ) ;
#178331=FACE_OUTER_BOUND ( 'NONE', #166038, .T. ) ;
#178340=ORIENTED_EDGE ( 'NONE', *, *, #136688, .T. ) ;
#178355=AXIS2_PLACEMENT_3D ( 'NONE', #40638, #199695, #21059 ) ;
#178392=CARTESIAN_POINT ( 'NONE',  ( 18.79999999999999716, -11.65000000000000036, 32.89999999999999858 ) ) ;
#178403=ADVANCED_FACE ( 'NONE', ( #94864 ), #182029, .T. ) ;
#178426=DIRECTION ( 'NONE',  ( 0.000000000000000000, 0.000000000000000000, -1.000000000000000000 ) ) ;
#178445=ORIENTED_EDGE ( 'NONE', *, *, #65886, .T. ) ;
#178453=CARTESIAN_POINT ( 'NONE',  ( -11.60000000000000320, -9.650000000000005684, 12.40000000000000391 ) ) ;
#178479=CARTESIAN_POINT ( 'NONE',  ( -21.00000000000000000, 6.258114003436814343, 11.90000000000000036 ) ) ;
#178499=ORIENTED_EDGE ( 'NONE', *, *, #14271, .F. ) ;
#178540=AXIS2_PLACEMENT_3D ( 'NONE', #13374, #208994, #91617 ) ;
#178545=CARTESIAN_POINT ( 'NONE',  ( -19.95857864376268509, 4.513204987021262937, 22.00000000000000355 ) ) ;
#178549=EDGE_LOOP ( 'NONE', ( #242162, #93088, #78501, #239811 ) ) ;
#178553=CARTESIAN_POINT ( 'NONE',  ( -18.69999999999999929, 7.799999999999999822, 1.212568896937007867 ) ) ;
#178583=CARTESIAN_POINT ( 'NONE',  ( 21.10000000000000142, 0.000000000000000000, 0.000000000000000000 ) ) ;
#178602=AXIS2_PLACEMENT_3D ( 'NONE', #251049, #50277, #13738 ) ;
#178622=ORIENTED_EDGE ( 'NONE', *, *, #50018, .F. ) ;
#178631=EDGE_CURVE ( 'NONE', #108582, #183834, #190434, .T. ) ;
#178635=ORIENTED_EDGE ( 'NONE', *, *, #95700, .F. ) ;
#178645=DIRECTION ( 'NONE',  ( 0.000000000000000000, 0.000000000000000000, -1.000000000000000000 ) ) ;
#178674=CARTESIAN_POINT ( 'NONE',  ( -22.94999999999999929, 8.000000000000000000, 1.212568896937007867 ) ) ;
#178689=DIRECTION ( 'NONE',  ( 0.000000000000000000, 0.000000000000000000, -1.000000000000000000 ) ) ;
#178720=ORIENTED_EDGE ( 'NONE', *, *, #104326, .F. ) ;
#178912=CIRCLE ( 'NONE', #103836, 4.900000000000003020 ) ;
#178919=VECTOR ( 'NONE', #18914, 1000.000000000000000 ) ;
#178956=CARTESIAN_POINT ( 'NONE',  ( -22.94999999999999929, -1.885425182446134107, -11.49641995933507843 ) ) ;
#179011=EDGE_LOOP ( 'NONE', ( #220489, #194144, #63246 ) ) ;
#179052=DIRECTION ( 'NONE',  ( 0.000000000000000000, 1.000000000000000000, 0.000000000000000000 ) ) ;
#179078=VERTEX_POINT ( 'NONE', #209079 ) ;
#179086=VECTOR ( 'NONE', #6322, 1000.000000000000000 ) ;
#179087=EDGE_CURVE ( 'NONE', #168244, #169705, #153397, .T. ) ;
#179095=FACE_OUTER_BOUND ( 'NONE', #249273, .T. ) ;
#179109=DIRECTION ( 'NONE',  ( 1.000000000000000000, 0.000000000000000000, 0.000000000000000000 ) ) ;
#179142=CARTESIAN_POINT ( 'NONE',  ( -37.88850191057539973, -10.80884033489985363, 6.000000000000001776 ) ) ;
#179162=DIRECTION ( 'NONE',  ( 0.000000000000000000, 0.000000000000000000, -1.000000000000000000 ) ) ;
#179179=ORIENTED_EDGE ( 'NONE', *, *, #233784, .F. ) ;
#179195=CARTESIAN_POINT ( 'NONE',  ( 20.90000000000000213, 1.885425182446133885, -11.49641995933507843 ) ) ;
#179268=ORIENTED_EDGE ( 'NONE', *, *, #101136, .T. ) ;
#179314=EDGE_CURVE ( 'NONE', #13384, #149370, #61768, .T. ) ;
#179370=EDGE_CURVE ( 'NONE', #217909, #103588, #235071, .T. ) ;
#179396=AXIS2_PLACEMENT_3D ( 'NONE', #220902, #256123, #119268 ) ;
#179397=ORIENTED_EDGE ( 'NONE', *, *, #217176, .T. ) ;
#179447=AXIS2_PLACEMENT_3D ( 'NONE', #248813, #50575, #149730 ) ;
#179492=DIRECTION ( 'NONE',  ( -1.000000000000000000, 0.000000000000000000, 0.000000000000000000 ) ) ;
#179577=CARTESIAN_POINT ( 'NONE',  ( -18.69999999999999929, 1.350000000000000089, 16.39999999999999858 ) ) ;
#179599=DIRECTION ( 'NONE',  ( -1.000000000000000000, 0.000000000000000000, 0.000000000000000000 ) ) ;
#179617=DIRECTION ( 'NONE',  ( -1.000000000000000000, -0.000000000000000000, -0.000000000000000000 ) ) ;
#179690=ORIENTED_EDGE ( 'NONE', *, *, #35431, .F. ) ;
#179700=ADVANCED_FACE ( 'NONE', ( #45391 ), #184901, .F. ) ;
#179704=CARTESIAN_POINT ( 'NONE',  ( -18.79999999999999716, 2.168342339202985247, -13.59640602015278432 ) ) ;
#179723=ORIENTED_EDGE ( 'NONE', *, *, #202432, .T. ) ;
#179729=ORIENTED_EDGE ( 'NONE', *, *, #246068, .F. ) ;
#179803=EDGE_LOOP ( 'NONE', ( #78951, #205691, #116974, #57500 ) ) ;
#179826=FACE_OUTER_BOUND ( 'NONE', #50119, .T. ) ;
#179895=ADVANCED_FACE ( 'NONE', ( #93173 ), #28873, .T. ) ;
#179908=DIRECTION ( 'NONE',  ( 0.000000000000000000, 0.000000000000000000, -1.000000000000000000 ) ) ;
#179911=LINE ( 'NONE', #157810, #161969 ) ;
#179944=DIRECTION ( 'NONE',  ( 1.000000000000000000, 0.000000000000000000, 0.000000000000000000 ) ) ;
#179963=DIRECTION ( 'NONE',  ( 0.000000000000000000, -1.000000000000000000, 0.000000000000000000 ) ) ;
#179996=FACE_OUTER_BOUND ( 'NONE', #133249, .T. ) ;
#180008=CARTESIAN_POINT ( 'NONE',  ( 11.60000000000000320, -11.65000000000000036, 12.30000000000000426 ) ) ;
#180031=EDGE_LOOP ( 'NONE', ( #17901, #244402 ) ) ;
#180072=CARTESIAN_POINT ( 'NONE',  ( -18.69999999999999929, 1.350000000000000089, 21.90000000000000213 ) ) ;
#180163=CIRCLE ( 'NONE', #242493, 0.2000000000000005107 ) ;
#180188=EDGE_LOOP ( 'NONE', ( #54087, #148882, #144181, #120062 ) ) ;
#180193=ORIENTED_EDGE ( 'NONE', *, *, #90536, .T. ) ;
#180232=DIRECTION ( 'NONE',  ( 0.000000000000000000, -0.000000000000000000, -1.000000000000000000 ) ) ;
#180239=EDGE_LOOP ( 'NONE', ( #234024, #235380, #62225, #137519 ) ) ;
#180277=ADVANCED_FACE ( 'NONE', ( #73352 ), #48608, .T. ) ;
#180279=ORIENTED_EDGE ( 'NONE', *, *, #3501, .F. ) ;
#180299=CARTESIAN_POINT ( 'NONE',  ( -18.79999999999999716, 1.350000000000000089, 22.00000000000000355 ) ) ;
#180304=DIRECTION ( 'NONE',  ( 0.000000000000000000, 0.000000000000000000, 1.000000000000000000 ) ) ;
#180310=AXIS2_PLACEMENT_3D ( 'NONE', #67433, #226486, #88254 ) ;
#180322=EDGE_LOOP ( 'NONE', ( #234263, #173984, #97808, #63960 ) ) ;
#180324=AXIS2_PLACEMENT_3D ( 'NONE', #18232, #235978, #61205 ) ;
#180333=AXIS2_PLACEMENT_3D ( 'NONE', #217816, #238686, #237409 ) ;
#180345=DIRECTION ( 'NONE',  ( 1.476360405086644309E-16, -1.000000000000000000, -0.000000000000000000 ) ) ;
#180416=VECTOR ( 'NONE', #29961, 1000.000000000000000 ) ;
#180432=CARTESIAN_POINT ( 'NONE',  ( 19.90000000000000568, 5.586869315528661062, 16.41686199900910736 ) ) ;
#180444=CARTESIAN_POINT ( 'NONE',  ( 19.90000000000000568, 11.61130914238355771, 16.60000000000000142 ) ) ;
#180483=DIRECTION ( 'NONE',  ( 0.000000000000000000, 1.000000000000000000, 0.000000000000000000 ) ) ;
#180502=FACE_OUTER_BOUND ( 'NONE', #167242, .T. ) ;
#180507=AXIS2_PLACEMENT_3D ( 'NONE', #219282, #181467, #40700 ) ;
#180514=DIRECTION ( 'NONE',  ( 0.000000000000000000, -0.7071067811865479058, -0.7071067811865472397 ) ) ;
#180527=FACE_OUTER_BOUND ( 'NONE', #245675, .T. ) ;
#180535=EDGE_LOOP ( 'NONE', ( #54543, #120725, #181355, #7966 ) ) ;
#180544=AXIS2_PLACEMENT_3D ( 'NONE', #739, #137696, #80274 ) ;
#180561=AXIS2_PLACEMENT_3D ( 'NONE', #42055, #6757, #62882 ) ;
#180569=DIRECTION ( 'NONE',  ( 0.000000000000000000, 0.000000000000000000, -1.000000000000000000 ) ) ;
#180583=SPHERICAL_SURFACE ( 'NONE', #67366, 0.1000000000000000056 ) ;
#180617=DIRECTION ( 'NONE',  ( 0.000000000000000000, -0.9868171638914228216, 0.1618390714546044939 ) ) ;
#180645=EDGE_CURVE ( 'NONE', #221804, #22186, #87439, .T. ) ;
#180649=CARTESIAN_POINT ( 'NONE',  ( -18.69999999999999929, -1.212568896937008089, -7.800000000000000711 ) ) ;
#180652=CIRCLE ( 'NONE', #68226, 0.09999999999999993616 ) ;
#180705=CIRCLE ( 'NONE', #238976, 0.1999999999999987899 ) ;
#180720=DIRECTION ( 'NONE',  ( 0.000000000000000000, 0.000000000000000000, 1.000000000000000000 ) ) ;
#180721=VECTOR ( 'NONE', #219409, 1000.000000000000000 ) ;
#180756=CARTESIAN_POINT ( 'NONE',  ( 18.79999999999999361, -11.75000000000000000, 5.900000000000001243 ) ) ;
#180759=AXIS2_PLACEMENT_3D ( 'NONE', #216570, #75786, #217831 ) ;
#180766=ORIENTED_EDGE ( 'NONE', *, *, #41890, .T. ) ;
#180794=CARTESIAN_POINT ( 'NONE',  ( -18.79999999999999716, -11.65000000000000036, -15.00000000000000000 ) ) ;
#180804=VECTOR ( 'NONE', #37112, 1000.000000000000000 ) ;
#180815=FACE_OUTER_BOUND ( 'NONE', #107165, .T. ) ;
#180868=LINE ( 'NONE', #219978, #194216 ) ;
#180873=VECTOR ( 'NONE', #186295, 1000.000000000000000 ) ;
#180885=CIRCLE ( 'NONE', #176619, 0.09999999999999939493 ) ;
#180916=LINE ( 'NONE', #195366, #141359 ) ;
#180950=CARTESIAN_POINT ( 'NONE',  ( -11.60000000000000320, -8.279289321881350361, 15.00000000000000355 ) ) ;
#180976=PLANE ( 'NONE',  #232161 ) ;
#181190=VERTEX_POINT ( 'NONE', #154842 ) ;
#181242=DIRECTION ( 'NONE',  ( -5.204170427930453469E-14, 1.000000000000000000, -0.000000000000000000 ) ) ;
#181254=FACE_OUTER_BOUND ( 'NONE', #257741, .T. ) ;
#181259=DIRECTION ( 'NONE',  ( -0.000000000000000000, 1.000000000000000000, 0.000000000000000000 ) ) ;
#181267=ORIENTED_EDGE ( 'NONE', *, *, #70054, .T. ) ;
#181269=CARTESIAN_POINT ( 'NONE',  ( 20.00000000000000355, 4.547418889303922462, 21.90000000000000213 ) ) ;
#181275=DIRECTION ( 'NONE',  ( 1.000000000000000000, 0.000000000000000000, 0.000000000000000000 ) ) ;
#181278=CARTESIAN_POINT ( 'NONE',  ( -5.900000000000003020, -11.65000000000000036, 10.10000000000000142 ) ) ;
#181279=EDGE_CURVE ( 'NONE', #171946, #58688, #83885, .T. ) ;
#181283=DIRECTION ( 'NONE',  ( 0.000000000000000000, 0.000000000000000000, 1.000000000000000000 ) ) ;
#181309=CARTESIAN_POINT ( 'NONE',  ( 18.69999999999999929, 7.973296578895943121, -1.410778198689827123 ) ) ;
#181351=ORIENTED_EDGE ( 'NONE', *, *, #117758, .T. ) ;
#181355=ORIENTED_EDGE ( 'NONE', *, *, #194309, .F. ) ;
#181390=ORIENTED_EDGE ( 'NONE', *, *, #138799, .F. ) ;
#181404=DIRECTION ( 'NONE',  ( 1.000000000000000000, -0.000000000000000000, 0.000000000000000000 ) ) ;
#181409=CARTESIAN_POINT ( 'NONE',  ( 19.90000000000000924, 4.513204987021263825, 22.10000000000000142 ) ) ;
#181414=VECTOR ( 'NONE', #247331, 1000.000000000000000 ) ;
#181418=ORIENTED_EDGE ( 'NONE', *, *, #124434, .F. ) ;
#181466=VERTEX_POINT ( 'NONE', #35549 ) ;
#181467=DIRECTION ( 'NONE',  ( 0.000000000000000000, 1.000000000000000000, 0.000000000000000000 ) ) ;
#181510=ORIENTED_EDGE ( 'NONE', *, *, #130128, .F. ) ;
#181516=LINE ( 'NONE', #84924, #49182 ) ;
#181546=CARTESIAN_POINT ( 'NONE',  ( -18.69999999999999929, 1.149999999999999911, 16.60000000000000142 ) ) ;
#181582=LINE ( 'NONE', #245399, #122325 ) ;
#181590=CARTESIAN_POINT ( 'NONE',  ( -19.89999999999999858, 4.611773100472912112, 22.11686199900910665 ) ) ;
#181597=CARTESIAN_POINT ( 'NONE',  ( 22.94999999999999929, 4.898587196589412829E-16, -4.000000000000000000 ) ) ;
#181603=FACE_OUTER_BOUND ( 'NONE', #179803, .T. ) ;
#181630=EDGE_CURVE ( 'NONE', #34286, #12756, #101879, .T. ) ;
#181638=LINE ( 'NONE', #102059, #209747 ) ;
#181665=VERTEX_POINT ( 'NONE', #109599 ) ;
#181673=ORIENTED_EDGE ( 'NONE', *, *, #75031, .F. ) ;
#181684=ORIENTED_EDGE ( 'NONE', *, *, #60826, .F. ) ;
#181704=ORIENTED_EDGE ( 'NONE', *, *, #110202, .T. ) ;
#181710=CARTESIAN_POINT ( 'NONE',  ( -20.90000000000000213, 7.986648289447971116, -1.311673547813416718 ) ) ;
#181764=EDGE_CURVE ( 'NONE', #217337, #181466, #82078, .T. ) ;
#181909=ORIENTED_EDGE ( 'NONE', *, *, #222194, .T. ) ;
#181914=LINE ( 'NONE', #123220, #255884 ) ;
#181931=CIRCLE ( 'NONE', #148816, 0.1000000000000028644 ) ;
#181950=DIRECTION ( 'NONE',  ( -2.489438768765008884E-17, -0.1686199900910312910, 0.9856811345164826488 ) ) ;
#181983=AXIS2_PLACEMENT_3D ( 'NONE', #237717, #235149, #138573 ) ;
#182019=DIRECTION ( 'NONE',  ( 0.000000000000000000, 0.000000000000000000, -1.000000000000000000 ) ) ;
#182029=TOROIDAL_SURFACE ( 'NONE', #236189, 0.2000000000000000111, 0.1000000000000000056 ) ;
#182062=DIRECTION ( 'NONE',  ( -1.000000000000000000, 0.000000000000000000, 0.000000000000000000 ) ) ;
#182091=CARTESIAN_POINT ( 'NONE',  ( 18.69999999999999929, 5.488301202077013663, 16.39999999999999858 ) ) ;
#182097=ORIENTED_EDGE ( 'NONE', *, *, #82486, .T. ) ;
#182127=DIRECTION ( 'NONE',  ( 1.000000000000000000, -0.000000000000000000, 0.000000000000000000 ) ) ;
#182139=VERTEX_POINT ( 'NONE', #108034 ) ;
#182143=DIRECTION ( 'NONE',  ( -1.645090726704136556E-14, -0.1618390714546045217, 0.9868171638914230437 ) ) ;
#182195=EDGE_CURVE ( 'NONE', #162811, #163992, #158737, .T. ) ;
#182296=CIRCLE ( 'NONE', #165553, 0.09999999999999939493 ) ;
#182331=CARTESIAN_POINT ( 'NONE',  ( -5.900000000000002132, -11.65000000000000036, 13.90000000000000213 ) ) ;
#182466=CARTESIAN_POINT ( 'NONE',  ( 11.60000000000000142, -11.75000000000000000, 12.30000000000000426 ) ) ;
#182469=VECTOR ( 'NONE', #107920, 1000.000000000000000 ) ;
#182490=EDGE_CURVE ( 'NONE', #110926, #82512, #660, .T. ) ;
#182505=ORIENTED_EDGE ( 'NONE', *, *, #162166, .T. ) ;
#182512=CARTESIAN_POINT ( 'NONE',  ( 18.69999999999999929, -1.467286812112899463, 32.89999999999999858 ) ) ;
#182582=ORIENTED_EDGE ( 'NONE', *, *, #131058, .T. ) ;
#182593=AXIS2_PLACEMENT_3D ( 'NONE', #37999, #138326, #117509 ) ;
#182680=VERTEX_POINT ( 'NONE', #73752 ) ;
#182697=ORIENTED_EDGE ( 'NONE', *, *, #120871, .T. ) ;
#182700=EDGE_CURVE ( 'NONE', #110943, #159030, #115410, .T. ) ;
#182720=DIRECTION ( 'NONE',  ( 0.000000000000000000, 0.000000000000000000, 1.000000000000000000 ) ) ;
#182751=CIRCLE ( 'NONE', #195235, 0.1000000000000002554 ) ;
#182774=CARTESIAN_POINT ( 'NONE',  ( -5.900000000000002132, -11.34999999999999964, 14.00000000000000178 ) ) ;
#182784=LINE ( 'NONE', #21157, #20299 ) ;
#182791=DIRECTION ( 'NONE',  ( 0.000000000000000000, -1.000000000000000000, 0.000000000000000000 ) ) ;
#182830=AXIS2_PLACEMENT_3D ( 'NONE', #163106, #242613, #243899 ) ;
#182838=DIRECTION ( 'NONE',  ( 0.000000000000000000, 0.9856811345164832039, 0.1686199900910280158 ) ) ;
#182926=CIRCLE ( 'NONE', #70520, 0.2000000000000005107 ) ;
#182948=ORIENTED_EDGE ( 'NONE', *, *, #77344, .F. ) ;
#182957=ORIENTED_EDGE ( 'NONE', *, *, #179314, .T. ) ;
#182961=CARTESIAN_POINT ( 'NONE',  ( -18.79999999999999716, 1.149999999999999911, -15.00000000000000000 ) ) ;
#182963=ORIENTED_EDGE ( 'NONE', *, *, #176025, .F. ) ;
#182977=CARTESIAN_POINT ( 'NONE',  ( -13.40000000000000213, -11.65000000000000036, 15.00000000000000355 ) ) ;
#182986=CARTESIAN_POINT ( 'NONE',  ( 19.93974701750897438, 4.631764625248131928, 22.00000000173902137 ) ) ;
#182992=AXIS2_PLACEMENT_3D ( 'NONE', #172788, #64971, #46684 ) ;
#183024=AXIS2_PLACEMENT_3D ( 'NONE', #169438, #112005, #191555 ) ;
#183041=ORIENTED_EDGE ( 'NONE', *, *, #221498, .T. ) ;
#183088=AXIS2_PLACEMENT_3D ( 'NONE', #90421, #154314, #228681 ) ;
#183092=PLANE ( 'NONE',  #229641 ) ;
#183170=CIRCLE ( 'NONE', #70763, 0.09999999999999939493 ) ;
#183176=ORIENTED_EDGE ( 'NONE', *, *, #123320, .T. ) ;
#183231=DIRECTION ( 'NONE',  ( 0.000000000000000000, 0.000000000000000000, 1.000000000000000000 ) ) ;
#183244=EDGE_LOOP ( 'NONE', ( #168018, #251165, #119652, #244929 ) ) ;
#183254=ORIENTED_EDGE ( 'NONE', *, *, #228993, .F. ) ;
#183262=CIRCLE ( 'NONE', #195757, 0.09999999999999990841 ) ;
#183263=CIRCLE ( 'NONE', #58331, 0.1000000000000002554 ) ;
#183312=DIRECTION ( 'NONE',  ( -0.000000000000000000, 1.000000000000000000, 0.000000000000000000 ) ) ;
#183340=FILL_AREA_STYLE ('',( #103763 ) ) ;
#183434=DIRECTION ( 'NONE',  ( 0.000000000000000000, -0.1686199900910312910, 0.9856811345164826488 ) ) ;
#183435=ORIENTED_EDGE ( 'NONE', *, *, #3449, .F. ) ;
#183471=CARTESIAN_POINT ( 'NONE',  ( 20.90000000000000213, 11.59795743183152972, -1.899104650876408451 ) ) ;
#183555=DIRECTION ( 'NONE',  ( -0.000000000000000000, -0.000000000000000000, -1.000000000000000000 ) ) ;
#183564=FACE_OUTER_BOUND ( 'NONE', #77125, .T. ) ;
#183619=CARTESIAN_POINT ( 'NONE',  ( 13.40000000000000036, -8.250000000000003553, 17.60000000000000497 ) ) ;
#183620=DIRECTION ( 'NONE',  ( 0.000000000000000000, 0.000000000000000000, -1.000000000000000000 ) ) ;
#183666=CYLINDRICAL_SURFACE ( 'NONE', #33599, 0.09999999999999990841 ) ;
#183679=ORIENTED_EDGE ( 'NONE', *, *, #152429, .F. ) ;
#183703=DIRECTION ( 'NONE',  ( 0.000000000000000000, 0.000000000000000000, 1.000000000000000000 ) ) ;
#183752=EDGE_CURVE ( 'NONE', #156184, #82535, #45674, .T. ) ;
#183764=EDGE_CURVE ( 'NONE', #14083, #98899, #108222, .T. ) ;
#183809=CYLINDRICAL_SURFACE ( 'NONE', #60178, 11.75000000000000000 ) ;
#183812=CARTESIAN_POINT ( 'NONE',  ( 20.00000000000000711, 4.527376849368447864, 21.95857864376269220 ) ) ;
#183815=DIRECTION ( 'NONE',  ( 0.000000000000000000, 0.1335171055202867274, 0.9910465087640866200 ) ) ;
#183834=VERTEX_POINT ( 'NONE', #63958 ) ;
#183871=AXIS2_PLACEMENT_3D ( 'NONE', #233972, #59154, #252246 ) ;
#183890=ORIENTED_EDGE ( 'NONE', *, *, #24924, .T. ) ;
#183903=DIRECTION ( 'NONE',  ( -1.000000000000000000, -0.000000000000000000, 0.000000000000000000 ) ) ;
#183925=DIRECTION ( 'NONE',  ( 1.000000000000000000, -0.000000000000000000, -0.000000000000000000 ) ) ;
#183936=EDGE_CURVE ( 'NONE', #126, #75809, #200774, .T. ) ;
#183939=ORIENTED_EDGE ( 'NONE', *, *, #127158, .T. ) ;
#183946=ORIENTED_EDGE ( 'NONE', *, *, #165471, .T. ) ;
#183959=CIRCLE ( 'NONE', #175590, 0.09999999999999939493 ) ;
#183972=DIRECTION ( 'NONE',  ( 0.000000000000000000, 1.000000000000000000, 0.000000000000000000 ) ) ;
#183981=CARTESIAN_POINT ( 'NONE',  ( -22.94999999999999929, 1.800000000000000044, -11.61130914238355771 ) ) ;
#183985=CARTESIAN_POINT ( 'NONE',  ( 19.90000000000000924, 11.61130914238355771, 21.90000000000000213 ) ) ;
#183997=AXIS2_PLACEMENT_3D ( 'NONE', #243055, #25323, #20173 ) ;
#184048=VECTOR ( 'NONE', #218745, 1000.000000000000000 ) ;
#184049=DIRECTION ( 'NONE',  ( 0.000000000000000000, 0.000000000000000000, -1.000000000000000000 ) ) ;
#184079=AXIS2_PLACEMENT_3D ( 'NONE', #100976, #161013, #4483 ) ;
#184099=ORIENTED_EDGE ( 'NONE', *, *, #67939, .F. ) ;
#184133=DIRECTION ( 'NONE',  ( 0.000000000000000000, 0.000000000000000000, -1.000000000000000000 ) ) ;
#184142=CARTESIAN_POINT ( 'NONE',  ( -20.01715728752537871, 5.586869315528661062, 16.41686199900910736 ) ) ;
#184160=VECTOR ( 'NONE', #214228, 1000.000000000000000 ) ;
#184167=ORIENTED_EDGE ( 'NONE', *, *, #133631, .T. ) ;
#184217=EDGE_LOOP ( 'NONE', ( #68520, #58269, #243637, #92420 ) ) ;
#184263=DIRECTION ( 'NONE',  ( 0.000000000000000000, 0.1618390714546044939, 0.9868171638914228216 ) ) ;
#184295=VERTEX_POINT ( 'NONE', #116571 ) ;
#184321=DIRECTION ( 'NONE',  ( 1.000000000000000000, 0.000000000000000000, 0.000000000000000000 ) ) ;
#184329=EDGE_LOOP ( 'NONE', ( #88922, #127807, #62251, #45314 ) ) ;
#184338=AXIS2_PLACEMENT_3D ( 'NONE', #214608, #15144, #193776 ) ;
#184366=DIRECTION ( 'NONE',  ( 0.000000000000000000, 1.000000000000000000, 0.000000000000000000 ) ) ;
#184384=EDGE_CURVE ( 'NONE', #56204, #46280, #37062, .T. ) ;
#184407=DIRECTION ( 'NONE',  ( -0.000000000000000000, 1.000000000000000000, -0.000000000000000000 ) ) ;
#184411=AXIS2_PLACEMENT_3D ( 'NONE', #32703, #252977, #112215 ) ;
#184414=CARTESIAN_POINT ( 'NONE',  ( 0.000000000000000000, -8.350000000000004974, 32.89999999999999858 ) ) ;
#184432=AXIS2_PLACEMENT_3D ( 'NONE', #69056, #208565, #45628 ) ;
#184439=CARTESIAN_POINT ( 'NONE',  ( 5.999999999999995559, -11.75000000000000000, 10.10000000000000142 ) ) ;
#184443=CARTESIAN_POINT ( 'NONE',  ( -21.00000000000000000, 0.000000000000000000, 0.000000000000000000 ) ) ;
#184465=CARTESIAN_POINT ( 'NONE',  ( 18.69999999999999929, -10.64999999999999325, 33.00000000000000000 ) ) ;
#184468=VECTOR ( 'NONE', #6722, 1000.000000000000000 ) ;
#184495=CARTESIAN_POINT ( 'NONE',  ( 22.20000000000000284, 10.21702379168713115, -11.24211197275198160 ) ) ;
#184502=VECTOR ( 'NONE', #605, 1000.000000000000000 ) ;
#184511=FACE_OUTER_BOUND ( 'NONE', #117280, .T. ) ;
#184512=CIRCLE ( 'NONE', #109502, 0.09999999999999939493 ) ;
#184546=CARTESIAN_POINT ( 'NONE',  ( 18.69999999999999929, -8.350000000000004974, 10.52591260281975138 ) ) ;
#184563=VECTOR ( 'NONE', #197377, 1000.000000000000000 ) ;
#184582=DIRECTION ( 'NONE',  ( 0.000000000000000000, 0.000000000000000000, 1.000000000000000000 ) ) ;
#184596=DIRECTION ( 'NONE',  ( 0.000000000000000000, 0.000000000000000000, 1.000000000000000000 ) ) ;
#184603=ORIENTED_EDGE ( 'NONE', *, *, #224314, .T. ) ;
#184644=CIRCLE ( 'NONE', #197112, 4.041421356237310469 ) ;
#184709=CARTESIAN_POINT ( 'NONE',  ( 22.10000000000000142, -11.65000000000000036, 11.99999999999999645 ) ) ;
#184741=VECTOR ( 'NONE', #117027, 1000.000000000000000 ) ;
#184776=VERTEX_POINT ( 'NONE', #75855 ) ;
#184796=ORIENTED_EDGE ( 'NONE', *, *, #63365, .F. ) ;
#184818=VERTEX_POINT ( 'NONE', #237505 ) ;
#184901=CYLINDRICAL_SURFACE ( 'NONE', #199340, 2.600000000000001421 ) ;
#184935=FACE_OUTER_BOUND ( 'NONE', #197146, .T. ) ;
#184940=CARTESIAN_POINT ( 'NONE',  ( -6.000000000000002665, -11.65000000000000036, 14.00000000000000178 ) ) ;
#185007=EDGE_LOOP ( 'NONE', ( #185649, #207033, #200412, #209666 ) ) ;
#185014=ORIENTED_EDGE ( 'NONE', *, *, #84864, .T. ) ;
#185045=ORIENTED_EDGE ( 'NONE', *, *, #145146, .F. ) ;
#185093=TOROIDAL_SURFACE ( 'NONE', #159582, 11.65000000000000036, 0.1000000000000000056 ) ;
#185157=AXIS2_PLACEMENT_3D ( 'NONE', #140626, #162782, #183620 ) ;
#185207=FACE_OUTER_BOUND ( 'NONE', #55165, .T. ) ;
#185213=DIRECTION ( 'NONE',  ( 1.000000000000000000, -0.000000000000000000, -0.000000000000000000 ) ) ;
#185275=DIRECTION ( 'NONE',  ( 1.000000000000000000, -0.000000000000000000, -0.000000000000000000 ) ) ;
#185283=DIRECTION ( 'NONE',  ( 0.000000000000000000, 0.000000000000000000, -1.000000000000000000 ) ) ;
#185316=DIRECTION ( 'NONE',  ( 0.000000000000000000, 0.000000000000000000, -1.000000000000000000 ) ) ;
#185320=DIRECTION ( 'NONE',  ( 0.000000000000000000, 0.000000000000000000, -1.000000000000000000 ) ) ;
#185433=CARTESIAN_POINT ( 'NONE',  ( 18.79999999999999716, -1.885425182446133885, -11.49641995933507843 ) ) ;
#185445=VECTOR ( 'NONE', #141256, 1000.000000000000000 ) ;
#185533=EDGE_CURVE ( 'NONE', #223778, #217337, #126859, .T. ) ;
#185536=CARTESIAN_POINT ( 'NONE',  ( 19.90000000000000568, 1.350000000000000089, 16.60000000000000142 ) ) ;
#185542=CARTESIAN_POINT ( 'NONE',  ( 19.99016485861948667, 4.635725510443823971, 21.97684634237453594 ) ) ;
#185545=LINE ( 'NONE', #130372, #113781 ) ;
#185577=DIRECTION ( 'NONE',  ( 0.000000000000000000, 0.000000000000000000, -1.000000000000000000 ) ) ;
#185592=ORIENTED_EDGE ( 'NONE', *, *, #173156, .F. ) ;
#185626=CIRCLE ( 'NONE', #64801, 0.1000000000000028644 ) ;
#185630=ORIENTED_EDGE ( 'NONE', *, *, #26813, .F. ) ;
#185649=ORIENTED_EDGE ( 'NONE', *, *, #189016, .T. ) ;
#185689=EDGE_CURVE ( 'NONE', #109487, #1729, #197573, .T. ) ;
#185759=CARTESIAN_POINT ( 'NONE',  ( -20.90000000000000213, 11.49641995933507843, 1.885425182446133885 ) ) ;
#185784=AXIS2_PLACEMENT_3D ( 'NONE', #27616, #228355, #207519 ) ;
#185786=AXIS2_PLACEMENT_3D ( 'NONE', #180950, #140516, #200507 ) ;
#185793=CARTESIAN_POINT ( 'NONE',  ( -18.69999999999999929, -10.63400887967554986, 6.002871413764276909 ) ) ;
#185794=DIRECTION ( 'NONE',  ( -1.000000000000000000, 0.000000000000000000, 0.000000000000000000 ) ) ;
#185833=AXIS2_PLACEMENT_3D ( 'NONE', #187405, #110415, #53003 ) ;
#185858=ORIENTED_EDGE ( 'NONE', *, *, #125912, .T. ) ;
#185867=FACE_BOUND ( 'NONE', #225943, .T. ) ;
#185870=ORIENTED_EDGE ( 'NONE', *, *, #167281, .F. ) ;
#185991=ORIENTED_EDGE ( 'NONE', *, *, #10294, .T. ) ;
#186018=DIRECTION ( 'NONE',  ( 0.000000000000000000, 0.000000000000000000, 1.000000000000000000 ) ) ;
#186020=AXIS2_PLACEMENT_3D ( 'NONE', #84361, #163966, #25734 ) ;
#186049=LINE ( 'NONE', #204306, #241331 ) ;
#186088=CARTESIAN_POINT ( 'NONE',  ( 6.099999999999998757, -11.65000000000000036, 10.10000000000000142 ) ) ;
#186110=CARTESIAN_POINT ( 'NONE',  ( 13.40000000000000036, -11.75000000000000000, 12.30000000000000426 ) ) ;
#186121=CARTESIAN_POINT ( 'NONE',  ( 18.69999999999998153, 7.900000000000000355, -1.212568896937008089 ) ) ;
#186137=CARTESIAN_POINT ( 'NONE',  ( -22.19999999999999929, -11.65000000000000036, 28.70000000000000284 ) ) ;
#186182=AXIS2_PLACEMENT_3D ( 'NONE', #97381, #102514, #118275 ) ;
#186198=DIRECTION ( 'NONE',  ( 1.000000000000000000, 0.000000000000000000, 0.000000000000000000 ) ) ;
#186201=EDGE_LOOP ( 'NONE', ( #34843, #256343, #237134, #131021 ) ) ;
#186207=VERTEX_POINT ( 'NONE', #4061 ) ;
#186250=ADVANCED_FACE ( 'NONE', ( #146137 ), #44492, .F. ) ;
#186255=LINE ( 'NONE', #29773, #121741 ) ;
#186272=FACE_OUTER_BOUND ( 'NONE', #63226, .T. ) ;
#186275=AXIS2_PLACEMENT_3D ( 'NONE', #106693, #66309, #225358 ) ;
#186284=CARTESIAN_POINT ( 'NONE',  ( 0.000000000000000000, -10.64999999999999325, 32.89999999999999858 ) ) ;
#186295=DIRECTION ( 'NONE',  ( -1.284434275755705296E-16, 0.7071067811865471286, -0.7071067811865479058 ) ) ;
#186300=CARTESIAN_POINT ( 'NONE',  ( -18.79999999999999716, 4.611773100472912112, 22.11686199900910665 ) ) ;
#186327=EDGE_CURVE ( 'NONE', #109487, #102722, #226995, .T. ) ;
#186410=CONICAL_SURFACE ( 'NONE', #74003, 4.000000000000000000, 0.7853981633974489451 ) ;
#186433=DIRECTION ( 'NONE',  ( 0.000000000000000000, 0.000000000000000000, -1.000000000000000000 ) ) ;
#186442=CARTESIAN_POINT ( 'NONE',  ( -18.79999999999999716, -1.467286812112899463, 28.00000000000000000 ) ) ;
#186447=EDGE_CURVE ( 'NONE', #150252, #51689, #210447, .T. ) ;
#186500=CARTESIAN_POINT ( 'NONE',  ( -22.94999999999999929, 0.000000000000000000, 0.000000000000000000 ) ) ;
#186568=ORIENTED_EDGE ( 'NONE', *, *, #188393, .T. ) ;
#186571=DIRECTION ( 'NONE',  ( -1.000000000000000000, 0.000000000000000000, 0.000000000000000000 ) ) ;
#186592=AXIS2_PLACEMENT_3D ( 'NONE', #253207, #88985, #131982 ) ;
#186603=AXIS2_PLACEMENT_3D ( 'NONE', #115613, #193881, #218541 ) ;
#186662=AXIS2_PLACEMENT_3D ( 'NONE', #242777, #82398, #202381 ) ;
#186667=CIRCLE ( 'NONE', #37013, 0.2000000000000005107 ) ;
#186735=CARTESIAN_POINT ( 'NONE',  ( 18.69999999999999929, 3.362550747017869490, 28.82623795144604983 ) ) ;
#186744=ORIENTED_EDGE ( 'NONE', *, *, #180645, .F. ) ;
#186748=DIRECTION ( 'NONE',  ( 1.000000000000000000, 0.000000000000000000, 0.000000000000000000 ) ) ;
#186764=VERTEX_POINT ( 'NONE', #209664 ) ;
#186779=AXIS2_PLACEMENT_3D ( 'NONE', #22399, #242698, #224418 ) ;
#186797=CARTESIAN_POINT ( 'NONE',  ( 18.59999999999999787, -10.84999999999999076, 31.59999999999999787 ) ) ;
#186800=EDGE_LOOP ( 'NONE', ( #105355, #98946, #238332, #1687 ) ) ;
#186819=ADVANCED_FACE ( 'NONE', ( #171861 ), #65340, .T. ) ;
#186845=VECTOR ( 'NONE', #98282, 1000.000000000000000 ) ;
#186909=EDGE_LOOP ( 'NONE', ( #17413, #148509, #39504, #188681 ) ) ;
#186911=EDGE_CURVE ( 'NONE', #8100, #156872, #17867, .T. ) ;
#186935=DIRECTION ( 'NONE',  ( 0.000000000000000000, 0.000000000000000000, -1.000000000000000000 ) ) ;
#186943=DIRECTION ( 'NONE',  ( 0.000000000000000000, 1.000000000000000000, -0.000000000000000000 ) ) ;
#186944=CARTESIAN_POINT ( 'NONE',  ( -18.69999999999999929, -11.65000000000000036, 0.000000000000000000 ) ) ;
#186958=DIRECTION ( 'NONE',  ( 0.000000000000000000, 1.000000000000000000, 0.000000000000000000 ) ) ;
#186969=ADVANCED_FACE ( 'NONE', ( #180815 ), #73764, .T. ) ;
#186972=CARTESIAN_POINT ( 'NONE',  ( -18.79999999999999716, -10.84999999999999076, 32.89999999999999858 ) ) ;
#187034=VERTEX_POINT ( 'NONE', #6001 ) ;
#187047=ORIENTED_EDGE ( 'NONE', *, *, #145094, .T. ) ;
#187078=ADVANCED_FACE ( 'NONE', ( #7295 ), #166410, .T. ) ;
#187115=SPHERICAL_SURFACE ( 'NONE', #248143, 0.1000000000000000056 ) ;
#187122=EDGE_LOOP ( 'NONE', ( #226123, #53032, #137367 ) ) ;
#187152=LINE ( 'NONE', #166320, #81733 ) ;
#187188=LINE ( 'NONE', #151919, #141461 ) ;
#187212=ORIENTED_EDGE ( 'NONE', *, *, #52789, .T. ) ;
#187214=ORIENTED_EDGE ( 'NONE', *, *, #214398, .F. ) ;
#187219=CARTESIAN_POINT ( 'NONE',  ( -20.90000000000000213, -1.885425182446133885, -11.49641995933507843 ) ) ;
#187231=ADVANCED_FACE ( 'NONE', ( #225866 ), #123101, .T. ) ;
#187238=TOROIDAL_SURFACE ( 'NONE', #145510, 4.041421356237310469, 0.1000000000000000056 ) ;
#187275=DIRECTION ( 'NONE',  ( -0.000000000000000000, -0.9910465087640860649, -0.1335171055202901413 ) ) ;
#187276=CARTESIAN_POINT ( 'NONE',  ( -20.90000000000000213, -1.899104650876408451, -11.59795743183152972 ) ) ;
#187283=TOROIDAL_SURFACE ( 'NONE', #228964, 0.2000000000000000111, 0.1000000000000000056 ) ;
#187284=CARTESIAN_POINT ( 'NONE',  ( -18.79999999999999716, 5.488301202077013663, 16.40000000000000213 ) ) ;
#187332=CARTESIAN_POINT ( 'NONE',  ( -18.79999999999999716, -11.65000000000000036, 30.09999999999999787 ) ) ;
#187344=DIRECTION ( 'NONE',  ( 1.000000000000000000, -0.000000000000000000, -0.000000000000000000 ) ) ;
#187405=CARTESIAN_POINT ( 'NONE',  ( -18.79999999999999716, 10.31653824539117714, -11.82383137372478110 ) ) ;
#187427=ORIENTED_EDGE ( 'NONE', *, *, #86847, .F. ) ;
#187450=FACE_OUTER_BOUND ( 'NONE', #216584, .T. ) ;
#187452=AXIS2_PLACEMENT_3D ( 'NONE', #141346, #6966, #104751 ) ;
#187453=DIRECTION ( 'NONE',  ( -0.000000000000000000, 1.000000000000000000, -0.000000000000000000 ) ) ;
#187502=DIRECTION ( 'NONE',  ( 0.000000000000000000, -0.4856429311786357728, -0.8741572761215358200 ) ) ;
#187515=EDGE_CURVE ( 'NONE', #246378, #254139, #148211, .T. ) ;
#187622=VECTOR ( 'NONE', #179617, 1000.000000000000000 ) ;
#187627=CARTESIAN_POINT ( 'NONE',  ( -18.79999999999999716, 1.149999999999999911, 21.90000000000000213 ) ) ;
#187674=DIRECTION ( 'NONE',  ( 0.000000000000000000, 0.000000000000000000, -1.000000000000000000 ) ) ;
#187767=DIRECTION ( 'NONE',  ( 0.000000000000000000, 0.000000000000000000, -1.000000000000000000 ) ) ;
#187784=ORIENTED_EDGE ( 'NONE', *, *, #219413, .T. ) ;
#187816=CARTESIAN_POINT ( 'NONE',  ( -5.900000000000003020, -11.65000000000000036, 9.900000000000002132 ) ) ;
#187876=DIRECTION ( 'NONE',  ( 1.476360405086644309E-16, -1.000000000000000000, -0.000000000000000000 ) ) ;
#187954=CARTESIAN_POINT ( 'NONE',  ( -19.89999999999999858, 1.350000000000000089, 16.60000000000000142 ) ) ;
#187979=EDGE_CURVE ( 'NONE', #94336, #181665, #180868, .T. ) ;
#187987=ORIENTED_EDGE ( 'NONE', *, *, #202572, .T. ) ;
#187989=CIRCLE ( 'NONE', #208830, 0.09999999999999939493 ) ;
#187996=ORIENTED_EDGE ( 'NONE', *, *, #86685, .T. ) ;
#188035=ORIENTED_EDGE ( 'NONE', *, *, #20023, .T. ) ;
#188052=FACE_OUTER_BOUND ( 'NONE', #52966, .T. ) ;
#188056=ORIENTED_EDGE ( 'NONE', *, *, #95903, .T. ) ;
#188064=DIRECTION ( 'NONE',  ( -0.000000000000000000, 1.000000000000000000, -0.000000000000000000 ) ) ;
#188066=CARTESIAN_POINT ( 'NONE',  ( -0.8999999999999993561, -11.65000000000000036, 26.00000000000000355 ) ) ;
#188142=ORIENTED_EDGE ( 'NONE', *, *, #55320, .T. ) ;
#188244=DIRECTION ( 'NONE',  ( -1.000000000000000000, 0.000000000000000000, -0.000000000000000000 ) ) ;
#188246=EDGE_CURVE ( 'NONE', #137467, #193899, #27813, .T. ) ;
#188311=VECTOR ( 'NONE', #195628, 1000.000000000000000 ) ;
#188314=AXIS2_PLACEMENT_3D ( 'NONE', #230560, #210991, #192714 ) ;
#188390=EDGE_LOOP ( 'NONE', ( #48429, #110677, #159549, #133032 ) ) ;
#188393=EDGE_CURVE ( 'NONE', #136731, #160911, #123154, .T. ) ;
#188417=VERTEX_POINT ( 'NONE', #124444 ) ;
#188426=DIRECTION ( 'NONE',  ( 0.000000000000000000, -1.000000000000000000, 0.000000000000000000 ) ) ;
#188437=AXIS2_PLACEMENT_3D ( 'NONE', #188516, #245935, #244632 ) ;
#188493=TOROIDAL_SURFACE ( 'NONE', #142680, 2.699999999999999734, 0.1000000000000000056 ) ;
#188512=DIRECTION ( 'NONE',  ( -0.000000000000000000, 1.000000000000000000, -0.000000000000000000 ) ) ;
#188516=CARTESIAN_POINT ( 'NONE',  ( -22.94999999999999929, 3.461118860469513336, 28.84309995045515507 ) ) ;
#188530=CARTESIAN_POINT ( 'NONE',  ( -20.90000000000000213, -1.885425182446133885, -11.49641995933507843 ) ) ;
#188531=CARTESIAN_POINT ( 'NONE',  ( 20.90000000000000213, -11.65000000000000036, 0.000000000000000000 ) ) ;
#188543=CARTESIAN_POINT ( 'NONE',  ( 21.00000000000000000, 7.800000000000000711, -1.212568896937008089 ) ) ;
#188620=ADVANCED_FACE ( 'NONE', ( #154321 ), #52590, .F. ) ;
#188628=EDGE_LOOP ( 'NONE', ( #247470, #90062, #65493, #150303 ) ) ;
#188657=ORIENTED_EDGE ( 'NONE', *, *, #47982, .T. ) ;
#188679=ORIENTED_EDGE ( 'NONE', *, *, #48158, .F. ) ;
#188681=ORIENTED_EDGE ( 'NONE', *, *, #172772, .T. ) ;
#188682=DIRECTION ( 'NONE',  ( 0.000000000000000000, 1.000000000000000000, 0.000000000000000000 ) ) ;
#188691=DIRECTION ( 'NONE',  ( 0.000000000000000000, -1.000000000000000000, 0.000000000000000000 ) ) ;
#188698=AXIS2_PLACEMENT_3D ( 'NONE', #97203, #178094, #137641 ) ;
#188700=TOROIDAL_SURFACE ( 'NONE', #192818, 0.2000000000000000111, 0.1000000000000000056 ) ;
#188714=VECTOR ( 'NONE', #110350, 1000.000000000000000 ) ;
#188735=ORIENTED_EDGE ( 'NONE', *, *, #132501, .T. ) ;
#188819=DIRECTION ( 'NONE',  ( 1.000000000000000000, 0.000000000000000000, 0.000000000000000000 ) ) ;
#188863=AXIS2_PLACEMENT_3D ( 'NONE', #29029, #26431, #224605 ) ;
#188867=AXIS2_PLACEMENT_3D ( 'NONE', #158023, #176280, #133277 ) ;
#188883=CARTESIAN_POINT ( 'NONE',  ( 18.79999999999999361, -11.65000000000000036, -15.00000000000000000 ) ) ;
#188887=DIRECTION ( 'NONE',  ( 0.000000000000000000, 0.000000000000000000, -1.000000000000000000 ) ) ;
#188894=DIRECTION ( 'NONE',  ( -0.000000000000000000, -0.000000000000000000, -1.000000000000000000 ) ) ;
#188929=VERTEX_POINT ( 'NONE', #90115 ) ;
#188965=CARTESIAN_POINT ( 'NONE',  ( -18.79999999999999716, 8.000000000000000000, 1.212568896937007867 ) ) ;
#188975=ORIENTED_EDGE ( 'NONE', *, *, #73680, .T. ) ;
#189003=CARTESIAN_POINT ( 'NONE',  ( -21.00000000000000000, 6.742993295648862961, 9.658650260582458458 ) ) ;
#189011=DIRECTION ( 'NONE',  ( -1.000000000000000000, -0.000000000000000000, -0.000000000000000000 ) ) ;
#189016=EDGE_CURVE ( 'NONE', #41107, #211171, #195685, .T. ) ;
#189021=CARTESIAN_POINT ( 'NONE',  ( 21.00000000000000000, 0.000000000000000000, 0.000000000000000000 ) ) ;
#189022=ORIENTED_EDGE ( 'NONE', *, *, #69908, .F. ) ;
#189045=AXIS2_PLACEMENT_3D ( 'NONE', #149447, #167731, #166457 ) ;
#189059=CARTESIAN_POINT ( 'NONE',  ( -22.94999999999999929, 3.461118860469513336, 28.84309995045515507 ) ) ;
#189060=DIRECTION ( 'NONE',  ( 1.000000000000000000, -0.000000000000000000, -0.000000000000000000 ) ) ;
#189152=CARTESIAN_POINT ( 'NONE',  ( 21.10000000000000142, 6.223900101154157483, 12.00000000000000000 ) ) ;
#189162=EDGE_LOOP ( 'NONE', ( #210377, #226889, #14170, #81958 ) ) ;
#189172=VECTOR ( 'NONE', #129471, 1000.000000000000000 ) ;
#189216=CYLINDRICAL_SURFACE ( 'NONE', #131467, 2.600000000000001421 ) ;
#189251=CARTESIAN_POINT ( 'NONE',  ( -18.79999999999999716, -11.75000000000000000, -15.00000000000000000 ) ) ;
#189327=ORIENTED_EDGE ( 'NONE', *, *, #50018, .T. ) ;
#189355=DIRECTION ( 'NONE',  ( 0.000000000000000000, 0.000000000000000000, -1.000000000000000000 ) ) ;
#189397=AXIS2_PLACEMENT_3D ( 'NONE', #75476, #110721, #233266 ) ;
#189450=VECTOR ( 'NONE', #181404, 1000.000000000000000 ) ;
#189526=EDGE_CURVE ( 'NONE', #127870, #221991, #38853, .T. ) ;
#189532=CYLINDRICAL_SURFACE ( 'NONE', #213715, 0.09999999999999939493 ) ;
#189578=( BOUNDED_CURVE ( )  B_SPLINE_CURVE ( 3, ( #81292, #141302, #177878, #180432 ),
 .UNSPECIFIED., .F., .F. ) 
 B_SPLINE_CURVE_WITH_KNOTS ( ( 4, 4 ),
 ( 4.712388980384690562, 6.283185307179586232 ),
 .UNSPECIFIED. ) 
 CURVE ( )  GEOMETRIC_REPRESENTATION_ITEM ( )  RATIONAL_B_SPLINE_CURVE ( ( 1.000000000000000000, 0.8047378541243652705, 0.8047378541243652705, 1.000000000000000000 ) ) 
 REPRESENTATION_ITEM ( '' )  );
#189583=VERTEX_POINT ( 'NONE', #97494 ) ;
#189638=FACE_OUTER_BOUND ( 'NONE', #33461, .T. ) ;
#189677=DIRECTION ( 'NONE',  ( 0.000000000000000000, 1.000000000000000000, 1.224646799147353207E-16 ) ) ;
#189731=AXIS2_PLACEMENT_3D ( 'NONE', #27570, #126626, #66662 ) ;
#189737=EDGE_CURVE ( 'NONE', #178041, #76531, #107037, .T. ) ;
#189812=ADVANCED_FACE ( 'NONE', ( #136002 ), #236407, .F. ) ;
#189815=FACE_OUTER_BOUND ( 'NONE', #14424, .T. ) ;
#189888=DIRECTION ( 'NONE',  ( -0.000000000000000000, 0.4856429311786307212, 0.8741572761215384846 ) ) ;
#189894=CARTESIAN_POINT ( 'NONE',  ( -21.00000000000000000, 0.000000000000000000, 0.000000000000000000 ) ) ;
#189929=DIRECTION ( 'NONE',  ( -1.000000000000000000, -3.469446951953635646E-14, 0.000000000000000000 ) ) ;
#189932=VERTEX_POINT ( 'NONE', #201131 ) ;
#189944=ORIENTED_EDGE ( 'NONE', *, *, #144570, .T. ) ;
#189972=DIRECTION ( 'NONE',  ( -0.000000000000000000, -0.1335171055202901413, -0.9910465087640860649 ) ) ;
#189989=CIRCLE ( 'NONE', #239891, 0.1000000000000002554 ) ;
#190090=ADVANCED_FACE ( 'NONE', ( #68043 ), #28971, .F. ) ;
#190122=EDGE_CURVE ( 'NONE', #79286, #110943, #165512, .T. ) ;
#190169=VERTEX_POINT ( 'NONE', #236102 ) ;
#190192=LINE ( 'NONE', #228022, #36948 ) ;
#190211=CARTESIAN_POINT ( 'NONE',  ( 18.69999999999999929, 10.88519226655716565, -15.14794223642649840 ) ) ;
#190236=EDGE_CURVE ( 'NONE', #90690, #238394, #53060, .T. ) ;
#190254=DIRECTION ( 'NONE',  ( -1.000000000000000000, 0.000000000000000000, 0.000000000000000000 ) ) ;
#190300=ORIENTED_EDGE ( 'NONE', *, *, #214497, .F. ) ;
#190381=CARTESIAN_POINT ( 'NONE',  ( 20.90000000000000213, 0.000000000000000000, 0.000000000000000000 ) ) ;
#190421=DIRECTION ( 'NONE',  ( 0.000000000000000000, 0.000000000000000000, 1.000000000000000000 ) ) ;
#190434=CIRCLE ( 'NONE', #11339, 2.600000000000001421 ) ;
#190437=DIRECTION ( 'NONE',  ( -1.000000000000000000, 0.000000000000000000, -0.000000000000000000 ) ) ;
#190484=FACE_OUTER_BOUND ( 'NONE', #52491, .T. ) ;
#190493=ORIENTED_EDGE ( 'NONE', *, *, #251889, .F. ) ;
#190506=ADVANCED_FACE ( 'NONE', ( #134112 ), #203280, .T. ) ;
#190527=ORIENTED_EDGE ( 'NONE', *, *, #125913, .F. ) ;
#190533=CARTESIAN_POINT ( 'NONE',  ( 21.10000000000000142, 6.322468214605803993, 12.11686199900910488 ) ) ;
#190583=DIRECTION ( 'NONE',  ( 0.000000000000000000, 0.000000000000000000, 1.000000000000000000 ) ) ;
#190587=FACE_OUTER_BOUND ( 'NONE', #29303, .T. ) ;
#190645=CARTESIAN_POINT ( 'NONE',  ( 0.000000000000000000, 1.250000000000000000, 0.000000000000000000 ) ) ;
#190676=VERTEX_POINT ( 'NONE', #97534 ) ;
#190681=CARTESIAN_POINT ( 'NONE',  ( 18.59999999999999787, -9.849999999999942801, -15.00000000000002309 ) ) ;
#190683=DIRECTION ( 'NONE',  ( 1.000000000000000000, -0.000000000000000000, -0.000000000000000000 ) ) ;
#190722=ORIENTED_EDGE ( 'NONE', *, *, #152792, .T. ) ;
#190763=ORIENTED_EDGE ( 'NONE', *, *, #69982, .T. ) ;
#190789=VERTEX_POINT ( 'NONE', #165245 ) ;
#190881=VERTEX_POINT ( 'NONE', #170432 ) ;
#190891=EDGE_CURVE ( 'NONE', #12756, #129607, #99201, .T. ) ;
#190912=DIRECTION ( 'NONE',  ( -1.000000000000000000, -0.000000000000000000, 0.000000000000000000 ) ) ;
#191025=DIRECTION ( 'NONE',  ( 0.000000000000000000, 0.000000000000000000, -1.000000000000000000 ) ) ;
#191064=CIRCLE ( 'NONE', #132801, 0.09999999999999939493 ) ;
#191172=CIRCLE ( 'NONE', #145344, 0.09999999999999961697 ) ;
#191182=EDGE_CURVE ( 'NONE', #233025, #246137, #216106, .T. ) ;
#191204=EDGE_CURVE ( 'NONE', #206620, #169705, #200931, .T. ) ;
#191230=EDGE_CURVE ( 'NONE', #27940, #136731, #202218, .T. ) ;
#191248=AXIS2_PLACEMENT_3D ( 'NONE', #174967, #255683, #195788 ) ;
#191256=VECTOR ( 'NONE', #99449, 1000.000000000000114 ) ;
#191258=EDGE_CURVE ( 'NONE', #27940, #79153, #166082, .T. ) ;
#191274=AXIS2_PLACEMENT_3D ( 'NONE', #106804, #207219, #162963 ) ;
#191288=CARTESIAN_POINT ( 'NONE',  ( -22.19999999999999929, -11.65000000000000036, 12.09999999999999609 ) ) ;
#191292=LINE ( 'NONE', #53022, #85382 ) ;
#191347=ORIENTED_EDGE ( 'NONE', *, *, #202665, .T. ) ;
#191375=ORIENTED_EDGE ( 'NONE', *, *, #75607, .F. ) ;
#191418=DIRECTION ( 'NONE',  ( -1.000000000000000000, -0.000000000000000000, -0.000000000000000000 ) ) ;
#191442=DIRECTION ( 'NONE',  ( 0.000000000000000000, -1.000000000000000000, 0.000000000000000000 ) ) ;
#191455=CIRCLE ( 'NONE', #145603, 0.09999999999999993616 ) ;
#191516=DIRECTION ( 'NONE',  ( 1.000000000000000000, 0.000000000000000000, 0.000000000000000000 ) ) ;
#191535=CARTESIAN_POINT ( 'NONE',  ( 18.69999999999999929, -10.63400887967554986, 6.002871413764276909 ) ) ;
#191555=DIRECTION ( 'NONE',  ( 1.000000000000000000, 0.000000000000000000, 0.000000000000000000 ) ) ;
#191596=ORIENTED_EDGE ( 'NONE', *, *, #102875, .F. ) ;
#191710=ORIENTED_EDGE ( 'NONE', *, *, #83535, .T. ) ;
#191725=CARTESIAN_POINT ( 'NONE',  ( -0.8999999999999993561, -11.65000000000000036, 23.40000000000000568 ) ) ;
#191726=DIRECTION ( 'NONE',  ( 3.469446951953635015E-14, 0.000000000000000000, 1.000000000000000000 ) ) ;
#191743=CIRCLE ( 'NONE', #79243, 0.09999999999999939493 ) ;
#191759=CARTESIAN_POINT ( 'NONE',  ( -18.60000000000000142, -8.350000000000004974, 32.89999999999999858 ) ) ;
#191820=AXIS2_PLACEMENT_3D ( 'NONE', #115601, #158611, #178173 ) ;
#191829=DIRECTION ( 'NONE',  ( 0.000000000000000000, 0.000000000000000000, 1.000000000000000000 ) ) ;
#191858=AXIS2_PLACEMENT_3D ( 'NONE', #48662, #27860, #31711 ) ;
#191907=CARTESIAN_POINT ( 'NONE',  ( -18.79999999999999716, 5.488301202077012775, 16.40000000000000213 ) ) ;
#191933=ORIENTED_EDGE ( 'NONE', *, *, #135292, .F. ) ;
#191959=ORIENTED_EDGE ( 'NONE', *, *, #59360, .F. ) ;
#191989=CARTESIAN_POINT ( 'NONE',  ( -6.100000000000006750, -11.75000000000000000, 10.10000000000000142 ) ) ;
#192016=CARTESIAN_POINT ( 'NONE',  ( -21.00000000000000000, -0.04453801223857078301, 0.3305886640091971196 ) ) ;
#192025=FACE_OUTER_BOUND ( 'NONE', #106932, .T. ) ;
#192058=ADVANCED_FACE ( 'NONE', ( #67214 ), #24973, .T. ) ;
#192148=CIRCLE ( 'NONE', #225413, 0.1000000000000000472 ) ;
#192159=CARTESIAN_POINT ( 'NONE',  ( -6.000000000000002665, -11.34999999999999964, 13.90000000000000213 ) ) ;
#192176=VERTEX_POINT ( 'NONE', #136139 ) ;
#192186=ORIENTED_EDGE ( 'NONE', *, *, #236248, .F. ) ;
#192216=DIRECTION ( 'NONE',  ( 1.284434275755705789E-16, -0.7071067811865472397, -0.7071067811865479058 ) ) ;
#192223=DIRECTION ( 'NONE',  ( -1.000000000000000000, 0.000000000000000000, 0.000000000000000000 ) ) ;
#192275=DIRECTION ( 'NONE',  ( 0.000000000000000000, 0.9910465087640860649, 0.1335171055202901413 ) ) ;
#192317=SPHERICAL_SURFACE ( 'NONE', #130546, 0.1000000000000000056 ) ;
#192330=CIRCLE ( 'NONE', #79870, 0.09999999999999990841 ) ;
#192347=EDGE_LOOP ( 'NONE', ( #71027, #175843, #173541, #248131 ) ) ;
#192467=DIRECTION ( 'NONE',  ( -1.000000000000000000, 0.000000000000000000, 0.000000000000000000 ) ) ;
#192550=CIRCLE ( 'NONE', #163334, 0.09999999999999990841 ) ;
#192587=VECTOR ( 'NONE', #256423, 1000.000000000000000 ) ;
#192591=EDGE_LOOP ( 'NONE', ( #113336, #160089, #176153, #14547 ) ) ;
#192618=TOROIDAL_SURFACE ( 'NONE', #238396, 2.699999999999999734, 0.1000000000000000056 ) ;
#192691=CIRCLE ( 'NONE', #113572, 0.1000000000000028644 ) ;
#192714=DIRECTION ( 'NONE',  ( -1.000000000000000000, 0.000000000000000000, 0.000000000000000000 ) ) ;
#192721=DIRECTION ( 'NONE',  ( 0.000000000000000000, 0.9910465087640865089, -0.1335171055202864221 ) ) ;
#192735=EDGE_LOOP ( 'NONE', ( #138983, #58008, #36795, #41643 ) ) ;
#192778=CARTESIAN_POINT ( 'NONE',  ( 18.69999999999999574, -11.65000000000000036, 30.00000000000000000 ) ) ;
#192792=ORIENTED_EDGE ( 'NONE', *, *, #111579, .F. ) ;
#192804=DIRECTION ( 'NONE',  ( 0.000000000000000000, 0.000000000000000000, -1.000000000000000000 ) ) ;
#192818=AXIS2_PLACEMENT_3D ( 'NONE', #151674, #211623, #108658 ) ;
#192827=LINE ( 'NONE', #14204, #50580 ) ;
#192833=EDGE_LOOP ( 'NONE', ( #103363, #139037, #48537, #106710 ) ) ;
#192838=CIRCLE ( 'NONE', #176283, 0.09999999999999939493 ) ;
#192886=CARTESIAN_POINT ( 'NONE',  ( 18.79999999999999716, 6.726092018229619107, 9.512212474619550662 ) ) ;
#192900=VERTEX_POINT ( 'NONE', #20458 ) ;
#192923=ORIENTED_EDGE ( 'NONE', *, *, #6503, .T. ) ;
#192981=VECTOR ( 'NONE', #248988, 1000.000000000000000 ) ;
#193025=ORIENTED_EDGE ( 'NONE', *, *, #52572, .F. ) ;
#193054=DIRECTION ( 'NONE',  ( 1.000000000000000000, 0.000000000000000000, 0.000000000000000000 ) ) ;
#193055=DIRECTION ( 'NONE',  ( 1.000000000000000000, -0.000000000000000000, -0.000000000000000000 ) ) ;
#193111=DIRECTION ( 'NONE',  ( 0.000000000000000000, 0.9910465087640868420, -0.1335171055202844237 ) ) ;
#193129=CARTESIAN_POINT ( 'NONE',  ( -22.84999999999999787, 0.000000000000000000, 0.000000000000000000 ) ) ;
#193189=FACE_OUTER_BOUND ( 'NONE', #48069, .T. ) ;
#193230=CYLINDRICAL_SURFACE ( 'NONE', #14940, 0.09999999999999939493 ) ;
#193250=DIRECTION ( 'NONE',  ( 0.000000000000000000, 0.000000000000000000, -1.000000000000000000 ) ) ;
#193254=EDGE_CURVE ( 'NONE', #25377, #70370, #241425, .T. ) ;
#193274=LINE ( 'NONE', #118883, #170802 ) ;
#193313=EDGE_CURVE ( 'NONE', #62787, #235390, #166606, .T. ) ;
#193393=EDGE_LOOP ( 'NONE', ( #9039, #218221, #53754, #214210 ) ) ;
#193446=ADVANCED_FACE ( 'NONE', ( #169958 ), #129505, .F. ) ;
#193487=VERTEX_POINT ( 'NONE', #210334 ) ;
#193529=ORIENTED_EDGE ( 'NONE', *, *, #97871, .F. ) ;
#193541=AXIS2_PLACEMENT_3D ( 'NONE', #64938, #20708, #42822 ) ;
#193583=CARTESIAN_POINT ( 'NONE',  ( 18.79999999999999716, 1.800000000000000044, -11.61130914238355771 ) ) ;
#193602=CIRCLE ( 'NONE', #97711, 0.2000000000000005107 ) ;
#193668=CARTESIAN_POINT ( 'NONE',  ( 18.59999999999999787, -10.64999999999999325, 31.50000000000000000 ) ) ;
#193680=DIRECTION ( 'NONE',  ( -1.284434275755705296E-16, 0.7071067811865471286, 0.7071067811865479058 ) ) ;
#193683=ADVANCED_FACE ( 'NONE', ( #117637 ), #96004, .T. ) ;
#193697=AXIS2_PLACEMENT_3D ( 'NONE', #224678, #89023, #142569 ) ;
#193740=DIRECTION ( 'NONE',  ( -1.000000000000000000, 0.000000000000000000, 0.000000000000000000 ) ) ;
#193745=CARTESIAN_POINT ( 'NONE',  ( -18.59999999999999787, -11.65000000000000036, 30.09999999999999787 ) ) ;
#193750=CYLINDRICAL_SURFACE ( 'NONE', #244527, 0.09999999999999939493 ) ;
#193776=DIRECTION ( 'NONE',  ( 0.000000000000000000, 0.000000000000000000, -1.000000000000000000 ) ) ;
#193782=MECHANICAL_DESIGN_GEOMETRIC_PRESENTATION_REPRESENTATION('',(#235458),#252208);
#193818=CARTESIAN_POINT ( 'NONE',  ( -18.59999999999999787, -10.84999999999999076, 31.59999999999999787 ) ) ;
#193836=ADVANCED_FACE ( 'NONE', ( #1524 ), #54313, .T. ) ;
#193837=DIRECTION ( 'NONE',  ( 1.000000000000000000, 0.000000000000000000, 0.000000000000000000 ) ) ;
#193870=EDGE_LOOP ( 'NONE', ( #22108, #184099, #220492, #198022 ) ) ;
#193881=DIRECTION ( 'NONE',  ( -1.000000000000000000, 0.000000000000000000, 0.000000000000000000 ) ) ;
#193899=VERTEX_POINT ( 'NONE', #247852 ) ;
#193902=EDGE_CURVE ( 'NONE', #126, #208096, #91361, .T. ) ;
#193960=ORIENTED_EDGE ( 'NONE', *, *, #63365, .T. ) ;
#194008=CARTESIAN_POINT ( 'NONE',  ( -21.10000000000000142, 6.223900101154155706, 12.00000000000000178 ) ) ;
#194018=CIRCLE ( 'NONE', #98100, 4.000000000000000000 ) ;
#194029=ORIENTED_EDGE ( 'NONE', *, *, #108785, .F. ) ;
#194035=CIRCLE ( 'NONE', #252252, 0.09999999999999990841 ) ;
#194041=CARTESIAN_POINT ( 'NONE',  ( 18.79999999999999716, 2.524878688533307880, -16.24283924587617989 ) ) ;
#194049=DIRECTION ( 'NONE',  ( 0.000000000000000000, 0.9910465087640860649, 0.1335171055202901413 ) ) ;
#194070=FACE_OUTER_BOUND ( 'NONE', #90127, .T. ) ;
#194083=ORIENTED_EDGE ( 'NONE', *, *, #124177, .T. ) ;
#194097=CYLINDRICAL_SURFACE ( 'NONE', #198593, 0.1000000000000001443 ) ;
#194129=EDGE_CURVE ( 'NONE', #83776, #103483, #50386, .T. ) ;
#194131=DIRECTION ( 'NONE',  ( -1.000000000000000000, 0.000000000000000000, 0.000000000000000000 ) ) ;
#194144=ORIENTED_EDGE ( 'NONE', *, *, #224601, .T. ) ;
#194156=ORIENTED_EDGE ( 'NONE', *, *, #26293, .F. ) ;
#194195=DIRECTION ( 'NONE',  ( -1.000000000000000000, 0.000000000000000000, 0.000000000000000000 ) ) ;
#194216=VECTOR ( 'NONE', #183434, 1000.000000000000227 ) ;
#194265=DIRECTION ( 'NONE',  ( 0.000000000000000000, -0.1335171055202867274, -0.9910465087640866200 ) ) ;
#194299=CARTESIAN_POINT ( 'NONE',  ( 21.00000000000000000, -11.65000000000000036, 0.000000000000000000 ) ) ;
#194303=DIRECTION ( 'NONE',  ( -0.000000000000000000, 1.000000000000000000, -0.000000000000000000 ) ) ;
#194309=EDGE_CURVE ( 'NONE', #69570, #22186, #46484, .T. ) ;
#194354=DIRECTION ( 'NONE',  ( 0.000000000000000000, -1.000000000000000000, 0.000000000000000000 ) ) ;
#194417=VERTEX_POINT ( 'NONE', #34620 ) ;
#194439=EDGE_LOOP ( 'NONE', ( #146374, #187212, #35432 ) ) ;
#194444=CYLINDRICAL_SURFACE ( 'NONE', #115181, 0.1000000000000028644 ) ;
#194459=EDGE_CURVE ( 'NONE', #7521, #2147, #187989, .T. ) ;
#194477=AXIS2_PLACEMENT_3D ( 'NONE', #109588, #187876, #127890 ) ;
#194485=ORIENTED_EDGE ( 'NONE', *, *, #139886, .F. ) ;
#194516=EDGE_CURVE ( 'NONE', #29111, #166243, #163055, .T. ) ;
#194517=EDGE_LOOP ( 'NONE', ( #56509, #199083, #90945, #221836 ) ) ;
#194526=CARTESIAN_POINT ( 'NONE',  ( 18.59999999999999787, -11.65000000000000036, 30.09999999999999787 ) ) ;
#194544=ORIENTED_EDGE ( 'NONE', *, *, #34931, .F. ) ;
#194569=ORIENTED_EDGE ( 'NONE', *, *, #157054, .F. ) ;
#194608=CARTESIAN_POINT ( 'NONE',  ( -22.20000000000000284, 6.322468214605804882, 12.11686199900910310 ) ) ;
#194632=VERTEX_POINT ( 'NONE', #151006 ) ;
#194637=CARTESIAN_POINT ( 'NONE',  ( -19.95447128016622784, 5.488301201494659942, 16.50000000000000000 ) ) ;
#194668=VECTOR ( 'NONE', #167196, 1000.000000000000000 ) ;
#194711=ORIENTED_EDGE ( 'NONE', *, *, #183936, .T. ) ;
#194732=ORIENTED_EDGE ( 'NONE', *, *, #56458, .F. ) ;
#194763=AXIS2_PLACEMENT_3D ( 'NONE', #24594, #48927, #61121 ) ;
#194796=EDGE_LOOP ( 'NONE', ( #117909, #146793, #69588, #76465 ) ) ;
#194799=AXIS2_PLACEMENT_3D ( 'NONE', #193745, #93347, #209445 ) ;
#194810=EDGE_LOOP ( 'NONE', ( #157385, #129058 ) ) ;
#194888=EDGE_CURVE ( 'NONE', #215605, #219055, #45164, .T. ) ;
#194964=DIRECTION ( 'NONE',  ( -0.000000000000000000, 0.1686199900910312910, -0.9856811345164826488 ) ) ;
#194965=DIRECTION ( 'NONE',  ( 0.000000000000000000, 0.000000000000000000, -1.000000000000000000 ) ) ;
#195035=TOROIDAL_SURFACE ( 'NONE', #20242, 4.100000000000000533, 0.1000000000000000056 ) ;
#195040=EDGE_CURVE ( 'NONE', #152492, #209282, #250860, .T. ) ;
#195043=ORIENTED_EDGE ( 'NONE', *, *, #165912, .T. ) ;
#195052=CARTESIAN_POINT ( 'NONE',  ( 18.79999999999999716, 1.885425182446133885, -11.49641995933507843 ) ) ;
#195055=CARTESIAN_POINT ( 'NONE',  ( 20.89999999999999503, 8.000000000000000000, -1.212568896937008089 ) ) ;
#195070=EDGE_CURVE ( 'NONE', #247452, #66961, #150930, .T. ) ;
#195082=DIRECTION ( 'NONE',  ( -1.000000000000000000, 0.000000000000000000, 0.000000000000000000 ) ) ;
#195115=FACE_OUTER_BOUND ( 'NONE', #209509, .T. ) ;
#195138=CYLINDRICAL_SURFACE ( 'NONE', #248363, 0.09999999999999939493 ) ;
#195142=ORIENTED_EDGE ( 'NONE', *, *, #79475, .F. ) ;
#195147=DIRECTION ( 'NONE',  ( 0.000000000000000000, 0.9910465087640866200, 0.1335171055202867274 ) ) ;
#195191=CARTESIAN_POINT ( 'NONE',  ( -18.69999999999999929, 11.49641995933507843, -1.885425182446134107 ) ) ;
#195235=AXIS2_PLACEMENT_3D ( 'NONE', #101143, #146713, #120789 ) ;
#195263=EDGE_LOOP ( 'NONE', ( #239654, #52219, #105406, #20332 ) ) ;
#195281=DIRECTION ( 'NONE',  ( 0.000000000000000000, -0.9910465087640866200, 0.1335171055202867274 ) ) ;
#195309=LINE ( 'NONE', #135285, #205395 ) ;
#195344=ADVANCED_FACE ( 'NONE', ( #80094 ), #94553, .T. ) ;
#195350=DIRECTION ( 'NONE',  ( 1.000000000000000000, -0.000000000000000000, -0.000000000000000000 ) ) ;
#195366=CARTESIAN_POINT ( 'NONE',  ( -22.10000000000000497, 6.342459739679072506, 12.00000000000000000 ) ) ;
#195374=ORIENTED_EDGE ( 'NONE', *, *, #68088, .F. ) ;
#195451=DIRECTION ( 'NONE',  ( 0.000000000000000000, -1.000000000000000000, 0.000000000000000000 ) ) ;
#195453=CIRCLE ( 'NONE', #162127, 0.09999999999999939493 ) ;
#195459=ORIENTED_EDGE ( 'NONE', *, *, #103804, .F. ) ;
#195481=EDGE_LOOP ( 'NONE', ( #253108, #126245, #224388, #149279 ) ) ;
#195482=EDGE_CURVE ( 'NONE', #236459, #87211, #213649, .T. ) ;
#195496=VERTEX_POINT ( 'NONE', #50001 ) ;
#195566=DIRECTION ( 'NONE',  ( 1.000000000000000000, -0.000000000000000000, -3.469446951953635646E-14 ) ) ;
#195628=DIRECTION ( 'NONE',  ( 0.000000000000000000, -0.000000000000000000, 1.000000000000000000 ) ) ;
#195683=DIRECTION ( 'NONE',  ( 1.000000000000000000, -0.000000000000000000, 0.000000000000000000 ) ) ;
#195685=LINE ( 'NONE', #210103, #73401 ) ;
#195726=CARTESIAN_POINT ( 'NONE',  ( 11.60000000000000142, -9.650000000000002132, 15.00000000000000355 ) ) ;
#195746=DIRECTION ( 'NONE',  ( 1.000000000000000000, 0.000000000000000000, 0.000000000000000000 ) ) ;
#195757=AXIS2_PLACEMENT_3D ( 'NONE', #133599, #93189, #196146 ) ;
#195785=DIRECTION ( 'NONE',  ( 0.000000000000000000, 1.000000000000000000, 0.000000000000000000 ) ) ;
#195788=DIRECTION ( 'NONE',  ( 0.000000000000000000, 0.000000000000000000, 1.000000000000000000 ) ) ;
#195790=VERTEX_POINT ( 'NONE', #164523 ) ;
#195796=FACE_OUTER_BOUND ( 'NONE', #16133, .T. ) ;
#195799=ORIENTED_EDGE ( 'NONE', *, *, #107671, .F. ) ;
#195805=ORIENTED_EDGE ( 'NONE', *, *, #214497, .T. ) ;
#195813=FACE_OUTER_BOUND ( 'NONE', #214925, .T. ) ;
#195909=CARTESIAN_POINT ( 'NONE',  ( -19.96434256916585070, 5.572646937746800866, 16.50000000334722117 ) ) ;
#195947=DIRECTION ( 'NONE',  ( -0.000000000000000000, -1.000000000000000000, -0.000000000000000000 ) ) ;
#195960=LINE ( 'NONE', #79817, #184160 ) ;
#195962=CARTESIAN_POINT ( 'NONE',  ( -18.59999999999999787, -9.849999999999996092, 31.39999999999999858 ) ) ;
#195979=ADVANCED_FACE ( 'NONE', ( #135304 ), #176257, .F. ) ;
#195987=CARTESIAN_POINT ( 'NONE',  ( -0.8999999999999994671, -8.250000000000005329, 21.95857864376268864 ) ) ;
#195992=ORIENTED_EDGE ( 'NONE', *, *, #243645, .T. ) ;
#195999=AXIS2_PLACEMENT_3D ( 'NONE', #237013, #137882, #156216 ) ;
#196053=CARTESIAN_POINT ( 'NONE',  ( -22.94999999999999929, -1.885425182446134107, -11.49641995933507843 ) ) ;
#196059=CARTESIAN_POINT ( 'NONE',  ( -20.90000000000000213, -1.885425182446133885, -11.49641995933507843 ) ) ;
#196092=ORIENTED_EDGE ( 'NONE', *, *, #26721, .T. ) ;
#196113=CARTESIAN_POINT ( 'NONE',  ( 5.999999999999997335, -11.25000000000000000, 13.90000000000000213 ) ) ;
#196135=VECTOR ( 'NONE', #107822, 1000.000000000000000 ) ;
#196146=DIRECTION ( 'NONE',  ( 0.000000000000000000, -0.1335171055202867274, 0.9910465087640866200 ) ) ;
#196147=CYLINDRICAL_SURFACE ( 'NONE', #153260, 0.09999999999999939493 ) ;
#196148=DIRECTION ( 'NONE',  ( -0.000000000000000000, -0.000000000000000000, -1.000000000000000000 ) ) ;
#196190=CARTESIAN_POINT ( 'NONE',  ( 0.000000000000000000, -11.65000000000000036, 33.00000000000000000 ) ) ;
#196229=DIRECTION ( 'NONE',  ( 1.000000000000000000, 0.000000000000000000, -0.000000000000000000 ) ) ;
#196331=CARTESIAN_POINT ( 'NONE',  ( 18.69999999999999929, -1.467286812112899463, 28.00000000000000000 ) ) ;
#196371=ADVANCED_FACE ( 'NONE', ( #200131 ), #122921, .T. ) ;
#196372=CARTESIAN_POINT ( 'NONE',  ( 13.40000000000000036, -8.279289321881348584, 18.97071067811865674 ) ) ;
#196428=ORIENTED_EDGE ( 'NONE', *, *, #53549, .F. ) ;
#196451=CIRCLE ( 'NONE', #154979, 0.09999999999999939493 ) ;
#196466=EDGE_CURVE ( 'NONE', #247436, #120372, #5371, .T. ) ;
#196469=ADVANCED_FACE ( 'NONE', ( #176727 ), #140130, .T. ) ;
#196472=CARTESIAN_POINT ( 'NONE',  ( -21.04142135623731136, 6.223900101154156594, 12.00000000000000000 ) ) ;
#196512=CARTESIAN_POINT ( 'NONE',  ( -22.94999999999999929, 11.59510167572422112, 1.901609089591594692 ) ) ;
#196520=CIRCLE ( 'NONE', #42400, 0.09999999999999939493 ) ;
#196555=LINE ( 'NONE', #17912, #200837 ) ;
#196593=ORIENTED_EDGE ( 'NONE', *, *, #107069, .T. ) ;
#196685=DIRECTION ( 'NONE',  ( -0.000000000000000000, 1.000000000000000000, -0.000000000000000000 ) ) ;
#196701=ORIENTED_EDGE ( 'NONE', *, *, #125729, .F. ) ;
#196746=ORIENTED_EDGE ( 'NONE', *, *, #154179, .T. ) ;
#196788=DIRECTION ( 'NONE',  ( -2.316152573905153269E-15, -0.9910465087640865089, 0.1335171055202867274 ) ) ;
#196816=DIRECTION ( 'NONE',  ( 0.000000000000000000, -1.000000000000000000, 0.000000000000000000 ) ) ;
#196817=ADVANCED_FACE ( 'NONE', ( #237672 ), #172231, .T. ) ;
#196823=CIRCLE ( 'NONE', #200924, 0.2000000000000000944 ) ;
#196833=CARTESIAN_POINT ( 'NONE',  ( 18.79999999999999716, 1.149999999999999911, -15.00000000000000000 ) ) ;
#196838=FACE_OUTER_BOUND ( 'NONE', #209088, .T. ) ;
#196890=EDGE_CURVE ( 'NONE', #62787, #89611, #105508, .T. ) ;
#196893=EDGE_CURVE ( 'NONE', #63429, #67858, #184644, .T. ) ;
#196970=CARTESIAN_POINT ( 'NONE',  ( 13.40000000000000036, -8.279289321881350361, 15.00000000000000355 ) ) ;
#196973=CARTESIAN_POINT ( 'NONE',  ( 0.000000000000000000, -11.65000000000000036, 32.89999999999999858 ) ) ;
#196994=DIRECTION ( 'NONE',  ( 0.000000000000000000, 0.000000000000000000, -1.000000000000000000 ) ) ;
#197011=ORIENTED_EDGE ( 'NONE', *, *, #236515, .T. ) ;
#197031=ORIENTED_EDGE ( 'NONE', *, *, #189526, .F. ) ;
#197033=DIRECTION ( 'NONE',  ( 1.000000000000000000, 0.000000000000000000, 0.000000000000000000 ) ) ;
#197084=CARTESIAN_POINT ( 'NONE',  ( 11.60000000000000320, -9.650000000000002132, 17.60000000000000497 ) ) ;
#197112=AXIS2_PLACEMENT_3D ( 'NONE', #64170, #201105, #101975 ) ;
#197146=EDGE_LOOP ( 'NONE', ( #162616, #211252, #56511, #82092 ) ) ;
#197152=AXIS2_PLACEMENT_3D ( 'NONE', #255336, #170776, #57163 ) ;
#197187=EDGE_CURVE ( 'NONE', #12756, #106580, #176129, .T. ) ;
#197221=CIRCLE ( 'NONE', #81058, 0.1000000000000028644 ) ;
#197246=DIRECTION ( 'NONE',  ( -1.000000000000000000, 0.000000000000000000, -0.000000000000000000 ) ) ;
#197254=EDGE_CURVE ( 'NONE', #70167, #176282, #101662, .T. ) ;
#197282=DIRECTION ( 'NONE',  ( 0.000000000000000000, 0.000000000000000000, -1.000000000000000000 ) ) ;
#197305=AXIS2_PLACEMENT_3D ( 'NONE', #40179, #87910, #244437 ) ;
#197308=ORIENTED_EDGE ( 'NONE', *, *, #190236, .F. ) ;
#197376=ADVANCED_FACE ( 'NONE', ( #131528 ), #109382, .T. ) ;
#197377=DIRECTION ( 'NONE',  ( -0.000000000000000000, 1.000000000000000000, 0.000000000000000000 ) ) ;
#197427=DIRECTION ( 'NONE',  ( -1.000000000000000000, 0.000000000000000000, 0.000000000000000000 ) ) ;
#197514=FACE_OUTER_BOUND ( 'NONE', #18949, .T. ) ;
#197523=DIRECTION ( 'NONE',  ( -0.000000000000000000, -0.1686199900910294591, 0.9856811345164832039 ) ) ;
#197531=VECTOR ( 'NONE', #115473, 1000.000000000000000 ) ;
#197550=ORIENTED_EDGE ( 'NONE', *, *, #25043, .F. ) ;
#197570=CIRCLE ( 'NONE', #39213, 4.100000000000000533 ) ;
#197573=CIRCLE ( 'NONE', #151825, 0.09999999999999990841 ) ;
#197625=DIRECTION ( 'NONE',  ( 0.000000000000000000, -1.000000000000000000, -0.000000000000000000 ) ) ;
#197680=ORIENTED_EDGE ( 'NONE', *, *, #84971, .F. ) ;
#197689=TOROIDAL_SURFACE ( 'NONE', #27048, 0.2000000000000000111, 0.1000000000000000056 ) ;
#197711=FACE_OUTER_BOUND ( 'NONE', #45226, .T. ) ;
#197735=CARTESIAN_POINT ( 'NONE',  ( 21.10000000000000142, 0.000000000000000000, 4.000000000000000000 ) ) ;
#197751=LINE ( 'NONE', #42523, #238700 ) ;
#197754=ORIENTED_EDGE ( 'NONE', *, *, #123186, .T. ) ;
#197760=FACE_OUTER_BOUND ( 'NONE', #62947, .T. ) ;
#197781=DIRECTION ( 'NONE',  ( 0.000000000000000000, -1.000000000000000000, 0.000000000000000000 ) ) ;
#197785=ORIENTED_EDGE ( 'NONE', *, *, #42319, .T. ) ;
#197836=CARTESIAN_POINT ( 'NONE',  ( 18.79999999999999716, -2.105948478070175156, -13.13328020565119125 ) ) ;
#197850=ADVANCED_FACE ( 'NONE', ( #219406 ), #35401, .T. ) ;
#197888=DIRECTION ( 'NONE',  ( -0.000000000000000000, -0.000000000000000000, 1.000000000000000000 ) ) ;
#197925=ADVANCED_FACE ( 'NONE', ( #99452 ), #235142, .T. ) ;
#197936=DIRECTION ( 'NONE',  ( 0.000000000000000000, -0.9910465087640866200, 0.1335171055202867274 ) ) ;
#197963=DIRECTION ( 'NONE',  ( 0.000000000000000000, 0.000000000000000000, 1.000000000000000000 ) ) ;
#198022=ORIENTED_EDGE ( 'NONE', *, *, #134603, .F. ) ;
#198030=DIRECTION ( 'NONE',  ( 1.000000000000000000, 0.000000000000000000, 0.000000000000000000 ) ) ;
#198038=ORIENTED_EDGE ( 'NONE', *, *, #237310, .T. ) ;
#198059=DIRECTION ( 'NONE',  ( -0.000000000000000000, -0.000000000000000000, -1.000000000000000000 ) ) ;
#198089=ORIENTED_EDGE ( 'NONE', *, *, #237014, .T. ) ;
#198095=ORIENTED_EDGE ( 'NONE', *, *, #45031, .T. ) ;
#198137=CARTESIAN_POINT ( 'NONE',  ( 20.10000000000000853, 5.552655413246003313, 16.61686199900910310 ) ) ;
#198215=ORIENTED_EDGE ( 'NONE', *, *, #166934, .F. ) ;
#198222=DIRECTION ( 'NONE',  ( 0.000000000000000000, 0.1335171055202901413, 0.9910465087640860649 ) ) ;
#198288=EDGE_CURVE ( 'NONE', #184295, #237894, #207131, .T. ) ;
#198290=EDGE_CURVE ( 'NONE', #95570, #136069, #14725, .T. ) ;
#198428=TOROIDAL_SURFACE ( 'NONE', #219267, 11.65000000000000036, 0.1000000000000000056 ) ;
#198443=CIRCLE ( 'NONE', #19969, 0.1000000000000000749 ) ;
#198484=DIRECTION ( 'NONE',  ( 0.000000000000000000, 0.000000000000000000, -1.000000000000000000 ) ) ;
#198489=FACE_OUTER_BOUND ( 'NONE', #241474, .T. ) ;
#198493=DIRECTION ( 'NONE',  ( 1.000000000000000000, -0.000000000000000000, 0.000000000000000000 ) ) ;
#198508=DIRECTION ( 'NONE',  ( 0.000000000000000000, 0.000000000000000000, -1.000000000000000000 ) ) ;
#198523=VERTEX_POINT ( 'NONE', #87160 ) ;
#198554=DIRECTION ( 'NONE',  ( 0.000000000000000000, 0.000000000000000000, 1.000000000000000000 ) ) ;
#198593=AXIS2_PLACEMENT_3D ( 'NONE', #57101, #234472, #54557 ) ;
#198603=FACE_OUTER_BOUND ( 'NONE', #256628, .T. ) ;
#198637=CARTESIAN_POINT ( 'NONE',  ( -22.94999999999999929, 0.000000000000000000, 0.000000000000000000 ) ) ;
#198646=CIRCLE ( 'NONE', #244615, 0.09999999999999939493 ) ;
#198684=EDGE_CURVE ( 'NONE', #118720, #219738, #79145, .T. ) ;
#198778=AXIS2_PLACEMENT_3D ( 'NONE', #157086, #38407, #39719 ) ;
#198787=VECTOR ( 'NONE', #150962, 1000.000000000000227 ) ;
#198835=CARTESIAN_POINT ( 'NONE',  ( -37.88850191057539973, -8.350000000000004974, 10.52591260281975138 ) ) ;
#198844=VECTOR ( 'NONE', #119924, 1000.000000000000000 ) ;
#198958=EDGE_CURVE ( 'NONE', #17438, #74968, #231002, .T. ) ;
#199012=CARTESIAN_POINT ( 'NONE',  ( -18.59999999999999787, -9.849999999999996092, 31.39999999999999858 ) ) ;
#199026=CIRCLE ( 'NONE', #215580, 11.65000000000000036 ) ;
#199030=DIRECTION ( 'NONE',  ( -0.000000000000000000, -0.000000000000000000, -1.000000000000000000 ) ) ;
#199083=ORIENTED_EDGE ( 'NONE', *, *, #107671, .T. ) ;
#199086=DIRECTION ( 'NONE',  ( 1.000000000000000000, -0.000000000000000000, 0.000000000000000000 ) ) ;
#199152=CYLINDRICAL_SURFACE ( 'NONE', #224659, 0.1000000000000001443 ) ;
#199215=CARTESIAN_POINT ( 'NONE',  ( -6.100000000000012079, -11.75000000000000000, -15.00000000000000355 ) ) ;
#199238=EDGE_CURVE ( 'NONE', #173345, #182680, #256037, .T. ) ;
#199294=EDGE_LOOP ( 'NONE', ( #156214, #28631, #175764 ) ) ;
#199340=AXIS2_PLACEMENT_3D ( 'NONE', #246164, #6249, #67517 ) ;
#199421=CARTESIAN_POINT ( 'NONE',  ( 6.099999999999987210, -11.65000000000000036, -15.00000000000001243 ) ) ;
#199423=CARTESIAN_POINT ( 'NONE',  ( -22.94999999999999929, 11.59510167572422112, 1.901609089591594692 ) ) ;
#199428=DIRECTION ( 'NONE',  ( 0.000000000000000000, 0.000000000000000000, -1.000000000000000000 ) ) ;
#199493=CARTESIAN_POINT ( 'NONE',  ( 18.69999999999999929, 10.88519226655716565, -15.14794223642649840 ) ) ;
#199521=CARTESIAN_POINT ( 'NONE',  ( 21.10000000000000142, 4.898587196589412829E-16, -4.000000000000000000 ) ) ;
#199551=ORIENTED_EDGE ( 'NONE', *, *, #211626, .F. ) ;
#199559=AXIS2_PLACEMENT_3D ( 'NONE', #227374, #203956, #205229 ) ;
#199677=ORIENTED_EDGE ( 'NONE', *, *, #167257, .T. ) ;
#199695=DIRECTION ( 'NONE',  ( -1.000000000000000000, 0.000000000000000000, 0.000000000000000000 ) ) ;
#199798=VERTEX_POINT ( 'NONE', #21811 ) ;
#199805=CARTESIAN_POINT ( 'NONE',  ( 18.59999999999999787, -8.250000000000005329, 10.50000000000000178 ) ) ;
#199852=AXIS2_PLACEMENT_3D ( 'NONE', #42052, #163279, #221922 ) ;
#199853=EDGE_CURVE ( 'NONE', #139155, #194632, #242119, .T. ) ;
#199856=FACE_OUTER_BOUND ( 'NONE', #110814, .T. ) ;
#199883=DIRECTION ( 'NONE',  ( 0.000000000000000000, 0.000000000000000000, -1.000000000000000000 ) ) ;
#199915=EDGE_LOOP ( 'NONE', ( #178340, #163461, #170851, #195374 ) ) ;
#199918=AXIS2_PLACEMENT_3D ( 'NONE', #168022, #148427, #11486 ) ;
#199926=DIRECTION ( 'NONE',  ( -0.000000000000000000, -1.000000000000000000, -0.000000000000000000 ) ) ;
#199932=CIRCLE ( 'NONE', #54156, 0.09999999999999939493 ) ;
#199935=ORIENTED_EDGE ( 'NONE', *, *, #246388, .F. ) ;
#199940=ORIENTED_EDGE ( 'NONE', *, *, #256561, .F. ) ;
#199950=FACE_OUTER_BOUND ( 'NONE', #220123, .T. ) ;
#199962=ORIENTED_EDGE ( 'NONE', *, *, #29048, .T. ) ;
#199980=CYLINDRICAL_SURFACE ( 'NONE', #161267, 0.1000000000000028644 ) ;
#199994=AXIS2_PLACEMENT_3D ( 'NONE', #75242, #154781, #234276 ) ;
#200065=CYLINDRICAL_SURFACE ( 'NONE', #61724, 0.09999999999999939493 ) ;
#200081=EDGE_CURVE ( 'NONE', #173524, #75404, #252167, .T. ) ;
#200091=DIRECTION ( 'NONE',  ( 0.000000000000000000, -1.000000000000000000, 0.000000000000000000 ) ) ;
#200095=CARTESIAN_POINT ( 'NONE',  ( -20.90000000000000213, 1.885425182446133885, -11.49641995933507843 ) ) ;
#200098=CARTESIAN_POINT ( 'NONE',  ( -18.79999999999999716, 8.000000000000000000, 1.212568896937007867 ) ) ;
#200099=CIRCLE ( 'NONE', #87649, 0.09999999999999990841 ) ;
#200106=CARTESIAN_POINT ( 'NONE',  ( -20.90000000000000213, -11.75000000000000000, 11.89999999999999858 ) ) ;
#200131=FACE_OUTER_BOUND ( 'NONE', #28103, .T. ) ;
#200132=EDGE_CURVE ( 'NONE', #106580, #59743, #95878, .T. ) ;
#200148=ORIENTED_EDGE ( 'NONE', *, *, #225381, .T. ) ;
#200157=AXIS2_PLACEMENT_3D ( 'NONE', #111818, #53109, #113095 ) ;
#200212=ORIENTED_EDGE ( 'NONE', *, *, #210495, .T. ) ;
#200252=CARTESIAN_POINT ( 'NONE',  ( -21.00000000000000000, 1.885425182446133885, -11.49641995933507843 ) ) ;
#200317=DIRECTION ( 'NONE',  ( 0.000000000000000000, 0.000000000000000000, -1.000000000000000000 ) ) ;
#200345=DIRECTION ( 'NONE',  ( -0.000000000000000000, -0.000000000000000000, -1.000000000000000000 ) ) ;
#200346=DIRECTION ( 'NONE',  ( 0.000000000000000000, 0.000000000000000000, 1.000000000000000000 ) ) ;
#200403=ADVANCED_FACE ( 'NONE', ( #89163 ), #128315, .T. ) ;
#200412=ORIENTED_EDGE ( 'NONE', *, *, #131008, .T. ) ;
#200507=DIRECTION ( 'NONE',  ( 0.000000000000000000, 0.000000000000000000, 1.000000000000000000 ) ) ;
#200533=DIRECTION ( 'NONE',  ( 0.000000000000000000, 0.9910465087640865089, 0.1335171055202864221 ) ) ;
#200550=ADVANCED_FACE ( 'NONE', ( #253380 ), #74790, .F. ) ;
#200620=AXIS2_PLACEMENT_3D ( 'NONE', #232423, #20752, #119860 ) ;
#200624=AXIS2_PLACEMENT_3D ( 'NONE', #3098, #180483, #1819 ) ;
#200625=CARTESIAN_POINT ( 'NONE',  ( -0.8999999999999993561, -11.65000000000000036, 28.60000000000000142 ) ) ;
#200633=CARTESIAN_POINT ( 'NONE',  ( 22.84999999999999787, 0.000000000000000000, 0.000000000000000000 ) ) ;
#200704=LINE ( 'NONE', #53803, #229135 ) ;
#200774=CIRCLE ( 'NONE', #13342, 0.09999999999999939493 ) ;
#200786=AXIS2_PLACEMENT_3D ( 'NONE', #78211, #236004, #155226 ) ;
#200806=EDGE_CURVE ( 'NONE', #213256, #66123, #203030, .T. ) ;
#200820=ORIENTED_EDGE ( 'NONE', *, *, #200806, .F. ) ;
#200824=DIRECTION ( 'NONE',  ( 0.000000000000000000, -1.000000000000000000, 0.000000000000000000 ) ) ;
#200837=VECTOR ( 'NONE', #174493, 1000.000000000000000 ) ;
#200897=ORIENTED_EDGE ( 'NONE', *, *, #256894, .F. ) ;
#200915=VECTOR ( 'NONE', #181275, 1000.000000000000000 ) ;
#200919=CYLINDRICAL_SURFACE ( 'NONE', #152518, 0.09999999999999939493 ) ;
#200924=AXIS2_PLACEMENT_3D ( 'NONE', #90805, #11291, #230323 ) ;
#200931=LINE ( 'NONE', #24887, #253515 ) ;
#200951=VERTEX_POINT ( 'NONE', #209454 ) ;
#200978=ADVANCED_FACE ( 'NONE', ( #153383 ), #193750, .F. ) ;
#201026=ORIENTED_EDGE ( 'NONE', *, *, #117955, .T. ) ;
#201047=CARTESIAN_POINT ( 'NONE',  ( -21.00000000000000000, 1.410778198689825347, -7.973296578895943121 ) ) ;
#201057=DIRECTION ( 'NONE',  ( 1.000000000000000000, 0.000000000000000000, 0.000000000000000000 ) ) ;
#201061=EDGE_CURVE ( 'NONE', #19574, #157545, #86110, .T. ) ;
#201105=DIRECTION ( 'NONE',  ( -0.000000000000000000, -1.000000000000000000, 0.000000000000000000 ) ) ;
#201111=VECTOR ( 'NONE', #55767, 1000.000000000000000 ) ;
#201131=CARTESIAN_POINT ( 'NONE',  ( 20.90000000000000213, 1.901609089591594470, -11.59510167572422112 ) ) ;
#201145=AXIS2_PLACEMENT_3D ( 'NONE', #66659, #169652, #185316 ) ;
#201154=ORIENTED_EDGE ( 'NONE', *, *, #169577, .F. ) ;
#201166=AXIS2_PLACEMENT_3D ( 'NONE', #186137, #149603, #223963 ) ;
#201169=VECTOR ( 'NONE', #192216, 999.9999999999998863 ) ;
#201173=SPHERICAL_SURFACE ( 'NONE', #211109, 0.1000000000000000056 ) ;
#201239=CARTESIAN_POINT ( 'NONE',  ( 19.95447128016623140, 4.513204987603615770, 22.00000000000000355 ) ) ;
#201248=EDGE_LOOP ( 'NONE', ( #53990, #70939, #126074, #104920 ) ) ;
#201255=ORIENTED_EDGE ( 'NONE', *, *, #168943, .F. ) ;
#201275=AXIS2_PLACEMENT_3D ( 'NONE', #121833, #124398, #186958 ) ;
#201292=EDGE_CURVE ( 'NONE', #156872, #212150, #168802, .T. ) ;
#201298=ORIENTED_EDGE ( 'NONE', *, *, #74542, .F. ) ;
#201304=EDGE_CURVE ( 'NONE', #82095, #103469, #115534, .T. ) ;
#201307=CIRCLE ( 'NONE', #242996, 0.09999999999999939493 ) ;
#201333=CARTESIAN_POINT ( 'NONE',  ( 5.899999999999995914, -11.65000000000000036, 10.00000000000000178 ) ) ;
#201414=DIRECTION ( 'NONE',  ( 0.000000000000000000, 0.000000000000000000, -1.000000000000000000 ) ) ;
#201432=CARTESIAN_POINT ( 'NONE',  ( -18.69999999999999929, -10.13229168743236031, -1.028467303599445826 ) ) ;
#201448=VERTEX_POINT ( 'NONE', #99458 ) ;
#201482=VECTOR ( 'NONE', #134065, 1000.000000000000000 ) ;
#201499=LINE ( 'NONE', #84072, #158652 ) ;
#201526=CIRCLE ( 'NONE', #109758, 3.900000000000000355 ) ;
#201545=DIRECTION ( 'NONE',  ( -4.336808689942017736E-16, 0.000000000000000000, -1.000000000000000000 ) ) ;
#201601=ORIENTED_EDGE ( 'NONE', *, *, #63256, .T. ) ;
#201609=CARTESIAN_POINT ( 'NONE',  ( 18.79999999999999716, 0.000000000000000000, 0.000000000000000000 ) ) ;
#201614=AXIS2_PLACEMENT_3D ( 'NONE', #151484, #212729, #154077 ) ;
#201713=VECTOR ( 'NONE', #115594, 1000.000000000000000 ) ;
#201714=CARTESIAN_POINT ( 'NONE',  ( 5.899999999999996803, -11.25000000000000000, 13.90000000000000213 ) ) ;
#201747=CARTESIAN_POINT ( 'NONE',  ( 13.40000000000000036, -11.65000000000000036, 12.30000000000000426 ) ) ;
#201756=ORIENTED_EDGE ( 'NONE', *, *, #240200, .T. ) ;
#201782=DIRECTION ( 'NONE',  ( -1.000000000000000000, -0.000000000000000000, -0.000000000000000000 ) ) ;
#201801=DIRECTION ( 'NONE',  ( 0.000000000000000000, 0.000000000000000000, -1.000000000000000000 ) ) ;
#201823=ORIENTED_EDGE ( 'NONE', *, *, #63875, .F. ) ;
#201835=AXIS2_PLACEMENT_3D ( 'NONE', #51980, #128980, #229368 ) ;
#201860=CARTESIAN_POINT ( 'NONE',  ( -0.8999999999999986899, -12.25000000000000355, 26.00000000000000355 ) ) ;
#201919=CARTESIAN_POINT ( 'NONE',  ( 18.79999999999999005, -1.212568896937008089, -8.000000000000000000 ) ) ;
#202019=CARTESIAN_POINT ( 'NONE',  ( 18.69999999999999929, 8.000000000000000000, -1.212568896937008089 ) ) ;
#202025=CARTESIAN_POINT ( 'NONE',  ( -0.8999999999999986899, -12.25000000000000355, 26.00000000000000355 ) ) ;
#202027=FACE_OUTER_BOUND ( 'NONE', #202609, .T. ) ;
#202057=CIRCLE ( 'NONE', #43833, 0.1000000000000000472 ) ;
#202062=EDGE_CURVE ( 'NONE', #147074, #142179, #161738, .T. ) ;
#202093=DIRECTION ( 'NONE',  ( 0.000000000000000000, 0.000000000000000000, 1.000000000000000000 ) ) ;
#202126=DIRECTION ( 'NONE',  ( -1.000000000000000000, 0.000000000000000000, 0.000000000000000000 ) ) ;
#202166=EDGE_CURVE ( 'NONE', #99532, #89234, #152222, .T. ) ;
#202218=LINE ( 'NONE', #103087, #241083 ) ;
#202235=CARTESIAN_POINT ( 'NONE',  ( 21.00000000000000000, -11.65000000000000036, 11.89999999999999680 ) ) ;
#202238=CIRCLE ( 'NONE', #148237, 0.1000000000000000472 ) ;
#202255=AXIS2_PLACEMENT_3D ( 'NONE', #243313, #158688, #103786 ) ;
#202320=ORIENTED_EDGE ( 'NONE', *, *, #243962, .F. ) ;
#202344=DIRECTION ( 'NONE',  ( 1.000000000000000000, 0.000000000000000000, 0.000000000000000000 ) ) ;
#202359=CIRCLE ( 'NONE', #139802, 0.09999999999999939493 ) ;
#202370=ADVANCED_FACE ( 'NONE', ( #60772 ), #163747, .F. ) ;
#202378=EDGE_CURVE ( 'NONE', #26640, #157564, #186667, .T. ) ;
#202381=DIRECTION ( 'NONE',  ( 0.000000000000000000, 1.000000000000000000, 0.000000000000000000 ) ) ;
#202389=ADVANCED_FACE ( 'NONE', ( #240713 ), #3359, .F. ) ;
#202413=TOROIDAL_SURFACE ( 'NONE', #110835, 4.041421356237310469, 0.1000000000000000056 ) ;
#202420=AXIS2_PLACEMENT_3D ( 'NONE', #71339, #188691, #11346 ) ;
#202432=EDGE_CURVE ( 'NONE', #239767, #66395, #182751, .T. ) ;
#202489=DIRECTION ( 'NONE',  ( 0.000000000000000000, 0.9856811345164800953, 0.1686199900910462790 ) ) ;
#202543=FACE_OUTER_BOUND ( 'NONE', #153528, .T. ) ;
#202566=LINE ( 'NONE', #23951, #14877 ) ;
#202572=EDGE_CURVE ( 'NONE', #17438, #245624, #78741, .T. ) ;
#202609=EDGE_LOOP ( 'NONE', ( #17874, #191710, #95010, #181351 ) ) ;
#202633=CARTESIAN_POINT ( 'NONE',  ( -0.8999999999999994671, -8.279289321881350361, 29.97071067811866030 ) ) ;
#202642=CARTESIAN_POINT ( 'NONE',  ( 18.79999999999999716, 10.88519226655716565, -15.14794223642649840 ) ) ;
#202652=EDGE_CURVE ( 'NONE', #216154, #215604, #236892, .T. ) ;
#202665=EDGE_CURVE ( 'NONE', #137004, #171323, #91156, .T. ) ;
#202669=CARTESIAN_POINT ( 'NONE',  ( 21.00000000000000000, 7.973296578895943121, -1.410778198689825347 ) ) ;
#202694=DIRECTION ( 'NONE',  ( -1.000000000000000000, 0.000000000000000000, 0.000000000000000000 ) ) ;
#202717=DIRECTION ( 'NONE',  ( -1.000000000000000000, 0.000000000000000000, 0.000000000000000000 ) ) ;
#202729=LINE ( 'NONE', #243141, #213851 ) ;
#202818=CIRCLE ( 'NONE', #181983, 0.09999999999999939493 ) ;
#202901=CIRCLE ( 'NONE', #161419, 11.65000000000000036 ) ;
#202945=CARTESIAN_POINT ( 'NONE',  ( -18.79999999999999716, 1.885425182446134107, -11.59641995933507808 ) ) ;
#202963=DIRECTION ( 'NONE',  ( 0.000000000000000000, -0.9910465087640866200, 0.1335171055202867274 ) ) ;
#203014=ORIENTED_EDGE ( 'NONE', *, *, #131614, .F. ) ;
#203030=LINE ( 'NONE', #102624, #65297 ) ;
#203052=ORIENTED_EDGE ( 'NONE', *, *, #177305, .F. ) ;
#203089=AXIS2_PLACEMENT_3D ( 'NONE', #255993, #39609, #240353 ) ;
#203093=AXIS2_PLACEMENT_3D ( 'NONE', #69058, #112029, #27386 ) ;
#203130=AXIS2_PLACEMENT_3D ( 'NONE', #257594, #39925, #195147 ) ;
#203207=ADVANCED_FACE ( 'NONE', ( #24934 ), #104419, .T. ) ;
#203218=CARTESIAN_POINT ( 'NONE',  ( 19.90000000000000568, 1.350000000000000089, 16.60000000000000142 ) ) ;
#203236=CARTESIAN_POINT ( 'NONE',  ( 18.69999999999999929, -9.849999999999994316, 30.09999999999999787 ) ) ;
#203254=CARTESIAN_POINT ( 'NONE',  ( 18.79999999999999716, 9.511171963237318394, 1.617965922123945521 ) ) ;
#203261=EDGE_LOOP ( 'NONE', ( #200212, #256004, #5266, #247346 ) ) ;
#203268=CARTESIAN_POINT ( 'NONE',  ( -20.09999999673964410, 5.571292164246353984, 16.50791943615039159 ) ) ;
#203280=TOROIDAL_SURFACE ( 'NONE', #90834, 0.2000000000000000111, 0.1000000000000000056 ) ;
#203308=DIRECTION ( 'NONE',  ( -0.000000000000000000, -0.000000000000000000, 1.000000000000000000 ) ) ;
#203345=EDGE_LOOP ( 'NONE', ( #21662, #68087, #110633, #185045 ) ) ;
#203405=CARTESIAN_POINT ( 'NONE',  ( -22.94999999999999929, 1.885425182446134107, -11.49641995933507843 ) ) ;
#203489=DIRECTION ( 'NONE',  ( 0.000000000000000000, 0.000000000000000000, -1.000000000000000000 ) ) ;
#203532=ORIENTED_EDGE ( 'NONE', *, *, #171310, .F. ) ;
#203565=LINE ( 'NONE', #24951, #53730 ) ;
#203583=ORIENTED_EDGE ( 'NONE', *, *, #93376, .T. ) ;
#203605=EDGE_LOOP ( 'NONE', ( #47412, #90331, #250912, #22965, #155210 ) ) ;
#203611=DIRECTION ( 'NONE',  ( -0.000000000000000000, 0.1335171055202901413, 0.9910465087640860649 ) ) ;
#203612=LINE ( 'NONE', #238898, #161780 ) ;
#203617=DIRECTION ( 'NONE',  ( 0.000000000000000000, -1.000000000000000000, 0.000000000000000000 ) ) ;
#203623=ORIENTED_EDGE ( 'NONE', *, *, #53020, .T. ) ;
#203630=ORIENTED_EDGE ( 'NONE', *, *, #36982, .F. ) ;
#203718=VERTEX_POINT ( 'NONE', #16295 ) ;
#203738=CIRCLE ( 'NONE', #120383, 3.970710678118657189 ) ;
#203769=CYLINDRICAL_SURFACE ( 'NONE', #144956, 0.09999999999999939493 ) ;
#203781=ORIENTED_EDGE ( 'NONE', *, *, #40078, .T. ) ;
#203797=TOROIDAL_SURFACE ( 'NONE', #124704, 0.2000000000000000111, 0.1000000000000000056 ) ;
#203813=FACE_OUTER_BOUND ( 'NONE', #110001, .T. ) ;
#203823=VERTEX_POINT ( 'NONE', #102182 ) ;
#203828=ORIENTED_EDGE ( 'NONE', *, *, #3965, .T. ) ;
#203870=VERTEX_POINT ( 'NONE', #26555 ) ;
#203927=DIRECTION ( 'NONE',  ( 0.000000000000000000, -0.7071067811865479058, -0.7071067811865472397 ) ) ;
#203939=CARTESIAN_POINT ( 'NONE',  ( -19.89999999999999858, 11.61130914238355771, 16.60000000000000142 ) ) ;
#203956=DIRECTION ( 'NONE',  ( 0.000000000000000000, 1.000000000000000000, 0.000000000000000000 ) ) ;
#203964=VERTEX_POINT ( 'NONE', #151654 ) ;
#204074=DIRECTION ( 'NONE',  ( 1.000000000000000000, 0.000000000000000000, 0.000000000000000000 ) ) ;
#204095=CYLINDRICAL_SURFACE ( 'NONE', #172369, 0.09999999999999939493 ) ;
#204133=DIRECTION ( 'NONE',  ( 0.000000000000000000, 0.000000000000000000, 1.000000000000000000 ) ) ;
#204166=AXIS2_PLACEMENT_3D ( 'NONE', #172522, #251999, #253273 ) ;
#204224=ORIENTED_EDGE ( 'NONE', *, *, #103701, .F. ) ;
#204254=CARTESIAN_POINT ( 'NONE',  ( -19.99999999999999645, 4.547418889303922462, 21.90000000000000213 ) ) ;
#204297=DIRECTION ( 'NONE',  ( 0.000000000000000000, 0.000000000000000000, 1.000000000000000000 ) ) ;
#204306=CARTESIAN_POINT ( 'NONE',  ( -0.8999999999999993561, -8.250000000000005329, 30.04142135623731136 ) ) ;
#204359=DIRECTION ( 'NONE',  ( 0.000000000000000000, -1.000000000000000000, 0.000000000000000000 ) ) ;
#204379=DIRECTION ( 'NONE',  ( 0.000000000000000000, -0.000000000000000000, 1.000000000000000000 ) ) ;
#204387=DIRECTION ( 'NONE',  ( -1.000000000000000000, 0.000000000000000000, 0.000000000000000000 ) ) ;
#204419=AXIS2_PLACEMENT_3D ( 'NONE', #135421, #20640, #79289 ) ;
#204509=CARTESIAN_POINT ( 'NONE',  ( 18.69999999999999929, -8.150000000000007461, 33.00000000000000000 ) ) ;
#204524=CARTESIAN_POINT ( 'NONE',  ( -18.69999999999999929, -11.65000000000000036, 30.09999999999999787 ) ) ;
#204545=CARTESIAN_POINT ( 'NONE',  ( 22.10000000000000142, -1.467286812112899463, 32.90000000000000568 ) ) ;
#204549=DIRECTION ( 'NONE',  ( -0.000000000000000000, 1.000000000000000000, 0.000000000000000000 ) ) ;
#204552=AXIS2_PLACEMENT_3D ( 'NONE', #77534, #237916, #257422 ) ;
#204654=DIRECTION ( 'NONE',  ( -1.000000000000000000, -0.000000000000000000, -0.000000000000000000 ) ) ;
#204744=CIRCLE ( 'NONE', #84078, 0.09999999999999939493 ) ;
#204755=VERTEX_POINT ( 'NONE', #186300 ) ;
#204758=EDGE_CURVE ( 'NONE', #256719, #53312, #109297, .T. ) ;
#204785=CARTESIAN_POINT ( 'NONE',  ( 18.69999999999999929, 1.149999999999999911, -15.00000000000000000 ) ) ;
#204788=AXIS2_PLACEMENT_3D ( 'NONE', #78121, #157725, #215078 ) ;
#204816=DIRECTION ( 'NONE',  ( 0.000000000000000000, 0.000000000000000000, 1.000000000000000000 ) ) ;
#204856=CARTESIAN_POINT ( 'NONE',  ( -0.8999999999999980238, -8.279289321881348584, 22.02928932188134326 ) ) ;
#204887=AXIS2_PLACEMENT_3D ( 'NONE', #175840, #255298, #197936 ) ;
#204912=CIRCLE ( 'NONE', #25875, 0.09999999999999918676 ) ;
#204919=VERTEX_POINT ( 'NONE', #156171 ) ;
#204985=DIRECTION ( 'NONE',  ( 0.000000000000000000, 0.000000000000000000, -1.000000000000000000 ) ) ;
#205007=EDGE_CURVE ( 'NONE', #73306, #51689, #17903, .T. ) ;
#205032=EDGE_CURVE ( 'NONE', #195496, #102722, #21784, .T. ) ;
#205036=CARTESIAN_POINT ( 'NONE',  ( 5.899999999999995914, -11.34999999999999964, 10.00000000000000178 ) ) ;
#205125=VERTEX_POINT ( 'NONE', #179577 ) ;
#205126=EDGE_CURVE ( 'NONE', #12728, #109914, #24357, .T. ) ;
#205135=SHAPE_REPRESENTATION ( 'Fixed End Mounting Bracket', ( #2425 ), #231390 ) ;
#205199=DIRECTION ( 'NONE',  ( 1.000000000000000000, -0.000000000000000000, 0.000000000000000000 ) ) ;
#205216=CARTESIAN_POINT ( 'NONE',  ( 11.60000000000000142, -8.250000000000003553, 12.40000000000000391 ) ) ;
#205229=DIRECTION ( 'NONE',  ( 1.000000000000000000, 0.000000000000000000, 0.000000000000000000 ) ) ;
#205230=CARTESIAN_POINT ( 'NONE',  ( 22.10000000000000142, -11.65000000000000036, 33.00000000000000000 ) ) ;
#205236=ORIENTED_EDGE ( 'NONE', *, *, #153792, .F. ) ;
#205302=CARTESIAN_POINT ( 'NONE',  ( 18.69999999999999929, 7.800000000000000711, -1.212568896937008089 ) ) ;
#205318=ORIENTED_EDGE ( 'NONE', *, *, #111451, .T. ) ;
#205335=LINE ( 'NONE', #184495, #83716 ) ;
#205370=EDGE_CURVE ( 'NONE', #176716, #16688, #61858, .T. ) ;
#205376=ORIENTED_EDGE ( 'NONE', *, *, #66534, .T. ) ;
#205395=VECTOR ( 'NONE', #212293, 1000.000000000000000 ) ;
#205435=AXIS2_PLACEMENT_3D ( 'NONE', #240982, #169176, #49188 ) ;
#205447=EDGE_LOOP ( 'NONE', ( #132048, #39266, #63931, #20593 ) ) ;
#205464=FACE_OUTER_BOUND ( 'NONE', #66303, .T. ) ;
#205471=ORIENTED_EDGE ( 'NONE', *, *, #29398, .F. ) ;
#205490=CARTESIAN_POINT ( 'NONE',  ( 19.90000000000000568, 5.586869315528661062, 16.41686199900910736 ) ) ;
#205505=AXIS2_PLACEMENT_3D ( 'NONE', #116314, #53752, #236240 ) ;
#205517=DIRECTION ( 'NONE',  ( 0.000000000000000000, -0.000000000000000000, -1.000000000000000000 ) ) ;
#205526=FACE_OUTER_BOUND ( 'NONE', #106224, .T. ) ;
#205531=VECTOR ( 'NONE', #92221, 1000.000000000000114 ) ;
#205589=DIRECTION ( 'NONE',  ( -1.000000000000000000, 0.000000000000000000, -0.000000000000000000 ) ) ;
#205592=ORIENTED_EDGE ( 'NONE', *, *, #108514, .T. ) ;
#205603=AXIS2_PLACEMENT_3D ( 'NONE', #160167, #239679, #61024 ) ;
#205620=AXIS2_PLACEMENT_3D ( 'NONE', #208887, #109776, #130633 ) ;
#205691=ORIENTED_EDGE ( 'NONE', *, *, #233408, .F. ) ;
#205700=CARTESIAN_POINT ( 'NONE',  ( -22.94999999999999929, 4.513204987021263825, 22.10000000000000142 ) ) ;
#205735=CARTESIAN_POINT ( 'NONE',  ( -20.90000000000000213, 1.885425182446133885, -11.49641995933507843 ) ) ;
#205737=ORIENTED_EDGE ( 'NONE', *, *, #99045, .F. ) ;
#205754=ORIENTED_EDGE ( 'NONE', *, *, #237014, .F. ) ;
#205789=ORIENTED_EDGE ( 'NONE', *, *, #239238, .F. ) ;
#205834=CARTESIAN_POINT ( 'NONE',  ( -22.19999999999999929, -11.65000000000000036, 32.89999999999999858 ) ) ;
#205858=CARTESIAN_POINT ( 'NONE',  ( 18.59999999999999787, -8.250000000000005329, 10.52591260281975138 ) ) ;
#205890=EDGE_CURVE ( 'NONE', #182680, #8100, #116400, .T. ) ;
#205918=CIRCLE ( 'NONE', #105941, 0.1000000000000000472 ) ;
#206004=LINE ( 'NONE', #88597, #180416 ) ;
#206046=ORIENTED_EDGE ( 'NONE', *, *, #138596, .F. ) ;
#206091=LINE ( 'NONE', #204785, #78557 ) ;
#206115=CARTESIAN_POINT ( 'NONE',  ( 18.69999999999999929, 1.350000000000000089, 21.90000000000000213 ) ) ;
#206123=DIRECTION ( 'NONE',  ( 0.000000000000000000, -0.1335171055202901691, 0.9910465087640861759 ) ) ;
#206125=LINE ( 'NONE', #249120, #158715 ) ;
#206138=FACE_OUTER_BOUND ( 'NONE', #34657, .T. ) ;
#206151=LINE ( 'NONE', #88746, #117952 ) ;
#206152=DIRECTION ( 'NONE',  ( 1.000000000000000000, 0.000000000000000000, 0.000000000000000000 ) ) ;
#206163=DIRECTION ( 'NONE',  ( -1.000000000000000000, -0.000000000000000000, -0.000000000000000000 ) ) ;
#206226=CARTESIAN_POINT ( 'NONE',  ( 18.69999999999999929, -11.65000000000000036, 5.900000000000001243 ) ) ;
#206228=DIRECTION ( 'NONE',  ( 1.000000000000000000, 0.000000000000000000, 0.000000000000000000 ) ) ;
#206233=DIRECTION ( 'NONE',  ( 0.000000000000000000, 0.000000000000000000, 1.000000000000000000 ) ) ;
#206243=DIRECTION ( 'NONE',  ( -1.000000000000000000, 0.000000000000000000, 0.000000000000000000 ) ) ;
#206282=LINE ( 'NONE', #181597, #208199 ) ;
#206297=EDGE_CURVE ( 'NONE', #168528, #134169, #83339, .T. ) ;
#206314=ADVANCED_FACE ( 'NONE', ( #222874 ), #25566, .F. ) ;
#206365=CARTESIAN_POINT ( 'NONE',  ( -22.10000000000000142, -1.467286812112899463, 28.00000000000000000 ) ) ;
#206401=CARTESIAN_POINT ( 'NONE',  ( 18.69999999999999929, -9.749999999999998224, 31.39999999999999858 ) ) ;
#206416=ORIENTED_EDGE ( 'NONE', *, *, #122454, .F. ) ;
#206453=AXIS2_PLACEMENT_3D ( 'NONE', #51992, #190254, #106839 ) ;
#206473=CARTESIAN_POINT ( 'NONE',  ( -21.00000000000000000, -0.04453801223857078301, -0.3305886640091971196 ) ) ;
#206494=ADVANCED_FACE ( 'NONE', ( #29849 ), #133715, .T. ) ;
#206529=ADVANCED_FACE ( 'NONE', ( #10270 ), #89778, .T. ) ;
#206546=ADVANCED_FACE ( 'NONE', ( #22797 ), #604, .T. ) ;
#206560=VECTOR ( 'NONE', #33923, 1000.000000000000000 ) ;
#206620=VERTEX_POINT ( 'NONE', #164856 ) ;
#206622=DIRECTION ( 'NONE',  ( -0.000000000000000000, 1.000000000000000000, -0.000000000000000000 ) ) ;
#206643=VECTOR ( 'NONE', #23609, 1000.000000000000114 ) ;
#206661=PLANE ( 'NONE',  #256233 ) ;
#206772=DIRECTION ( 'NONE',  ( 1.000000000000000000, 0.000000000000000000, 0.000000000000000000 ) ) ;
#206817=CARTESIAN_POINT ( 'NONE',  ( -6.100000000000004086, -11.65000000000000036, 10.10000000000000142 ) ) ;
#206838=VECTOR ( 'NONE', #209011, 1000.000000000000000 ) ;
#206844=FACE_OUTER_BOUND ( 'NONE', #158626, .T. ) ;
#206878=AXIS2_PLACEMENT_3D ( 'NONE', #180072, #58801, #137083 ) ;
#206884=DIRECTION ( 'NONE',  ( -0.000000000000000000, -1.000000000000000000, -0.000000000000000000 ) ) ;
#206892=CARTESIAN_POINT ( 'NONE',  ( 18.79999999999999361, -11.75000000000000000, -15.00000000000000000 ) ) ;
#206966=CARTESIAN_POINT ( 'NONE',  ( -21.00000000000000000, 8.000000000000000000, -1.212568896937008089 ) ) ;
#206998=DIRECTION ( 'NONE',  ( -1.000000000000000000, 0.000000000000000000, 0.000000000000000000 ) ) ;
#207002=CARTESIAN_POINT ( 'NONE',  ( 0.8999999999999993561, -8.250000000000005329, 23.40000000000000568 ) ) ;
#207011=ORIENTED_EDGE ( 'NONE', *, *, #83660, .T. ) ;
#207027=ORIENTED_EDGE ( 'NONE', *, *, #11529, .F. ) ;
#207033=ORIENTED_EDGE ( 'NONE', *, *, #166745, .T. ) ;
#207061=ORIENTED_EDGE ( 'NONE', *, *, #81555, .T. ) ;
#207076=DIRECTION ( 'NONE',  ( 0.000000000000000000, -1.000000000000000000, 0.000000000000000000 ) ) ;
#207131=LINE ( 'NONE', #28533, #243824 ) ;
#207154=DIRECTION ( 'NONE',  ( 0.000000000000000000, 0.8741572761215393728, -0.4856429311786291669 ) ) ;
#207170=CYLINDRICAL_SURFACE ( 'NONE', #152771, 0.09999999999999933942 ) ;
#207171=ADVANCED_FACE ( 'NONE', ( #17041 ), #97810, .F. ) ;
#207174=LINE ( 'NONE', #231883, #253493 ) ;
#207196=EDGE_CURVE ( 'NONE', #233154, #59508, #155286, .T. ) ;
#207213=CARTESIAN_POINT ( 'NONE',  ( -0.8999999999999993561, -8.350000000000004974, 26.00000000000000355 ) ) ;
#207219=DIRECTION ( 'NONE',  ( 0.000000000000000000, -0.000000000000000000, -1.000000000000000000 ) ) ;
#207227=VECTOR ( 'NONE', #156417, 1000.000000000000000 ) ;
#207262=AXIS2_PLACEMENT_3D ( 'NONE', #221501, #45450, #63727 ) ;
#207301=EDGE_CURVE ( 'NONE', #219183, #75451, #76000, .T. ) ;
#207399=ADVANCED_FACE ( 'NONE', ( #181254 ), #82102, .F. ) ;
#207423=CYLINDRICAL_SURFACE ( 'NONE', #23450, 0.09999999999999990841 ) ;
#207439=ORIENTED_EDGE ( 'NONE', *, *, #191258, .T. ) ;
#207448=CYLINDRICAL_SURFACE ( 'NONE', #222164, 0.09999999999999939493 ) ;
#207519=DIRECTION ( 'NONE',  ( 0.000000000000000000, 0.000000000000000000, 1.000000000000000000 ) ) ;
#207543=AXIS2_PLACEMENT_3D ( 'NONE', #255857, #101936, #237636 ) ;
#207572=CARTESIAN_POINT ( 'NONE',  ( -22.94999999999999929, -1.885425182446134107, -11.59641995933507808 ) ) ;
#207583=ORIENTED_EDGE ( 'NONE', *, *, #247380, .T. ) ;
#207627=AXIS2_PLACEMENT_3D ( 'NONE', #152630, #206152, #71796 ) ;
#207646=DIRECTION ( 'NONE',  ( -0.000000000000000000, -0.000000000000000000, -1.000000000000000000 ) ) ;
#207651=FACE_OUTER_BOUND ( 'NONE', #42798, .T. ) ;
#207660=VERTEX_POINT ( 'NONE', #141781 ) ;
#207675=EDGE_CURVE ( 'NONE', #247506, #6846, #172070, .T. ) ;
#207680=DIRECTION ( 'NONE',  ( 0.000000000000000000, -1.000000000000000000, -0.000000000000000000 ) ) ;
#207686=DIRECTION ( 'NONE',  ( 0.000000000000000000, 1.000000000000000000, 0.000000000000000000 ) ) ;
#207700=DIRECTION ( 'NONE',  ( 0.000000000000000000, -0.9856811345164800953, -0.1686199900910462790 ) ) ;
#207782=VECTOR ( 'NONE', #43723, 1000.000000000000000 ) ;
#207809=EDGE_LOOP ( 'NONE', ( #195992, #58803, #18282, #166069 ) ) ;
#207812=DIRECTION ( 'NONE',  ( 0.000000000000000000, 1.000000000000000000, 1.156482317317873105E-15 ) ) ;
#207820=CARTESIAN_POINT ( 'NONE',  ( 19.90000000000000924, 1.350000000000000089, 21.90000000000000213 ) ) ;
#207844=ORIENTED_EDGE ( 'NONE', *, *, #125412, .T. ) ;
#207858=DIRECTION ( 'NONE',  ( -1.000000000000000000, 0.000000000000000000, 0.000000000000000000 ) ) ;
#207861=DIRECTION ( 'NONE',  ( 0.000000000000000000, -0.1335171055202901413, -0.9910465087640860649 ) ) ;
#207912=VERTEX_POINT ( 'NONE', #13842 ) ;
#207937=ORIENTED_EDGE ( 'NONE', *, *, #119630, .T. ) ;
#207939=ORIENTED_EDGE ( 'NONE', *, *, #168326, .F. ) ;
#207941=AXIS2_PLACEMENT_3D ( 'NONE', #1236, #194354, #178645 ) ;
#207988=AXIS2_PLACEMENT_3D ( 'NONE', #212291, #214829, #255187 ) ;
#208008=ORIENTED_EDGE ( 'NONE', *, *, #209794, .F. ) ;
#208058=VERTEX_POINT ( 'NONE', #105862 ) ;
#208062=DIRECTION ( 'NONE',  ( 0.000000000000000000, -1.000000000000000000, 0.000000000000000000 ) ) ;
#208096=VERTEX_POINT ( 'NONE', #9347 ) ;
#208164=FACE_OUTER_BOUND ( 'NONE', #88812, .T. ) ;
#208180=CARTESIAN_POINT ( 'NONE',  ( -18.59999999999999787, -9.849999999999996092, 31.39999999999999858 ) ) ;
#208194=EDGE_LOOP ( 'NONE', ( #12045, #166630, #196428, #113696 ) ) ;
#208199=VECTOR ( 'NONE', #107169, 1000.000000000000000 ) ;
#208203=LINE ( 'NONE', #169098, #99922 ) ;
#208247=CARTESIAN_POINT ( 'NONE',  ( 0.9000000000000000222, -12.25000000000000355, 26.00000000000000355 ) ) ;
#208275=ORIENTED_EDGE ( 'NONE', *, *, #230034, .F. ) ;
#208319=ORIENTED_EDGE ( 'NONE', *, *, #49825, .F. ) ;
#208454=CARTESIAN_POINT ( 'NONE',  ( 13.40000000000000036, -11.65000000000000036, 17.60000000000000497 ) ) ;
#208519=DIRECTION ( 'NONE',  ( -1.000000000000000000, 0.000000000000000000, 0.000000000000000000 ) ) ;
#208565=DIRECTION ( 'NONE',  ( -0.000000000000000000, -1.000000000000000000, 0.000000000000000000 ) ) ;
#208570=CARTESIAN_POINT ( 'NONE',  ( 22.20000000000000284, 3.362550747017869490, 28.82623795144604983 ) ) ;
#208643=DIRECTION ( 'NONE',  ( 0.000000000000000000, -1.000000000000000000, 0.000000000000000000 ) ) ;
#208713=CARTESIAN_POINT ( 'NONE',  ( -6.000000000000003553, -11.34999999999999964, 10.10000000000000142 ) ) ;
#208716=CARTESIAN_POINT ( 'NONE',  ( 18.59999999999999787, -9.849999999999990763, 31.50000000000000000 ) ) ;
#208737=DIRECTION ( 'NONE',  ( 0.000000000000000000, 0.000000000000000000, 1.000000000000000000 ) ) ;
#208769=DIRECTION ( 'NONE',  ( 0.000000000000000000, -0.000000000000000000, 1.000000000000000000 ) ) ;
#208830=AXIS2_PLACEMENT_3D ( 'NONE', #38447, #196229, #175422 ) ;
#208874=ORIENTED_EDGE ( 'NONE', *, *, #142931, .F. ) ;
#208875=CARTESIAN_POINT ( 'NONE',  ( -22.94999999999999929, 6.223900101154156594, 12.09999999999999964 ) ) ;
#208877=VERTEX_POINT ( 'NONE', #200625 ) ;
#208887=CARTESIAN_POINT ( 'NONE',  ( -18.59999999999999787, -10.84999999999999076, -15.00000000000000000 ) ) ;
#208895=TOROIDAL_SURFACE ( 'NONE', #92366, 3.900000000000000355, 0.1000000000000000056 ) ;
#208923=CARTESIAN_POINT ( 'NONE',  ( 18.79999999999999716, 11.50977166988710820, -1.786320531569725478 ) ) ;
#208939=EDGE_LOOP ( 'NONE', ( #45551, #205236, #149477, #124644 ) ) ;
#208961=ORIENTED_EDGE ( 'NONE', *, *, #113779, .T. ) ;
#208987=AXIS2_PLACEMENT_3D ( 'NONE', #92872, #134556, #13357 ) ;
#208990=DIRECTION ( 'NONE',  ( 0.000000000000000000, 0.000000000000000000, 1.000000000000000000 ) ) ;
#208992=EDGE_CURVE ( 'NONE', #184295, #49052, #131060, .T. ) ;
#208994=DIRECTION ( 'NONE',  ( 1.000000000000000000, -0.000000000000000000, 0.000000000000000000 ) ) ;
#209011=DIRECTION ( 'NONE',  ( 1.000000000000000000, -0.000000000000000000, 0.000000000000000000 ) ) ;
#209047=DIRECTION ( 'NONE',  ( 0.000000000000000000, -1.000000000000000000, 0.000000000000000000 ) ) ;
#209077=ADVANCED_FACE ( 'NONE', ( #54374 ), #197689, .T. ) ;
#209079=CARTESIAN_POINT ( 'NONE',  ( 18.79999999999999716, -10.84999999999999076, 33.00000000000000000 ) ) ;
#209088=EDGE_LOOP ( 'NONE', ( #53405, #148652, #59174, #233144 ) ) ;
#209139=VECTOR ( 'NONE', #27440, 1000.000000000000000 ) ;
#209198=CARTESIAN_POINT ( 'NONE',  ( -18.69999999999999929, -9.849999999999942801, -15.00000000000000178 ) ) ;
#209220=CARTESIAN_POINT ( 'NONE',  ( 11.60000000000000320, -8.279289321881350361, 11.02928932188135036 ) ) ;
#209279=DIRECTION ( 'NONE',  ( 0.000000000000000000, -1.000000000000000000, 0.000000000000000000 ) ) ;
#209282=VERTEX_POINT ( 'NONE', #197735 ) ;
#209334=AXIS2_PLACEMENT_3D ( 'NONE', #61011, #160149, #84374 ) ;
#209356=DIRECTION ( 'NONE',  ( 1.000000000000000000, 0.000000000000000000, 0.000000000000000000 ) ) ;
#209374=CARTESIAN_POINT ( 'NONE',  ( 21.10000000000000142, 0.000000000000000000, 0.000000000000000000 ) ) ;
#209400=CARTESIAN_POINT ( 'NONE',  ( -18.69999999999999929, -1.467286812112899463, 28.00000000000000000 ) ) ;
#209402=ORIENTED_EDGE ( 'NONE', *, *, #80637, .F. ) ;
#209441=LINE ( 'NONE', #131185, #99867 ) ;
#209445=DIRECTION ( 'NONE',  ( 0.000000000000000000, 0.000000000000000000, -1.000000000000000000 ) ) ;
#209454=CARTESIAN_POINT ( 'NONE',  ( 18.79999999999999716, 1.350000000000000089, 22.00000000000000355 ) ) ;
#209455=ORIENTED_EDGE ( 'NONE', *, *, #198684, .F. ) ;
#209461=ORIENTED_EDGE ( 'NONE', *, *, #85503, .T. ) ;
#209490=LINE ( 'NONE', #229072, #181414 ) ;
#209509=EDGE_LOOP ( 'NONE', ( #240771, #178622, #75657, #247685 ) ) ;
#209512=DIRECTION ( 'NONE',  ( 0.000000000000000000, -0.000000000000000000, 1.000000000000000000 ) ) ;
#209513=CIRCLE ( 'NONE', #109553, 0.09999999999999993616 ) ;
#209546=CARTESIAN_POINT ( 'NONE',  ( -21.00000000000000000, -1.212568896937008089, -7.900000000000000355 ) ) ;
#209548=EDGE_CURVE ( 'NONE', #166706, #8100, #251294, .T. ) ;
#209565=FACE_OUTER_BOUND ( 'NONE', #44725, .T. ) ;
#209568=EDGE_CURVE ( 'NONE', #9700, #245573, #32951, .T. ) ;
#209569=CARTESIAN_POINT ( 'NONE',  ( -22.94999999999999929, 0.000000000000000000, 0.000000000000000000 ) ) ;
#209592=ORIENTED_EDGE ( 'NONE', *, *, #162166, .F. ) ;
#209594=CARTESIAN_POINT ( 'NONE',  ( -20.10000000000000142, 4.625944962820097039, 22.03401928653448749 ) ) ;
#209609=VERTEX_POINT ( 'NONE', #120193 ) ;
#209630=( NAMED_UNIT ( * ) PLANE_ANGLE_UNIT ( ) SI_UNIT ( $, .RADIAN. ) );
#209634=ORIENTED_EDGE ( 'NONE', *, *, #95248, .F. ) ;
#209664=CARTESIAN_POINT ( 'NONE',  ( 18.79999999999999716, -1.786320531569725478, -11.50977166988710820 ) ) ;
#209666=ORIENTED_EDGE ( 'NONE', *, *, #34547, .T. ) ;
#209687=DIRECTION ( 'NONE',  ( -1.462545276649569224E-15, 0.1686199900910448357, -0.9856811345164804283 ) ) ;
#209721=CIRCLE ( 'NONE', #97236, 3.970710678118657189 ) ;
#209747=VECTOR ( 'NONE', #180345, 1000.000000000000000 ) ;
#209778=ORIENTED_EDGE ( 'NONE', *, *, #38500, .T. ) ;
#209794=EDGE_CURVE ( 'NONE', #90690, #224002, #105720, .T. ) ;
#209795=DIRECTION ( 'NONE',  ( 0.000000000000000000, 0.000000000000000000, -1.000000000000000000 ) ) ;
#209799=ORIENTED_EDGE ( 'NONE', *, *, #100041, .T. ) ;
#209802=AXIS2_PLACEMENT_3D ( 'NONE', #5097, #242445, #63830 ) ;
#209812=FACE_OUTER_BOUND ( 'NONE', #134151, .T. ) ;
#209854=CARTESIAN_POINT ( 'NONE',  ( 18.69999999999998153, 7.986648289447971116, 1.311673547813416718 ) ) ;
#209932=AXIS2_PLACEMENT_3D ( 'NONE', #184546, #219826, #41229 ) ;
#209941=ORIENTED_EDGE ( 'NONE', *, *, #98227, .F. ) ;
#209943=FACE_OUTER_BOUND ( 'NONE', #247918, .T. ) ;
#209957=CARTESIAN_POINT ( 'NONE',  ( -22.94999999999999929, 1.885425182446134107, -11.59641995933507808 ) ) ;
#209958=AXIS2_PLACEMENT_3D ( 'NONE', #17096, #77037, #250539 ) ;
#209979=EDGE_LOOP ( 'NONE', ( #209799, #207439, #30411, #65828 ) ) ;
#209992=DIRECTION ( 'NONE',  ( -1.000000000000000000, -0.000000000000000000, -0.000000000000000000 ) ) ;
#210011=ORIENTED_EDGE ( 'NONE', *, *, #58392, .T. ) ;
#210035=AXIS2_PLACEMENT_3D ( 'NONE', #7083, #65780, #202717 ) ;
#210082=CARTESIAN_POINT ( 'NONE',  ( 21.00000000000000000, 6.258114003436813455, 11.90000000000000036 ) ) ;
#210103=CARTESIAN_POINT ( 'NONE',  ( -18.69999999999999929, 1.350000000000000089, 16.50000000000000000 ) ) ;
#210114=DIRECTION ( 'NONE',  ( -1.000000000000000000, 0.000000000000000000, 0.000000000000000000 ) ) ;
#210183=DIRECTION ( 'NONE',  ( 0.000000000000000000, -1.000000000000000000, 0.000000000000000000 ) ) ;
#210249=LINE ( 'NONE', #113700, #27160 ) ;
#210300=LINE ( 'NONE', #90322, #189172 ) ;
#210330=ORIENTED_EDGE ( 'NONE', *, *, #181630, .T. ) ;
#210334=CARTESIAN_POINT ( 'NONE',  ( -20.90000000000000213, 6.783826713665066066, 9.593862367105556288 ) ) ;
#210339=AXIS2_PLACEMENT_3D ( 'NONE', #227809, #89578, #106563 ) ;
#210377=ORIENTED_EDGE ( 'NONE', *, *, #91235, .T. ) ;
#210410=ORIENTED_EDGE ( 'NONE', *, *, #115386, .T. ) ;
#210423=EDGE_CURVE ( 'NONE', #13384, #118720, #236910, .T. ) ;
#210447=CIRCLE ( 'NONE', #68784, 0.09999999999999939493 ) ;
#210453=CARTESIAN_POINT ( 'NONE',  ( -37.88850191057539973, -10.74999999999999289, 31.59999999999999787 ) ) ;
#210484=DIRECTION ( 'NONE',  ( 0.000000000000000000, 1.000000000000000000, 0.000000000000000000 ) ) ;
#210486=CARTESIAN_POINT ( 'NONE',  ( 18.59999999999999787, -11.65000000000000036, 30.09999999999999787 ) ) ;
#210495=EDGE_CURVE ( 'NONE', #102722, #73021, #97882, .T. ) ;
#210508=ORIENTED_EDGE ( 'NONE', *, *, #170066, .F. ) ;
#210552=TOROIDAL_SURFACE ( 'NONE', #206453, 0.2000000000000000111, 0.1000000000000000056 ) ;
#210579=DIRECTION ( 'NONE',  ( 0.000000000000000000, 0.000000000000000000, -1.000000000000000000 ) ) ;
#210590=DIRECTION ( 'NONE',  ( 1.000000000000000000, 0.000000000000000000, 0.000000000000000000 ) ) ;
#210640=ORIENTED_EDGE ( 'NONE', *, *, #117411, .F. ) ;
#210652=ORIENTED_EDGE ( 'NONE', *, *, #230034, .T. ) ;
#210688=ORIENTED_EDGE ( 'NONE', *, *, #242810, .T. ) ;
#210697=DIRECTION ( 'NONE',  ( 0.000000000000000000, -1.000000000000000000, 0.000000000000000000 ) ) ;
#210706=AXIS2_PLACEMENT_3D ( 'NONE', #185759, #70979, #7107 ) ;
#210723=DIRECTION ( 'NONE',  ( 0.000000000000000000, 0.000000000000000000, 1.000000000000000000 ) ) ;
#210743=DIRECTION ( 'NONE',  ( 0.000000000000000000, 0.000000000000000000, 1.000000000000000000 ) ) ;
#210792=AXIS2_PLACEMENT_3D ( 'NONE', #54622, #134154, #75504 ) ;
#210800=VECTOR ( 'NONE', #199030, 1000.000000000000000 ) ;
#210870=EDGE_LOOP ( 'NONE', ( #53410, #56319, #127325, #231581 ) ) ;
#210883=VERTEX_POINT ( 'NONE', #244295 ) ;
#210885=ORIENTED_EDGE ( 'NONE', *, *, #193254, .F. ) ;
#210913=LINE ( 'NONE', #92236, #6823 ) ;
#210944=( GEOMETRIC_REPRESENTATION_CONTEXT ( 3 ) GLOBAL_UNCERTAINTY_ASSIGNED_CONTEXT ( ( #85677 ) ) GLOBAL_UNIT_ASSIGNED_CONTEXT ( ( #111500, #93207, #89347 ) ) REPRESENTATION_CONTEXT ( 'NONE', 'WORKASPACE' ) );
#210945=ORIENTED_EDGE ( 'NONE', *, *, #99702, .F. ) ;
#210946=ORIENTED_EDGE ( 'NONE', *, *, #98074, .T. ) ;
#210991=DIRECTION ( 'NONE',  ( 0.000000000000000000, 0.000000000000000000, 1.000000000000000000 ) ) ;
#210998=CARTESIAN_POINT ( 'NONE',  ( 22.94999999999999929, -11.64999999999999858, 11.99999999999999645 ) ) ;
#211000=CIRCLE ( 'NONE', #165194, 11.75000000000000000 ) ;
#211037=VERTEX_POINT ( 'NONE', #215447 ) ;
#211053=ADVANCED_FACE ( 'NONE', ( #156794 ), #143292, .T. ) ;
#211068=DIRECTION ( 'NONE',  ( 1.000000000000000000, 0.000000000000000000, 0.000000000000000000 ) ) ;
#211083=ADVANCED_FACE ( 'NONE', ( #243682 ), #158097, .T. ) ;
#211085=DIRECTION ( 'NONE',  ( 1.000000000000000000, 0.000000000000000000, 0.000000000000000000 ) ) ;
#211109=AXIS2_PLACEMENT_3D ( 'NONE', #82477, #62948, #142474 ) ;
#211115=DIRECTION ( 'NONE',  ( -0.000000000000000000, 0.000000000000000000, 1.000000000000000000 ) ) ;
#211127=DIRECTION ( 'NONE',  ( -1.000000000000000000, -0.000000000000000000, -0.000000000000000000 ) ) ;
#211134=ADVANCED_FACE ( 'NONE', ( #44211 ), #15872, .T. ) ;
#211160=AXIS2_PLACEMENT_3D ( 'NONE', #148654, #53386, #172094 ) ;
#211171=VERTEX_POINT ( 'NONE', #125033 ) ;
#211234=DIRECTION ( 'NONE',  ( 0.000000000000000000, 1.000000000000000000, 0.000000000000000000 ) ) ;
#211252=ORIENTED_EDGE ( 'NONE', *, *, #166745, .F. ) ;
#211260=EDGE_CURVE ( 'NONE', #15770, #246137, #6340, .T. ) ;
#211267=DIRECTION ( 'NONE',  ( 0.000000000000000000, -0.9856811345164800953, -0.1686199900910462790 ) ) ;
#211271=CARTESIAN_POINT ( 'NONE',  ( 18.69999999999999929, 0.000000000000000000, 0.000000000000000000 ) ) ;
#211325=FACE_OUTER_BOUND ( 'NONE', #112997, .T. ) ;
#211377=ORIENTED_EDGE ( 'NONE', *, *, #221529, .F. ) ;
#211407=EDGE_CURVE ( 'NONE', #49823, #138780, #98238, .T. ) ;
#211416=CARTESIAN_POINT ( 'NONE',  ( -18.59999999999999787, -11.65000000000000036, 6.100000000000002309 ) ) ;
#211430=FACE_OUTER_BOUND ( 'NONE', #240013, .T. ) ;
#211431=DIRECTION ( 'NONE',  ( 0.000000000000000000, 0.000000000000000000, 1.000000000000000000 ) ) ;
#211432=ORIENTED_EDGE ( 'NONE', *, *, #103701, .T. ) ;
#211460=ORIENTED_EDGE ( 'NONE', *, *, #185689, .T. ) ;
#211482=DIRECTION ( 'NONE',  ( 1.000000000000000000, -0.000000000000000000, 0.000000000000000000 ) ) ;
#211511=AXIS2_PLACEMENT_3D ( 'NONE', #181409, #241373, #142252 ) ;
#211514=ORIENTED_EDGE ( 'NONE', *, *, #18240, .T. ) ;
#211623=DIRECTION ( 'NONE',  ( 0.000000000000000000, -1.000000000000000000, 0.000000000000000000 ) ) ;
#211625=DIRECTION ( 'NONE',  ( 0.000000000000000000, 0.000000000000000000, -1.000000000000000000 ) ) ;
#211626=EDGE_CURVE ( 'NONE', #245971, #215605, #69263, .T. ) ;
#211654=ADVANCED_FACE ( 'NONE', ( #223794 ), #228952, .T. ) ;
#211671=ORIENTED_EDGE ( 'NONE', *, *, #244008, .F. ) ;
#211674=VECTOR ( 'NONE', #38017, 1000.000000000000000 ) ;
#211683=CARTESIAN_POINT ( 'NONE',  ( -18.69999999999999929, -10.84999999999999076, 32.89999999999999858 ) ) ;
#211685=VECTOR ( 'NONE', #36901, 1000.000000000000000 ) ;
#211764=EDGE_CURVE ( 'NONE', #228920, #8033, #65140, .T. ) ;
#211788=CYLINDRICAL_SURFACE ( 'NONE', #238941, 0.09999999999999939493 ) ;
#211793=DIRECTION ( 'NONE',  ( 0.000000000000000000, -0.000000000000000000, 1.000000000000000000 ) ) ;
#211823=AXIS2_PLACEMENT_3D ( 'NONE', #63881, #137305, #181283 ) ;
#211857=EDGE_CURVE ( 'NONE', #92855, #155056, #27767, .T. ) ;
#211882=CIRCLE ( 'NONE', #141150, 0.09999999999999993616 ) ;
#211888=FACE_OUTER_BOUND ( 'NONE', #53681, .T. ) ;
#211927=ORIENTED_EDGE ( 'NONE', *, *, #17635, .F. ) ;
#212026=EDGE_LOOP ( 'NONE', ( #73160, #32309, #101931, #117228 ) ) ;
#212067=AXIS2_PLACEMENT_3D ( 'NONE', #233182, #153678, #74114 ) ;
#212072=AXIS2_PLACEMENT_3D ( 'NONE', #163453, #25242, #185577 ) ;
#212093=ORIENTED_EDGE ( 'NONE', *, *, #108779, .T. ) ;
#212150=VERTEX_POINT ( 'NONE', #168268 ) ;
#212218=ORIENTED_EDGE ( 'NONE', *, *, #94389, .F. ) ;
#212246=CARTESIAN_POINT ( 'NONE',  ( 0.8999999999999993561, -11.75000000000000000, 23.30000000000000426 ) ) ;
#212266=ADVANCED_FACE ( 'NONE', ( #113253 ), #194097, .T. ) ;
#212291=CARTESIAN_POINT ( 'NONE',  ( -37.88850191057539973, -9.849999999999990763, 31.39999999999999858 ) ) ;
#212293=DIRECTION ( 'NONE',  ( 0.000000000000000000, 0.000000000000000000, -1.000000000000000000 ) ) ;
#212373=DIRECTION ( 'NONE',  ( 0.000000000000000000, 0.000000000000000000, 1.000000000000000000 ) ) ;
#212383=EDGE_LOOP ( 'NONE', ( #126385, #203828, #245233, #250599 ) ) ;
#212388=DIRECTION ( 'NONE',  ( -0.000000000000000000, -1.000000000000000000, -1.734723475976757554E-14 ) ) ;
#212440=ORIENTED_EDGE ( 'NONE', *, *, #232779, .F. ) ;
#212453=DIRECTION ( 'NONE',  ( 0.000000000000000000, -8.881784197001252323E-16, 1.000000000000000000 ) ) ;
#212472=EDGE_CURVE ( 'NONE', #194417, #176716, #6120, .T. ) ;
#212509=DIRECTION ( 'NONE',  ( 0.000000000000000000, -1.000000000000000000, 0.000000000000000000 ) ) ;
#212513=ORIENTED_EDGE ( 'NONE', *, *, #199238, .F. ) ;
#212515=CARTESIAN_POINT ( 'NONE',  ( 13.40000000000000036, -11.65000000000000036, 15.00000000000000355 ) ) ;
#212545=ORIENTED_EDGE ( 'NONE', *, *, #5645, .F. ) ;
#212602=ORIENTED_EDGE ( 'NONE', *, *, #75310, .F. ) ;
#212649=CIRCLE ( 'NONE', #17018, 2.600000000000000089 ) ;
#212664=VERTEX_POINT ( 'NONE', #249886 ) ;
#212696=ADVANCED_FACE ( 'NONE', ( #55495 ), #118073, .F. ) ;
#212729=DIRECTION ( 'NONE',  ( 0.000000000000000000, 1.000000000000000000, 0.000000000000000000 ) ) ;
#212747=LINE ( 'NONE', #131914, #46401 ) ;
#212768=EDGE_CURVE ( 'NONE', #203718, #166805, #115500, .T. ) ;
#212773=ORIENTED_EDGE ( 'NONE', *, *, #152304, .F. ) ;
#212785=ORIENTED_EDGE ( 'NONE', *, *, #221092, .F. ) ;
#212786=ORIENTED_EDGE ( 'NONE', *, *, #165993, .T. ) ;
#212791=CARTESIAN_POINT ( 'NONE',  ( -20.90000000000000213, -1.212568896937008089, -7.900000000000000355 ) ) ;
#212818=FACE_OUTER_BOUND ( 'NONE', #149513, .T. ) ;
#212842=DIRECTION ( 'NONE',  ( 1.000000000000000000, -0.000000000000000000, -0.000000000000000000 ) ) ;
#212854=DIRECTION ( 'NONE',  ( 0.000000000000000000, -8.881784197001252323E-16, 1.000000000000000000 ) ) ;
#212900=ORIENTED_EDGE ( 'NONE', *, *, #51416, .F. ) ;
#212906=ORIENTED_EDGE ( 'NONE', *, *, #71599, .T. ) ;
#212907=AXIS2_PLACEMENT_3D ( 'NONE', #199012, #174366, #234275 ) ;
#213056=DIRECTION ( 'NONE',  ( 0.000000000000000000, 0.000000000000000000, -1.000000000000000000 ) ) ;
#213057=CIRCLE ( 'NONE', #221413, 0.1000000000000000472 ) ;
#213091=ADVANCED_FACE ( 'NONE', ( #253419 ), #155651, .T. ) ;
#213124=DIRECTION ( 'NONE',  ( 1.000000000000000000, 0.000000000000000000, 0.000000000000000000 ) ) ;
#213131=CARTESIAN_POINT ( 'NONE',  ( -11.60000000000000320, -8.250000000000005329, 15.00000000000000355 ) ) ;
#213139=LINE ( 'NONE', #97005, #137443 ) ;
#213142=ADVANCED_FACE ( 'NONE', ( #216862 ), #137318, .T. ) ;
#213157=LINE ( 'NONE', #218273, #227753 ) ;
#213179=EDGE_LOOP ( 'NONE', ( #184167, #49925, #234148, #1117 ) ) ;
#213200=CARTESIAN_POINT ( 'NONE',  ( 18.69999999999999929, 1.885425182446133663, -11.49641995933507843 ) ) ;
#213203=DIRECTION ( 'NONE',  ( 0.000000000000000000, 0.000000000000000000, -1.000000000000000000 ) ) ;
#213205=DIRECTION ( 'NONE',  ( -0.000000000000000000, 1.000000000000000000, -0.000000000000000000 ) ) ;
#213256=VERTEX_POINT ( 'NONE', #128051 ) ;
#213313=DIRECTION ( 'NONE',  ( 1.000000000000000000, 0.000000000000000000, 0.000000000000000000 ) ) ;
#213401=CARTESIAN_POINT ( 'NONE',  ( -18.59999999999999787, -10.74999999999999289, -15.00000000000000000 ) ) ;
#213429=ORIENTED_EDGE ( 'NONE', *, *, #33531, .F. ) ;
#213440=DIRECTION ( 'NONE',  ( 1.000000000000000000, 0.000000000000000000, -0.000000000000000000 ) ) ;
#213546=DIRECTION ( 'NONE',  ( -0.000000000000000000, 1.000000000000000000, -0.000000000000000000 ) ) ;
#213563=CYLINDRICAL_SURFACE ( 'NONE', #65718, 0.09999999999999939493 ) ;
#213581=CARTESIAN_POINT ( 'NONE',  ( -22.94999999999999929, 7.900000000000000355, 1.300000000000000044 ) ) ;
#213645=CARTESIAN_POINT ( 'NONE',  ( -18.79999999999999716, -11.75000000000000000, -15.00000000000000000 ) ) ;
#213649=CIRCLE ( 'NONE', #67724, 0.1000000000000028644 ) ;
#213690=CARTESIAN_POINT ( 'NONE',  ( -6.100000000000005862, -11.65000000000000036, 13.90000000000000213 ) ) ;
#213707=ORIENTED_EDGE ( 'NONE', *, *, #127080, .T. ) ;
#213715=AXIS2_PLACEMENT_3D ( 'NONE', #203939, #184366, #5712 ) ;
#213778=DIRECTION ( 'NONE',  ( 1.000000000000000000, -0.000000000000000000, -0.000000000000000000 ) ) ;
#213787=LINE ( 'NONE', #24599, #132749 ) ;
#213797=DIRECTION ( 'NONE',  ( 1.000000000000000000, 0.000000000000000000, -6.938893903907270030E-14 ) ) ;
#213798=LINE ( 'NONE', #152578, #19980 ) ;
#213851=VECTOR ( 'NONE', #120655, 1000.000000000000000 ) ;
#213857=ORIENTED_EDGE ( 'NONE', *, *, #137878, .T. ) ;
#213878=EDGE_LOOP ( 'NONE', ( #17442, #219898, #172882, #183254 ) ) ;
#213887=DIRECTION ( 'NONE',  ( 0.000000000000000000, 8.673617379884087537E-15, 1.000000000000000000 ) ) ;
#213891=ORIENTED_EDGE ( 'NONE', *, *, #130147, .F. ) ;
#213906=CIRCLE ( 'NONE', #30776, 0.1000000000000028644 ) ;
#213968=CARTESIAN_POINT ( 'NONE',  ( 0.000000000000000000, -11.65000000000000036, 33.00000000000000000 ) ) ;
#214026=ADVANCED_FACE ( 'NONE', ( #29328 ), #224899, .F. ) ;
#214037=ORIENTED_EDGE ( 'NONE', *, *, #98439, .F. ) ;
#214039=AXIS2_PLACEMENT_3D ( 'NONE', #256218, #51642, #136313 ) ;
#214050=ORIENTED_EDGE ( 'NONE', *, *, #135729, .F. ) ;
#214100=AXIS2_PLACEMENT_3D ( 'NONE', #171680, #72561, #230325 ) ;
#214113=AXIS2_PLACEMENT_3D ( 'NONE', #29419, #106322, #184596 ) ;
#214140=LINE ( 'NONE', #231156, #224698 ) ;
#214144=ORIENTED_EDGE ( 'NONE', *, *, #61934, .F. ) ;
#214210=ORIENTED_EDGE ( 'NONE', *, *, #189016, .F. ) ;
#214228=DIRECTION ( 'NONE',  ( -1.000000000000000000, -0.000000000000000000, -0.000000000000000000 ) ) ;
#214237=FACE_OUTER_BOUND ( 'NONE', #116853, .T. ) ;
#214269=CIRCLE ( 'NONE', #76883, 0.09999999999999939493 ) ;
#214300=AXIS2_PLACEMENT_3D ( 'NONE', #234997, #121494, #135865 ) ;
#214312=AXIS2_PLACEMENT_3D ( 'NONE', #223927, #47853, #209512 ) ;
#214313=CIRCLE ( 'NONE', #201835, 0.09999999999999939493 ) ;
#214331=FACE_OUTER_BOUND ( 'NONE', #43719, .T. ) ;
#214354=FACE_OUTER_BOUND ( 'NONE', #153783, .T. ) ;
#214374=ADVANCED_FACE ( 'NONE', ( #82505 ), #203769, .T. ) ;
#214380=CARTESIAN_POINT ( 'NONE',  ( -18.79999999999999716, 0.000000000000000000, 33.00000000000000000 ) ) ;
#214398=EDGE_CURVE ( 'NONE', #63710, #691, #36678, .T. ) ;
#214408=PLANE ( 'NONE',  #183871 ) ;
#214489=DIRECTION ( 'NONE',  ( -0.000000000000000000, -0.1686199900910312910, 0.9856811345164826488 ) ) ;
#214497=EDGE_CURVE ( 'NONE', #58688, #59743, #7605, .T. ) ;
#214608=CARTESIAN_POINT ( 'NONE',  ( -18.79999999999999716, -1.212568896937008089, -7.800000000000000711 ) ) ;
#214658=ORIENTED_EDGE ( 'NONE', *, *, #151824, .T. ) ;
#214724=ORIENTED_EDGE ( 'NONE', *, *, #6503, .F. ) ;
#214781=EDGE_CURVE ( 'NONE', #56204, #26640, #40945, .T. ) ;
#214793=VERTEX_POINT ( 'NONE', #160514 ) ;
#214799=LINE ( 'NONE', #32356, #108092 ) ;
#214815=ORIENTED_EDGE ( 'NONE', *, *, #143200, .T. ) ;
#214829=DIRECTION ( 'NONE',  ( -1.000000000000000000, 0.000000000000000000, 0.000000000000000000 ) ) ;
#214838=ORIENTED_EDGE ( 'NONE', *, *, #147764, .F. ) ;
#214904=LINE ( 'NONE', #75428, #245282 ) ;
#214925=EDGE_LOOP ( 'NONE', ( #117223, #193960, #159918, #10587 ) ) ;
#214927=AXIS2_PLACEMENT_3D ( 'NONE', #55974, #112150, #14336 ) ;
#214936=CARTESIAN_POINT ( 'NONE',  ( -18.79999999999999716, -11.65000000000000036, 32.89999999999999858 ) ) ;
#214969=DIRECTION ( 'NONE',  ( -0.000000000000000000, -1.000000000000000000, -0.000000000000000000 ) ) ;
#214981=DIRECTION ( 'NONE',  ( -0.000000000000000000, 1.000000000000000000, -0.000000000000000000 ) ) ;
#215039=AXIS2_PLACEMENT_3D ( 'NONE', #126131, #204387, #166591 ) ;
#215046=ORIENTED_EDGE ( 'NONE', *, *, #241288, .T. ) ;
#215078=DIRECTION ( 'NONE',  ( -1.000000000000000000, -4.336808689942044242E-14, 0.000000000000000000 ) ) ;
#215145=EDGE_LOOP ( 'NONE', ( #135103, #33156, #12454 ) ) ;
#215146=CARTESIAN_POINT ( 'NONE',  ( 11.60000000000000142, -11.65000000000000036, 15.00000000000000355 ) ) ;
#215168=AXIS2_PLACEMENT_3D ( 'NONE', #72479, #155878, #56708 ) ;
#215212=DIRECTION ( 'NONE',  ( 1.000000000000000000, 0.000000000000000000, 0.000000000000000000 ) ) ;
#215220=EDGE_LOOP ( 'NONE', ( #161364, #80306, #219089, #3516 ) ) ;
#215229=EDGE_LOOP ( 'NONE', ( #256931, #180279, #222031, #230153 ) ) ;
#215293=AXIS2_PLACEMENT_3D ( 'NONE', #201609, #182062, #8554 ) ;
#215321=ORIENTED_EDGE ( 'NONE', *, *, #106959, .F. ) ;
#215359=DIRECTION ( 'NONE',  ( 0.000000000000000000, 1.156482317317873105E-15, -1.000000000000000000 ) ) ;
#215365=LINE ( 'NONE', #36778, #16403 ) ;
#215389=DIRECTION ( 'NONE',  ( -4.336808689942017736E-16, 0.000000000000000000, -1.000000000000000000 ) ) ;
#215410=VECTOR ( 'NONE', #78436, 1000.000000000000227 ) ;
#215413=FACE_OUTER_BOUND ( 'NONE', #116102, .T. ) ;
#215447=CARTESIAN_POINT ( 'NONE',  ( -22.10000000000000142, -11.75000000000000000, 12.09999999999999609 ) ) ;
#215480=CARTESIAN_POINT ( 'NONE',  ( 0.8999999999999992450, -8.250000000000005329, 30.04142135623731136 ) ) ;
#215493=CARTESIAN_POINT ( 'NONE',  ( -19.89999999999999858, 1.249999999999999334, 16.50000000000000000 ) ) ;
#215515=EDGE_CURVE ( 'NONE', #89756, #144975, #212649, .T. ) ;
#215516=ORIENTED_EDGE ( 'NONE', *, *, #118085, .F. ) ;
#215541=EDGE_CURVE ( 'NONE', #12728, #223175, #150288, .T. ) ;
#215580=AXIS2_PLACEMENT_3D ( 'NONE', #109239, #128828, #126237 ) ;
#215592=EDGE_CURVE ( 'NONE', #248319, #171697, #71006, .T. ) ;
#215599=LINE ( 'NONE', #57800, #47402 ) ;
#215604=VERTEX_POINT ( 'NONE', #56880 ) ;
#215605=VERTEX_POINT ( 'NONE', #124285 ) ;
#215630=EDGE_LOOP ( 'NONE', ( #168416, #12418, #165590, #65928 ) ) ;
#215632=ORIENTED_EDGE ( 'NONE', *, *, #135729, .T. ) ;
#215695=DIRECTION ( 'NONE',  ( 0.000000000000000000, 0.000000000000000000, 1.000000000000000000 ) ) ;
#215742=DIRECTION ( 'NONE',  ( 0.000000000000000000, 0.000000000000000000, 1.000000000000000000 ) ) ;
#215786=CARTESIAN_POINT ( 'NONE',  ( 18.79999999999999716, 7.900000000000000355, 1.300000000000000044 ) ) ;
#215822=AXIS2_PLACEMENT_3D ( 'NONE', #50268, #129817, #209356 ) ;
#215848=DIRECTION ( 'NONE',  ( -1.000000000000000000, -0.000000000000000000, -0.000000000000000000 ) ) ;
#215900=ORIENTED_EDGE ( 'NONE', *, *, #146996, .T. ) ;
#215906=ORIENTED_EDGE ( 'NONE', *, *, #45110, .F. ) ;
#215921=AXIS2_PLACEMENT_3D ( 'NONE', #27707, #164620, #242857 ) ;
#215924=AXIS2_PLACEMENT_3D ( 'NONE', #148782, #228313, #129210 ) ;
#215935=EDGE_CURVE ( 'NONE', #163777, #66482, #58667, .T. ) ;
#216010=CARTESIAN_POINT ( 'NONE',  ( -22.84999999999999787, 0.000000000000000000, 3.900000000000000355 ) ) ;
#216012=CARTESIAN_POINT ( 'NONE',  ( 21.00000000000000000, -0.04453801223857078301, 0.3305886640091971196 ) ) ;
#216028=EDGE_CURVE ( 'NONE', #130397, #132961, #59720, .T. ) ;
#216039=DIRECTION ( 'NONE',  ( -1.000000000000000000, 0.000000000000000000, 0.000000000000000000 ) ) ;
#216044=DIRECTION ( 'NONE',  ( 0.000000000000000000, 1.000000000000000000, 0.000000000000000000 ) ) ;
#216049=ORIENTED_EDGE ( 'NONE', *, *, #5094, .F. ) ;
#216081=AXIS2_PLACEMENT_3D ( 'NONE', #7040, #147856, #86550 ) ;
#216106=CIRCLE ( 'NONE', #37080, 0.2000000000000005107 ) ;
#216112=AXIS2_PLACEMENT_3D ( 'NONE', #231109, #207686, #169876 ) ;
#216139=DIRECTION ( 'NONE',  ( -0.000000000000000000, -0.1618390714546093789, 0.9868171638914220445 ) ) ;
#216154=VERTEX_POINT ( 'NONE', #246097 ) ;
#216187=DIRECTION ( 'NONE',  ( -1.000000000000000000, 0.000000000000000000, 0.000000000000000000 ) ) ;
#216189=VERTEX_POINT ( 'NONE', #15189 ) ;
#216195=LINE ( 'NONE', #213645, #167621 ) ;
#216199=EDGE_CURVE ( 'NONE', #110926, #23890, #9446, .T. ) ;
#216349=CARTESIAN_POINT ( 'NONE',  ( -19.99999999999999645, 4.547418889303922462, 21.90000000000000213 ) ) ;
#216353=EDGE_LOOP ( 'NONE', ( #11522, #205471, #27716, #249167 ) ) ;
#216404=ORIENTED_EDGE ( 'NONE', *, *, #20406, .F. ) ;
#216425=ORIENTED_EDGE ( 'NONE', *, *, #23138, .F. ) ;
#216426=FACE_OUTER_BOUND ( 'NONE', #135689, .T. ) ;
#216483=ORIENTED_EDGE ( 'NONE', *, *, #66552, .T. ) ;
#216505=ORIENTED_EDGE ( 'NONE', *, *, #201061, .T. ) ;
#216507=ADVANCED_FACE ( 'NONE', ( #47555 ), #29339, .T. ) ;
#216529=AXIS2_PLACEMENT_3D ( 'NONE', #175917, #78061, #221405 ) ;
#216570=CARTESIAN_POINT ( 'NONE',  ( -22.19999999999999929, -11.65000000000000036, 17.70000000000000639 ) ) ;
#216584=EDGE_LOOP ( 'NONE', ( #187047, #229312, #11999, #115029 ) ) ;
#216604=EDGE_LOOP ( 'NONE', ( #37687, #207061, #128767, #242486 ) ) ;
#216727=DIRECTION ( 'NONE',  ( -1.000000000000000000, 0.000000000000000000, -0.000000000000000000 ) ) ;
#216747=DIRECTION ( 'NONE',  ( 0.000000000000000000, 1.000000000000000000, 0.000000000000000000 ) ) ;
#216758=DIRECTION ( 'NONE',  ( 0.000000000000000000, -0.1335171055202878931, -0.9910465087640865089 ) ) ;
#216798=DIRECTION ( 'NONE',  ( -1.462545276649575732E-15, -0.1686199900910455851, 0.9856811345164804283 ) ) ;
#216849=EDGE_CURVE ( 'NONE', #119804, #66395, #130323, .T. ) ;
#216862=FACE_OUTER_BOUND ( 'NONE', #138900, .T. ) ;
#216878=DIRECTION ( 'NONE',  ( 1.000000000000000000, -0.000000000000000000, -0.000000000000000000 ) ) ;
#216897=CARTESIAN_POINT ( 'NONE',  ( -0.8999999999999993561, -11.75000000000000000, 23.30000000000000426 ) ) ;
#216902=ORIENTED_EDGE ( 'NONE', *, *, #17527, .F. ) ;
#216924=ORIENTED_EDGE ( 'NONE', *, *, #90551, .T. ) ;
#216930=ORIENTED_EDGE ( 'NONE', *, *, #66534, .F. ) ;
#217010=DIRECTION ( 'NONE',  ( -1.000000000000000000, 0.000000000000000000, 0.000000000000000000 ) ) ;
#217042=CARTESIAN_POINT ( 'NONE',  ( 18.79999999999999716, 3.461118860469513336, 28.84309995045515507 ) ) ;
#217043=AXIS2_PLACEMENT_3D ( 'NONE', #219578, #121795, #80042 ) ;
#217069=ORIENTED_EDGE ( 'NONE', *, *, #10148, .T. ) ;
#217070=AXIS2_PLACEMENT_3D ( 'NONE', #78862, #137555, #220951 ) ;
#217100=VECTOR ( 'NONE', #242136, 1000.000000000000000 ) ;
#217141=AXIS2_PLACEMENT_3D ( 'NONE', #122262, #201782, #242194 ) ;
#217156=ADVANCED_FACE ( 'NONE', ( #32237 ), #93454, .T. ) ;
#217176=EDGE_CURVE ( 'NONE', #44902, #92180, #201526, .T. ) ;
#217177=LINE ( 'NONE', #157254, #56465 ) ;
#217184=CARTESIAN_POINT ( 'NONE',  ( 18.59999999999999787, -9.849999999999996092, 31.39999999999999858 ) ) ;
#217271=EDGE_LOOP ( 'NONE', ( #1165, #55089, #237830, #35630 ) ) ;
#217289=CYLINDRICAL_SURFACE ( 'NONE', #130711, 0.09999999999999939493 ) ;
#217302=EDGE_CURVE ( 'NONE', #129607, #79153, #158603, .T. ) ;
#217303=EDGE_CURVE ( 'NONE', #66482, #167847, #10206, .T. ) ;
#217328=CARTESIAN_POINT ( 'NONE',  ( 18.59999999999999787, -10.80884033489985363, 6.000000000000001776 ) ) ;
#217337=VERTEX_POINT ( 'NONE', #98556 ) ;
#217405=DIRECTION ( 'NONE',  ( 0.000000000000000000, 1.000000000000000000, -0.000000000000000000 ) ) ;
#217423=EDGE_CURVE ( 'NONE', #16903, #106026, #239132, .T. ) ;
#217449=ORIENTED_EDGE ( 'NONE', *, *, #145128, .T. ) ;
#217459=EDGE_CURVE ( 'NONE', #208096, #67858, #1785, .T. ) ;
#217479=CARTESIAN_POINT ( 'NONE',  ( 18.69999999999999929, -9.849999999999994316, 30.00000000000000355 ) ) ;
#217532=CARTESIAN_POINT ( 'NONE',  ( 5.899999999999996803, -11.65000000000000036, 13.90000000000000213 ) ) ;
#217538=AXIS2_PLACEMENT_3D ( 'NONE', #72453, #91989, #49014 ) ;
#217554=FACE_OUTER_BOUND ( 'NONE', #215220, .T. ) ;
#217563=ORIENTED_EDGE ( 'NONE', *, *, #40078, .F. ) ;
#217712=CIRCLE ( 'NONE', #184411, 0.1000000000000002554 ) ;
#217714=DIRECTION ( 'NONE',  ( 1.000000000000000000, -0.000000000000000000, -0.000000000000000000 ) ) ;
#217816=CARTESIAN_POINT ( 'NONE',  ( 18.69999999999999929, -8.250000000000005329, -15.00000000000000000 ) ) ;
#217817=CYLINDRICAL_SURFACE ( 'NONE', #146593, 0.1000000000000000472 ) ;
#217820=ORIENTED_EDGE ( 'NONE', *, *, #120981, .F. ) ;
#217831=DIRECTION ( 'NONE',  ( 0.000000000000000000, 0.000000000000000000, 1.000000000000000000 ) ) ;
#217837=CIRCLE ( 'NONE', #226194, 0.09999999999999939493 ) ;
#217842=VERTEX_POINT ( 'NONE', #22639 ) ;
#217889=VECTOR ( 'NONE', #142310, 1000.000000000000000 ) ;
#217896=ORIENTED_EDGE ( 'NONE', *, *, #218552, .T. ) ;
#217898=DIRECTION ( 'NONE',  ( 0.000000000000000000, 0.000000000000000000, -1.000000000000000000 ) ) ;
#217909=VERTEX_POINT ( 'NONE', #219518 ) ;
#217930=ORIENTED_EDGE ( 'NONE', *, *, #137092, .T. ) ;
#217990=DIRECTION ( 'NONE',  ( 0.000000000000000000, 0.000000000000000000, 1.000000000000000000 ) ) ;
#218007=DIRECTION ( 'NONE',  ( -0.000000000000000000, 1.000000000000000000, -0.000000000000000000 ) ) ;
#218025=DIRECTION ( 'NONE',  ( -0.000000000000000000, -1.000000000000000000, 0.000000000000000000 ) ) ;
#218045=EDGE_CURVE ( 'NONE', #161554, #37930, #80701, .T. ) ;
#218086=DIRECTION ( 'NONE',  ( 0.000000000000000000, -0.1686199900910313187, 0.9856811345164828708 ) ) ;
#218132=DIRECTION ( 'NONE',  ( 0.000000000000000000, 1.000000000000000000, 0.000000000000000000 ) ) ;
#218160=CARTESIAN_POINT ( 'NONE',  ( -18.79999999999999716, -1.212568896937008089, -8.000000000000000000 ) ) ;
#218163=CIRCLE ( 'NONE', #130698, 0.09999999999999939493 ) ;
#218177=VECTOR ( 'NONE', #6218, 1000.000000000000000 ) ;
#218210=ADVANCED_FACE ( 'NONE', ( #135824 ), #257022, .T. ) ;
#218215=CARTESIAN_POINT ( 'NONE',  ( -19.99999999999999645, 5.454087299794355914, 16.60000000000000142 ) ) ;
#218221=ORIENTED_EDGE ( 'NONE', *, *, #11888, .F. ) ;
#218256=FACE_OUTER_BOUND ( 'NONE', #244217, .T. ) ;
#218273=CARTESIAN_POINT ( 'NONE',  ( -18.69999999999999929, -8.250000000000005329, 32.89999999999999858 ) ) ;
#218276=ORIENTED_EDGE ( 'NONE', *, *, #74139, .T. ) ;
#218286=ADVANCED_FACE ( 'NONE', ( #47956 ), #138382, .T. ) ;
#218300=ORIENTED_EDGE ( 'NONE', *, *, #204758, .F. ) ;
#218301=EDGE_CURVE ( 'NONE', #243832, #203823, #247294, .T. ) ;
#218328=EDGE_LOOP ( 'NONE', ( #41626, #80955, #178635, #156989 ) ) ;
#218381=CARTESIAN_POINT ( 'NONE',  ( 11.60000000000000142, -11.75000000000000000, 15.00000000000000355 ) ) ;
#218395=ADVANCED_FACE ( 'NONE', ( #233049 ), #53095, .T. ) ;
#218410=EDGE_LOOP ( 'NONE', ( #234857, #181704, #247664, #121410 ) ) ;
#218482=ORIENTED_EDGE ( 'NONE', *, *, #3501, .T. ) ;
#218496=ORIENTED_EDGE ( 'NONE', *, *, #214781, .F. ) ;
#218518=DIRECTION ( 'NONE',  ( 1.000000000000000000, 0.000000000000000000, -0.000000000000000000 ) ) ;
#218541=DIRECTION ( 'NONE',  ( 0.000000000000000000, 0.000000000000000000, 1.000000000000000000 ) ) ;
#218545=ORIENTED_EDGE ( 'NONE', *, *, #137543, .T. ) ;
#218552=EDGE_CURVE ( 'NONE', #8033, #2147, #140324, .T. ) ;
#218609=EDGE_CURVE ( 'NONE', #252739, #92180, #105815, .T. ) ;
#218626=ORIENTED_EDGE ( 'NONE', *, *, #111579, .T. ) ;
#218629=CARTESIAN_POINT ( 'NONE',  ( 20.00000000000000355, 5.552655413246002425, 16.61686199900910310 ) ) ;
#218632=DIRECTION ( 'NONE',  ( -0.000000000000000000, 0.9910465087640865089, 0.1335171055202867274 ) ) ;
#218737=DIRECTION ( 'NONE',  ( -1.000000000000000000, 0.000000000000000000, 0.000000000000000000 ) ) ;
#218745=DIRECTION ( 'NONE',  ( 1.000000000000000000, 0.000000000000000000, -0.000000000000000000 ) ) ;
#218777=ADVANCED_FACE ( 'NONE', ( #252263 ), #176777, .T. ) ;
#218786=LINE ( 'NONE', #100109, #114565 ) ;
#218837=CARTESIAN_POINT ( 'NONE',  ( -18.69999999999999929, -8.250000000000005329, -15.00000000000000000 ) ) ;
#218839=DIRECTION ( 'NONE',  ( 0.000000000000000000, -0.7071067811865479058, 0.7071067811865472397 ) ) ;
#218840=CIRCLE ( 'NONE', #85723, 0.1000000000000028644 ) ;
#218870=ORIENTED_EDGE ( 'NONE', *, *, #60162, .T. ) ;
#218912=CIRCLE ( 'NONE', #35787, 0.09999999999999939493 ) ;
#218938=AXIS2_PLACEMENT_3D ( 'NONE', #32884, #211482, #189355 ) ;
#218941=ORIENTED_EDGE ( 'NONE', *, *, #127082, .T. ) ;
#218964=CARTESIAN_POINT ( 'NONE',  ( -21.10000000000000142, -11.75000000000000000, 12.09999999999999609 ) ) ;
#218970=AXIS2_PLACEMENT_3D ( 'NONE', #218160, #119096, #20010 ) ;
#219011=DIRECTION ( 'NONE',  ( 0.000000000000000000, 1.000000000000000000, 0.000000000000000000 ) ) ;
#219036=CARTESIAN_POINT ( 'NONE',  ( -19.89999999999999858, 1.350000000000000089, 16.60000000000000142 ) ) ;
#219055=VERTEX_POINT ( 'NONE', #3071 ) ;
#219067=ADVANCED_FACE ( 'NONE', ( #120506 ), #104721, .T. ) ;
#219074=VECTOR ( 'NONE', #204549, 1000.000000000000000 ) ;
#219089=ORIENTED_EDGE ( 'NONE', *, *, #251682, .F. ) ;
#219100=CARTESIAN_POINT ( 'NONE',  ( 18.59999999999999787, -10.64999999999999325, 33.00000000000000000 ) ) ;
#219122=FACE_OUTER_BOUND ( 'NONE', #229469, .T. ) ;
#219133=ORIENTED_EDGE ( 'NONE', *, *, #226193, .F. ) ;
#219183=VERTEX_POINT ( 'NONE', #27830 ) ;
#219217=EDGE_CURVE ( 'NONE', #131589, #84718, #246831, .T. ) ;
#219219=DIRECTION ( 'NONE',  ( 1.000000000000000000, 0.000000000000000000, 0.000000000000000000 ) ) ;
#219267=AXIS2_PLACEMENT_3D ( 'NONE', #146682, #226208, #148002 ) ;
#219282=CARTESIAN_POINT ( 'NONE',  ( -20.90000000000000213, 1.885425182446133885, -11.49641995933507843 ) ) ;
#219325=DIRECTION ( 'NONE',  ( 1.000000000000000000, -0.000000000000000000, -0.000000000000000000 ) ) ;
#219354=AXIS2_PLACEMENT_3D ( 'NONE', #497, #196148, #159602 ) ;
#219374=VERTEX_POINT ( 'NONE', #181309 ) ;
#219405=EDGE_CURVE ( 'NONE', #247452, #248444, #28685, .T. ) ;
#219406=FACE_OUTER_BOUND ( 'NONE', #247785, .T. ) ;
#219409=DIRECTION ( 'NONE',  ( 1.000000000000000000, -0.000000000000000000, -0.000000000000000000 ) ) ;
#219413=EDGE_CURVE ( 'NONE', #37087, #89611, #230700, .T. ) ;
#219438=AXIS2_PLACEMENT_3D ( 'NONE', #132705, #75317, #32342 ) ;
#219481=EDGE_LOOP ( 'NONE', ( #70445, #200897, #221728, #84023 ) ) ;
#219510=CARTESIAN_POINT ( 'NONE',  ( -19.99999999999999645, 5.488301202077012775, 16.50000000000000000 ) ) ;
#219514=CIRCLE ( 'NONE', #136106, 4.100000000000000533 ) ;
#219518=CARTESIAN_POINT ( 'NONE',  ( -18.79999999999999716, -11.75000000000000000, 32.89999999999999858 ) ) ;
#219544=VERTEX_POINT ( 'NONE', #205834 ) ;
#219564=EDGE_CURVE ( 'NONE', #34850, #161554, #244955, .T. ) ;
#219578=CARTESIAN_POINT ( 'NONE',  ( -18.59999999999999787, -10.64999999999999325, 31.39999999999999858 ) ) ;
#219620=PLANE ( 'NONE',  #253263 ) ;
#219630=ADVANCED_FACE ( 'NONE', ( #11504 ), #8923, .F. ) ;
#219663=AXIS2_PLACEMENT_3D ( 'NONE', #39451, #219325, #198484 ) ;
#219670=ORIENTED_EDGE ( 'NONE', *, *, #68971, .T. ) ;
#219675=DIRECTION ( 'NONE',  ( 1.000000000000000000, 0.000000000000000000, 0.000000000000000000 ) ) ;
#219708=CARTESIAN_POINT ( 'NONE',  ( -19.89999999999999858, 5.586869315528661062, 16.41686199900910736 ) ) ;
#219738=VERTEX_POINT ( 'NONE', #227968 ) ;
#219745=CARTESIAN_POINT ( 'NONE',  ( -21.10000000000000142, 11.99999999999999822, 11.90000000000000036 ) ) ;
#219789=EDGE_CURVE ( 'NONE', #190881, #219055, #169146, .T. ) ;
#219793=FACE_OUTER_BOUND ( 'NONE', #79081, .T. ) ;
#219826=DIRECTION ( 'NONE',  ( -1.000000000000000000, 0.000000000000000000, 0.000000000000000000 ) ) ;
#219883=EDGE_LOOP ( 'NONE', ( #207844, #66193, #139759, #86343 ) ) ;
#219893=DIRECTION ( 'NONE',  ( 1.000000000000000000, -0.000000000000000000, -0.000000000000000000 ) ) ;
#219898=ORIENTED_EDGE ( 'NONE', *, *, #172772, .F. ) ;
#219932=CARTESIAN_POINT ( 'NONE',  ( 20.90000000000000213, 1.885425182446133885, -11.49641995933507843 ) ) ;
#219940=AXIS2_PLACEMENT_3D ( 'NONE', #173851, #152988, #36892 ) ;
#219978=CARTESIAN_POINT ( 'NONE',  ( 20.10000000000000853, 3.461118860469513336, 28.84309995045515507 ) ) ;
#220035=DIRECTION ( 'NONE',  ( 1.000000000000000000, 0.000000000000000000, -0.000000000000000000 ) ) ;
#220086=FACE_OUTER_BOUND ( 'NONE', #205447, .T. ) ;
#220123=EDGE_LOOP ( 'NONE', ( #173043, #163435, #134800, #199940 ) ) ;
#220125=DIRECTION ( 'NONE',  ( 0.000000000000000000, 0.000000000000000000, 1.000000000000000000 ) ) ;
#220126=AXIS2_PLACEMENT_3D ( 'NONE', #154452, #233948, #117842 ) ;
#220154=DIRECTION ( 'NONE',  ( 1.000000000000000000, 0.000000000000000000, 0.000000000000000000 ) ) ;
#220235=DIRECTION ( 'NONE',  ( 1.000000000000000000, 0.000000000000000000, 0.000000000000000000 ) ) ;
#220298=DIRECTION ( 'NONE',  ( 0.000000000000000000, -1.445602896647339410E-16, 1.000000000000000000 ) ) ;
#220383=DIRECTION ( 'NONE',  ( 0.000000000000000000, 0.000000000000000000, -1.000000000000000000 ) ) ;
#220411=DIRECTION ( 'NONE',  ( -0.000000000000000000, 1.000000000000000000, -0.000000000000000000 ) ) ;
#220427=ORIENTED_EDGE ( 'NONE', *, *, #153882, .T. ) ;
#220430=DIRECTION ( 'NONE',  ( -1.000000000000000000, 0.000000000000000000, 0.000000000000000000 ) ) ;
#220479=ORIENTED_EDGE ( 'NONE', *, *, #114824, .T. ) ;
#220480=DIRECTION ( 'NONE',  ( -1.000000000000000000, 0.000000000000000000, 0.000000000000000000 ) ) ;
#220489=ORIENTED_EDGE ( 'NONE', *, *, #103505, .T. ) ;
#220492=ORIENTED_EDGE ( 'NONE', *, *, #16207, .F. ) ;
#220567=VECTOR ( 'NONE', #92686, 1000.000000000000000 ) ;
#220597=EDGE_LOOP ( 'NONE', ( #227926, #4552, #17781, #146140, #45685, #241712, #199677, #77320, #243909, #252078, #51464, #191375, #143024, #43831, #192923, #11372, #135477, #91817, #14187, #96052, #111074, #187987 ) ) ;
#220693=CARTESIAN_POINT ( 'NONE',  ( -11.60000000000000320, -8.250000000000005329, 10.95857864376268864 ) ) ;
#220703=ORIENTED_EDGE ( 'NONE', *, *, #45197, .F. ) ;
#220704=DIRECTION ( 'NONE',  ( -1.000000000000000000, 0.000000000000000000, 0.000000000000000000 ) ) ;
#220735=AXIS2_PLACEMENT_3D ( 'NONE', #18292, #36612, #215212 ) ;
#220755=ADVANCED_FACE ( 'NONE', ( #166783 ), #207170, .T. ) ;
#220790=AXIS2_PLACEMENT_3D ( 'NONE', #109756, #85033, #49791 ) ;
#220794=ORIENTED_EDGE ( 'NONE', *, *, #173914, .T. ) ;
#220800=FACE_OUTER_BOUND ( 'NONE', #216353, .T. ) ;
#220902=CARTESIAN_POINT ( 'NONE',  ( -22.94999999999999929, -1.300000000000000044, -7.900000000000000355 ) ) ;
#220921=AXIS2_PLACEMENT_3D ( 'NONE', #186284, #7640, #67600 ) ;
#220951=DIRECTION ( 'NONE',  ( 1.000000000000000000, 0.000000000000000000, 0.000000000000000000 ) ) ;
#220979=DIRECTION ( 'NONE',  ( 0.000000000000000000, 0.000000000000000000, 1.000000000000000000 ) ) ;
#221004=AXIS2_PLACEMENT_3D ( 'NONE', #2304, #240943, #62299 ) ;
#221023=DIRECTION ( 'NONE',  ( 1.000000000000000000, 0.000000000000000000, 0.000000000000000000 ) ) ;
#221051=VECTOR ( 'NONE', #193680, 1000.000000000000000 ) ;
#221066=DIRECTION ( 'NONE',  ( 0.000000000000000000, -1.000000000000000000, 0.000000000000000000 ) ) ;
#221092=EDGE_CURVE ( 'NONE', #150252, #200951, #97445, .T. ) ;
#221125=DIRECTION ( 'NONE',  ( 0.000000000000000000, 0.000000000000000000, 1.000000000000000000 ) ) ;
#221152=DIRECTION ( 'NONE',  ( 1.000000000000000000, 0.000000000000000000, 0.000000000000000000 ) ) ;
#221223=DIRECTION ( 'NONE',  ( -1.000000000000000000, 0.000000000000000000, 0.000000000000000000 ) ) ;
#221279=LINE ( 'NONE', #161345, #217100 ) ;
#221349=VECTOR ( 'NONE', #63815, 1000.000000000000227 ) ;
#221366=EDGE_LOOP ( 'NONE', ( #185014, #95433, #231685, #212218 ) ) ;
#221368=DIRECTION ( 'NONE',  ( -1.284434275755705789E-16, 0.7071067811865472397, 0.7071067811865479058 ) ) ;
#221405=DIRECTION ( 'NONE',  ( 0.000000000000000000, 0.000000000000000000, -1.000000000000000000 ) ) ;
#221413=AXIS2_PLACEMENT_3D ( 'NONE', #28823, #105706, #185283 ) ;
#221426=VECTOR ( 'NONE', #255174, 1000.000000000000000 ) ;
#221436=ORIENTED_EDGE ( 'NONE', *, *, #132131, .F. ) ;
#221466=CIRCLE ( 'NONE', #121739, 11.65000000000000036 ) ;
#221498=EDGE_CURVE ( 'NONE', #155708, #204919, #257098, .T. ) ;
#221501=CARTESIAN_POINT ( 'NONE',  ( -18.59999999999999787, -8.150000000000005684, 10.52591260281975138 ) ) ;
#221529=EDGE_CURVE ( 'NONE', #58261, #219055, #228127, .T. ) ;
#221559=TOROIDAL_SURFACE ( 'NONE', #171730, 0.2000000000000000111, 0.1000000000000000056 ) ;
#221599=CARTESIAN_POINT ( 'NONE',  ( -18.59999999999999787, -9.849999999999990763, 31.39999999999999858 ) ) ;
#221632=EDGE_CURVE ( 'NONE', #141361, #28188, #127010, .T. ) ;
#221685=ORIENTED_EDGE ( 'NONE', *, *, #11876, .T. ) ;
#221687=DIRECTION ( 'NONE',  ( 0.000000000000000000, -1.000000000000000000, 0.000000000000000000 ) ) ;
#221722=VECTOR ( 'NONE', #214969, 1000.000000000000000 ) ;
#221728=ORIENTED_EDGE ( 'NONE', *, *, #25343, .F. ) ;
#221747=DIRECTION ( 'NONE',  ( 1.000000000000000000, -0.000000000000000000, 0.000000000000000000 ) ) ;
#221766=CARTESIAN_POINT ( 'NONE',  ( 18.79999999999999716, 1.250000000000000000, 21.90000000000000213 ) ) ;
#221804=VERTEX_POINT ( 'NONE', #99083 ) ;
#221815=FACE_BOUND ( 'NONE', #194810, .T. ) ;
#221836=ORIENTED_EDGE ( 'NONE', *, *, #243962, .T. ) ;
#221857=EDGE_CURVE ( 'NONE', #211037, #178041, #45132, .T. ) ;
#221905=DIRECTION ( 'NONE',  ( 0.000000000000000000, 0.1686199900910294591, -0.9856811345164832039 ) ) ;
#221922=DIRECTION ( 'NONE',  ( 0.000000000000000000, 0.000000000000000000, -1.000000000000000000 ) ) ;
#221953=LINE ( 'NONE', #240280, #235316 ) ;
#221964=DIRECTION ( 'NONE',  ( 0.000000000000000000, 0.000000000000000000, -1.000000000000000000 ) ) ;
#221991=VERTEX_POINT ( 'NONE', #246326 ) ;
#221995=ORIENTED_EDGE ( 'NONE', *, *, #147764, .T. ) ;
#221998=LINE ( 'NONE', #4245, #46854 ) ;
#222031=ORIENTED_EDGE ( 'NONE', *, *, #218609, .T. ) ;
#222062=CARTESIAN_POINT ( 'NONE',  ( 20.09999999673965121, 4.627350251755220079, 22.02580456186781532 ) ) ;
#222164=AXIS2_PLACEMENT_3D ( 'NONE', #28850, #108339, #228293 ) ;
#222182=DIRECTION ( 'NONE',  ( 1.000000000000000000, -0.000000000000000000, -0.000000000000000000 ) ) ;
#222185=FACE_OUTER_BOUND ( 'NONE', #11984, .T. ) ;
#222194=EDGE_CURVE ( 'NONE', #190789, #243888, #175791, .T. ) ;
#222239=EDGE_LOOP ( 'NONE', ( #216483, #162692, #86682, #71654 ) ) ;
#222256=LINE ( 'NONE', #184439, #29531 ) ;
#222264=CIRCLE ( 'NONE', #109856, 2.599999999999998312 ) ;
#222298=CIRCLE ( 'NONE', #18331, 4.000000000000000000 ) ;
#222316=FACE_OUTER_BOUND ( 'NONE', #23596, .T. ) ;
#222392=CARTESIAN_POINT ( 'NONE',  ( 5.899999999999996803, -11.75000000000000000, 13.90000000000000213 ) ) ;
#222503=ADVANCED_FACE ( 'NONE', ( #32125 ), #98872, .T. ) ;
#222544=DIRECTION ( 'NONE',  ( 1.284434275755705296E-16, -0.7071067811865471286, -0.7071067811865479058 ) ) ;
#222569=DIRECTION ( 'NONE',  ( -1.000000000000000000, 0.000000000000000000, 0.000000000000000000 ) ) ;
#222719=CARTESIAN_POINT ( 'NONE',  ( 18.79999999999999716, 7.800000000000000711, 1.212568896937007867 ) ) ;
#222730=ORIENTED_EDGE ( 'NONE', *, *, #93376, .F. ) ;
#222760=ORIENTED_EDGE ( 'NONE', *, *, #221529, .T. ) ;
#222768=CARTESIAN_POINT ( 'NONE',  ( 20.90000000000000213, 7.900000000000000355, -1.212568896937008089 ) ) ;
#222804=AXIS2_PLACEMENT_3D ( 'NONE', #234479, #18000, #231944 ) ;
#222836=DIRECTION ( 'NONE',  ( 0.000000000000000000, -0.1335171055202867274, 0.9910465087640866200 ) ) ;
#222846=DIRECTION ( 'NONE',  ( 1.000000000000000000, -0.000000000000000000, -0.000000000000000000 ) ) ;
#222856=LINE ( 'NONE', #165473, #67263 ) ;
#222874=FACE_OUTER_BOUND ( 'NONE', #6242, .T. ) ;
#222922=EDGE_CURVE ( 'NONE', #92448, #236459, #46214, .T. ) ;
#222937=CARTESIAN_POINT ( 'NONE',  ( -18.59999999999999787, -10.80884033489985363, 6.100000000000002309 ) ) ;
#222990=ORIENTED_EDGE ( 'NONE', *, *, #17527, .T. ) ;
#222992=CARTESIAN_POINT ( 'NONE',  ( -20.98284271247461064, 6.322468214605803993, 12.11686199900910488 ) ) ;
#223007=ORIENTED_EDGE ( 'NONE', *, *, #14671, .T. ) ;
#223079=VERTEX_POINT ( 'NONE', #57766 ) ;
#223110=EDGE_CURVE ( 'NONE', #71927, #14083, #174160, .T. ) ;
#223161=DIRECTION ( 'NONE',  ( 0.000000000000000000, 0.000000000000000000, 1.000000000000000000 ) ) ;
#223168=VECTOR ( 'NONE', #69686, 1000.000000000000000 ) ;
#223175=VERTEX_POINT ( 'NONE', #10519 ) ;
#223210=EDGE_LOOP ( 'NONE', ( #6158, #216930, #191596, #238239 ) ) ;
#223218=DIRECTION ( 'NONE',  ( -0.000000000000000000, 0.000000000000000000, 1.000000000000000000 ) ) ;
#223240=DIRECTION ( 'NONE',  ( 0.000000000000000000, 0.000000000000000000, 1.000000000000000000 ) ) ;
#223369=ORIENTED_EDGE ( 'NONE', *, *, #7808, .F. ) ;
#223435=CARTESIAN_POINT ( 'NONE',  ( -22.10000000000000497, 6.223900101154156594, 12.09999999999999964 ) ) ;
#223499=AXIS2_PLACEMENT_3D ( 'NONE', #154336, #149173, #233831 ) ;
#223531=ADVANCED_FACE ( 'NONE', ( #80228 ), #159824, .T. ) ;
#223591=CIRCLE ( 'NONE', #65406, 0.09999999999999939493 ) ;
#223611=EDGE_CURVE ( 'NONE', #132097, #198523, #106228, .T. ) ;
#223633=ORIENTED_EDGE ( 'NONE', *, *, #40887, .T. ) ;
#223673=AXIS2_PLACEMENT_3D ( 'NONE', #195052, #73833, #252417 ) ;
#223733=ORIENTED_EDGE ( 'NONE', *, *, #187979, .F. ) ;
#223754=ORIENTED_EDGE ( 'NONE', *, *, #118417, .T. ) ;
#223778=VERTEX_POINT ( 'NONE', #57815 ) ;
#223793=DIRECTION ( 'NONE',  ( 0.000000000000000000, 1.000000000000000000, -1.224646799147353207E-16 ) ) ;
#223794=FACE_OUTER_BOUND ( 'NONE', #45142, .T. ) ;
#223803=ORIENTED_EDGE ( 'NONE', *, *, #68165, .T. ) ;
#223811=CARTESIAN_POINT ( 'NONE',  ( -18.79999999999999716, 11.49641995933507665, 1.885425182446133663 ) ) ;
#223819=CYLINDRICAL_SURFACE ( 'NONE', #91496, 0.09999999999999945044 ) ;
#223820=DIRECTION ( 'NONE',  ( -0.000000000000000000, 1.000000000000000000, -0.000000000000000000 ) ) ;
#223840=ORIENTED_EDGE ( 'NONE', *, *, #145146, .T. ) ;
#223895=AXIS2_PLACEMENT_3D ( 'NONE', #86910, #28284, #109055 ) ;
#223900=DIRECTION ( 'NONE',  ( 1.000000000000000000, -0.000000000000000000, -0.000000000000000000 ) ) ;
#223927=CARTESIAN_POINT ( 'NONE',  ( 0.000000000000000000, -11.25000000000000000, 0.000000000000000000 ) ) ;
#223935=CIRCLE ( 'NONE', #194763, 0.09999999999999939493 ) ;
#223963=DIRECTION ( 'NONE',  ( 0.000000000000000000, 0.000000000000000000, 1.000000000000000000 ) ) ;
#223972=DIRECTION ( 'NONE',  ( -0.000000000000000000, 0.9910465087640860649, -0.1335171055202901413 ) ) ;
#223993=DIRECTION ( 'NONE',  ( 0.000000000000000000, -1.000000000000000000, 0.000000000000000000 ) ) ;
#224002=VERTEX_POINT ( 'NONE', #26430 ) ;
#224019=DIRECTION ( 'NONE',  ( 0.000000000000000000, 0.000000000000000000, -1.000000000000000000 ) ) ;
#224056=CARTESIAN_POINT ( 'NONE',  ( -18.69999999999999929, -11.65000000000000036, 32.89999999999999858 ) ) ;
#224085=CARTESIAN_POINT ( 'NONE',  ( 21.00000000000000000, -11.75000000000000178, 11.89999999999999680 ) ) ;
#224102=ADVANCED_FACE ( 'NONE', ( #92791 ), #128883, .F. ) ;
#224123=ORIENTED_EDGE ( 'NONE', *, *, #159213, .T. ) ;
#224148=VECTOR ( 'NONE', #48394, 1000.000000000000227 ) ;
#224262=ORIENTED_EDGE ( 'NONE', *, *, #133954, .T. ) ;
#224304=CARTESIAN_POINT ( 'NONE',  ( 21.10000000000000142, -11.65000000000000036, 11.89999999999999680 ) ) ;
#224307=CARTESIAN_POINT ( 'NONE',  ( -13.40000000000000036, -11.75000000000000000, 12.30000000000000426 ) ) ;
#224314=EDGE_CURVE ( 'NONE', #58261, #174523, #249674, .T. ) ;
#224354=CARTESIAN_POINT ( 'NONE',  ( 21.10000000000000142, 6.322468214605804882, 12.11686199900910310 ) ) ;
#224359=CIRCLE ( 'NONE', #82672, 0.09999999999999939493 ) ;
#224388=ORIENTED_EDGE ( 'NONE', *, *, #211764, .F. ) ;
#224418=DIRECTION ( 'NONE',  ( 0.000000000000000000, 0.9910465087640866200, -0.1335171055202867274 ) ) ;
#224511=DIRECTION ( 'NONE',  ( 0.000000000000000000, 0.000000000000000000, -1.000000000000000000 ) ) ;
#224539=FACE_OUTER_BOUND ( 'NONE', #132464, .T. ) ;
#224601=EDGE_CURVE ( 'NONE', #253988, #53312, #20742, .T. ) ;
#224605=DIRECTION ( 'NONE',  ( 0.000000000000000000, 0.000000000000000000, -1.000000000000000000 ) ) ;
#224623=VERTEX_POINT ( 'NONE', #38962 ) ;
#224630=EDGE_CURVE ( 'NONE', #91491, #45068, #58294, .T. ) ;
#224640=DIRECTION ( 'NONE',  ( 0.000000000000000000, 1.000000000000000000, 0.000000000000000000 ) ) ;
#224646=CIRCLE ( 'NONE', #233063, 0.09999999999999963085 ) ;
#224647=CARTESIAN_POINT ( 'NONE',  ( 20.90000000000000213, -1.885425182446133885, -11.49641995933507843 ) ) ;
#224659=AXIS2_PLACEMENT_3D ( 'NONE', #194041, #57038, #257782 ) ;
#224678=CARTESIAN_POINT ( 'NONE',  ( -20.90000000000000213, 7.800000000000000711, -1.212568896937008089 ) ) ;
#224698=VECTOR ( 'NONE', #35536, 1000.000000000000000 ) ;
#224723=ORIENTED_EDGE ( 'NONE', *, *, #36075, .T. ) ;
#224732=ORIENTED_EDGE ( 'NONE', *, *, #10904, .T. ) ;
#224781=LINE ( 'NONE', #160987, #130808 ) ;
#224885=ORIENTED_EDGE ( 'NONE', *, *, #173239, .T. ) ;
#224899=CYLINDRICAL_SURFACE ( 'NONE', #257161, 2.600000000000001421 ) ;
#224916=ORIENTED_EDGE ( 'NONE', *, *, #60826, .T. ) ;
#224932=CIRCLE ( 'NONE', #112537, 0.1000000000000000472 ) ;
#224947=FACE_OUTER_BOUND ( 'NONE', #154821, .T. ) ;
#225005=AXIS2_PLACEMENT_3D ( 'NONE', #130137, #209687, #31089 ) ;
#225014=DIRECTION ( 'NONE',  ( -1.000000000000000000, 0.000000000000000000, -0.000000000000000000 ) ) ;
#225025=LINE ( 'NONE', #88074, #40624 ) ;
#225036=VERTEX_POINT ( 'NONE', #3017 ) ;
#225040=CARTESIAN_POINT ( 'NONE',  ( 19.95447128016623140, 5.488301201494659942, 16.50000000000000000 ) ) ;
#225154=CARTESIAN_POINT ( 'NONE',  ( 19.95857864376268864, 5.488301202077012775, 16.50000000000000000 ) ) ;
#225177=ADVANCED_FACE ( 'NONE', ( #228520 ), #70746, .F. ) ;
#225182=CIRCLE ( 'NONE', #112787, 0.09999999999999939493 ) ;
#225198=AXIS2_PLACEMENT_3D ( 'NONE', #110565, #248810, #188819 ) ;
#225225=ORIENTED_EDGE ( 'NONE', *, *, #76402, .F. ) ;
#225267=AXIS2_PLACEMENT_3D ( 'NONE', #78001, #19322, #134118 ) ;
#225313=DIRECTION ( 'NONE',  ( 0.000000000000000000, 0.000000000000000000, 1.000000000000000000 ) ) ;
#225320=ORIENTED_EDGE ( 'NONE', *, *, #198290, .F. ) ;
#225354=EDGE_LOOP ( 'NONE', ( #143992, #241348, #145745, #59351 ) ) ;
#225358=DIRECTION ( 'NONE',  ( 0.000000000000000000, 0.8741572761215371523, -0.4856429311786332748 ) ) ;
#225381=EDGE_CURVE ( 'NONE', #193487, #45997, #62716, .T. ) ;
#225413=AXIS2_PLACEMENT_3D ( 'NONE', #52713, #31909, #8473 ) ;
#225429=DIRECTION ( 'NONE',  ( -0.000000000000000000, 0.000000000000000000, 1.000000000000000000 ) ) ;
#225493=LINE ( 'NONE', #7770, #167163 ) ;
#225509=CARTESIAN_POINT ( 'NONE',  ( -5.900000000000002132, -11.65000000000000036, 14.10000000000000142 ) ) ;
#225537=CIRCLE ( 'NONE', #204887, 0.09999999999999990841 ) ;
#225605=ORIENTED_EDGE ( 'NONE', *, *, #232779, .T. ) ;
#225642=EDGE_CURVE ( 'NONE', #53312, #131589, #109524, .T. ) ;
#225649=ADVANCED_FACE ( 'NONE', ( #209943 ), #192618, .T. ) ;
#225794=CARTESIAN_POINT ( 'NONE',  ( 22.19999999999999929, -11.65000000000000036, 12.09999999999999787 ) ) ;
#225828=ORIENTED_EDGE ( 'NONE', *, *, #69293, .T. ) ;
#225836=ORIENTED_EDGE ( 'NONE', *, *, #26671, .T. ) ;
#225856=EDGE_CURVE ( 'NONE', #114049, #243012, #180163, .T. ) ;
#225866=FACE_OUTER_BOUND ( 'NONE', #117860, .T. ) ;
#225875=EDGE_CURVE ( 'NONE', #162811, #204755, #59295, .T. ) ;
#225895=VECTOR ( 'NONE', #50821, 1000.000000000000000 ) ;
#225918=EDGE_CURVE ( 'NONE', #82535, #135547, #147104, .T. ) ;
#225939=EDGE_CURVE ( 'NONE', #200951, #52766, #184512, .T. ) ;
#225943=EDGE_LOOP ( 'NONE', ( #15933, #149054, #76012, #95471, #78271, #14029, #79874, #76706 ) ) ;
#226001=PLANE ( 'NONE',  #57924 ) ;
#226042=DIRECTION ( 'NONE',  ( -0.000000000000000000, 1.000000000000000000, -0.000000000000000000 ) ) ;
#226059=CIRCLE ( 'NONE', #13707, 0.09999999999999939493 ) ;
#226102=EDGE_LOOP ( 'NONE', ( #174540, #11660, #109809 ) ) ;
#226123=ORIENTED_EDGE ( 'NONE', *, *, #145870, .F. ) ;
#226154=CIRCLE ( 'NONE', #197152, 0.09999999999999939493 ) ;
#226163=LINE ( 'NONE', #228790, #131272 ) ;
#226191=AXIS2_PLACEMENT_3D ( 'NONE', #48103, #8980, #49400 ) ;
#226193=EDGE_CURVE ( 'NONE', #98150, #246378, #137762, .T. ) ;
#226194=AXIS2_PLACEMENT_3D ( 'NONE', #98360, #257420, #194965 ) ;
#226199=DIRECTION ( 'NONE',  ( 0.000000000000000000, 0.000000000000000000, 1.000000000000000000 ) ) ;
#226208=DIRECTION ( 'NONE',  ( -1.000000000000000000, 0.000000000000000000, 0.000000000000000000 ) ) ;
#226217=EDGE_CURVE ( 'NONE', #199798, #232547, #197751, .T. ) ;
#226241=EDGE_CURVE ( 'NONE', #203718, #82204, #230310, .T. ) ;
#226306=FACE_OUTER_BOUND ( 'NONE', #128083, .T. ) ;
#226320=ORIENTED_EDGE ( 'NONE', *, *, #235983, .T. ) ;
#226333=CIRCLE ( 'NONE', #209802, 0.1000000000000028644 ) ;
#226407=DIRECTION ( 'NONE',  ( 0.000000000000000000, -0.1686199900910312910, 0.9856811345164826488 ) ) ;
#226453=CARTESIAN_POINT ( 'NONE',  ( 22.10000000000000142, -11.65000000000000036, 32.89999999999999858 ) ) ;
#226486=DIRECTION ( 'NONE',  ( 0.000000000000000000, -0.8741572761215384846, 0.4856429311786307212 ) ) ;
#226508=ADVANCED_FACE ( 'NONE', ( #72385 ), #192317, .T. ) ;
#226534=VECTOR ( 'NONE', #97514, 1000.000000000000000 ) ;
#226604=CIRCLE ( 'NONE', #247465, 0.1000000000000000472 ) ;
#226655=DIRECTION ( 'NONE',  ( 1.000000000000000000, -0.000000000000000000, -0.000000000000000000 ) ) ;
#226670=DIRECTION ( 'NONE',  ( 1.000000000000000000, -0.000000000000000000, 0.000000000000000000 ) ) ;
#226683=EDGE_LOOP ( 'NONE', ( #188679, #194732, #109973 ) ) ;
#226724=CARTESIAN_POINT ( 'NONE',  ( -22.20000000000000284, 11.75000000000000000, -15.00000000000000000 ) ) ;
#226793=CARTESIAN_POINT ( 'NONE',  ( -18.79999999999999716, -11.75000000000000000, 5.900000000000001243 ) ) ;
#226827=AXIS2_PLACEMENT_3D ( 'NONE', #90108, #131818, #206228 ) ;
#226889=ORIENTED_EDGE ( 'NONE', *, *, #177474, .F. ) ;
#226901=CARTESIAN_POINT ( 'NONE',  ( -20.90000000000000213, 0.000000000000000000, 0.000000000000000000 ) ) ;
#226913=DIRECTION ( 'NONE',  ( -0.000000000000000000, 1.000000000000000000, -0.000000000000000000 ) ) ;
#226942=CARTESIAN_POINT ( 'NONE',  ( -22.94999999999999929, -1.901609089591594692, -11.59510167572422112 ) ) ;
#226988=EDGE_CURVE ( 'NONE', #66961, #203823, #24823, .T. ) ;
#226991=ORIENTED_EDGE ( 'NONE', *, *, #99081, .F. ) ;
#226995=CIRCLE ( 'NONE', #168789, 0.09999999999999939493 ) ;
#227055=CARTESIAN_POINT ( 'NONE',  ( -21.10000000000000142, 6.223900101154156594, 12.00000000000000000 ) ) ;
#227122=AXIS2_PLACEMENT_3D ( 'NONE', #177839, #100795, #21334 ) ;
#227186=DIRECTION ( 'NONE',  ( 0.000000000000000000, 0.000000000000000000, 1.000000000000000000 ) ) ;
#227201=CIRCLE ( 'NONE', #2328, 0.09999999999999939493 ) ;
#227310=AXIS2_PLACEMENT_3D ( 'NONE', #194526, #116262, #78391 ) ;
#227318=CARTESIAN_POINT ( 'NONE',  ( -22.94999999999999929, 7.900000000000000355, -1.300000000000000044 ) ) ;
#227342=ADVANCED_FACE ( 'NONE', ( #121031 ), #1011, .T. ) ;
#227343=DIRECTION ( 'NONE',  ( 0.000000000000000000, 0.000000000000000000, 1.000000000000000000 ) ) ;
#227374=CARTESIAN_POINT ( 'NONE',  ( -22.10000000000000497, 6.223900101154157483, 12.09999999999999964 ) ) ;
#227386=AXIS2_PLACEMENT_3D ( 'NONE', #218837, #100158, #237138 ) ;
#227421=ORIENTED_EDGE ( 'NONE', *, *, #127815, .F. ) ;
#227472=DIRECTION ( 'NONE',  ( -0.000000000000000000, 1.000000000000000000, -0.000000000000000000 ) ) ;
#227544=CARTESIAN_POINT ( 'NONE',  ( 18.69999999999999929, 6.726092018229619995, 9.512212474619552438 ) ) ;
#227553=LINE ( 'NONE', #107606, #46374 ) ;
#227562=DIRECTION ( 'NONE',  ( 0.000000000000000000, 0.000000000000000000, -1.000000000000000000 ) ) ;
#227607=CARTESIAN_POINT ( 'NONE',  ( 20.90000000000000213, 8.000000000000000000, -1.212568896937008089 ) ) ;
#227633=ORIENTED_EDGE ( 'NONE', *, *, #173156, .T. ) ;
#227709=EDGE_CURVE ( 'NONE', #105564, #134169, #127001, .T. ) ;
#227753=VECTOR ( 'NONE', #99601, 1000.000000000000000 ) ;
#227790=EDGE_CURVE ( 'NONE', #189583, #975, #226163, .T. ) ;
#227809=CARTESIAN_POINT ( 'NONE',  ( -21.10000000000000142, -11.65000000000000036, 12.09999999999999609 ) ) ;
#227838=CARTESIAN_POINT ( 'NONE',  ( 20.90000000000000213, 11.49641995933507843, -1.885425182446133885 ) ) ;
#227918=DIRECTION ( 'NONE',  ( 0.000000000000000000, 0.000000000000000000, -1.000000000000000000 ) ) ;
#227926=ORIENTED_EDGE ( 'NONE', *, *, #153176, .F. ) ;
#227960=VECTOR ( 'NONE', #230522, 1000.000000000000000 ) ;
#227968=CARTESIAN_POINT ( 'NONE',  ( -18.79999999999999716, 7.986648289447971116, -1.311673547813416718 ) ) ;
#227985=CYLINDRICAL_SURFACE ( 'NONE', #55019, 0.09999999999999939493 ) ;
#227995=VERTEX_POINT ( 'NONE', #23886 ) ;
#228022=CARTESIAN_POINT ( 'NONE',  ( 13.40000000000000036, -8.250000000000003553, 12.40000000000000391 ) ) ;
#228065=CIRCLE ( 'NONE', #69858, 0.09999999999999939493 ) ;
#228096=CYLINDRICAL_SURFACE ( 'NONE', #89349, 2.599999999999998312 ) ;
#228127=CIRCLE ( 'NONE', #53141, 0.09999999999999939493 ) ;
#228145=ADVANCED_FACE ( 'NONE', ( #228490 ), #66836, .T. ) ;
#228210=CIRCLE ( 'NONE', #244743, 0.1000000000000002554 ) ;
#228235=ORIENTED_EDGE ( 'NONE', *, *, #12245, .F. ) ;
#228264=CARTESIAN_POINT ( 'NONE',  ( 18.69999999999999929, 11.75000000000000000, 5.900000000000002132 ) ) ;
#228268=DIRECTION ( 'NONE',  ( -1.000000000000000000, -0.000000000000000000, -0.000000000000000000 ) ) ;
#228293=DIRECTION ( 'NONE',  ( -1.000000000000000000, 1.476360405086655403E-16, 0.000000000000000000 ) ) ;
#228313=DIRECTION ( 'NONE',  ( 0.000000000000000000, 0.000000000000000000, -1.000000000000000000 ) ) ;
#228324=CARTESIAN_POINT ( 'NONE',  ( -13.40000000000000036, -9.650000000000005684, 12.40000000000000391 ) ) ;
#228355=DIRECTION ( 'NONE',  ( -0.000000000000000000, 1.000000000000000000, 0.000000000000000000 ) ) ;
#228366=CARTESIAN_POINT ( 'NONE',  ( 21.00000000000000000, 7.800000000000000711, 0.000000000000000000 ) ) ;
#228397=EDGE_CURVE ( 'NONE', #219738, #149939, #247387, .T. ) ;
#228400=ORIENTED_EDGE ( 'NONE', *, *, #253681, .F. ) ;
#228421=VECTOR ( 'NONE', #130706, 1000.000000000000114 ) ;
#228431=ORIENTED_EDGE ( 'NONE', *, *, #45031, .F. ) ;
#228459=AXIS2_PLACEMENT_3D ( 'NONE', #132983, #71727, #31339 ) ;
#228461=ORIENTED_EDGE ( 'NONE', *, *, #44673, .T. ) ;
#228485=CARTESIAN_POINT ( 'NONE',  ( -18.59999999999999787, -11.65000000000000036, 30.09999999999999787 ) ) ;
#228490=FACE_OUTER_BOUND ( 'NONE', #170949, .T. ) ;
#228503=ORIENTED_EDGE ( 'NONE', *, *, #92015, .T. ) ;
#228514=VECTOR ( 'NONE', #203611, 1000.000000000000114 ) ;
#228520=FACE_OUTER_BOUND ( 'NONE', #36971, .T. ) ;
#228659=EDGE_LOOP ( 'NONE', ( #244004, #2475, #82134 ) ) ;
#228681=DIRECTION ( 'NONE',  ( 0.000000000000000000, -1.776356839400250465E-15, -1.000000000000000000 ) ) ;
#228731=ORIENTED_EDGE ( 'NONE', *, *, #113828, .T. ) ;
#228790=CARTESIAN_POINT ( 'NONE',  ( -22.94999999999999929, -1.786320531569725478, -11.50977166988710820 ) ) ;
#228869=CIRCLE ( 'NONE', #183088, 11.75000000000000000 ) ;
#228920=VERTEX_POINT ( 'NONE', #52733 ) ;
#228927=ORIENTED_EDGE ( 'NONE', *, *, #195070, .F. ) ;
#228952=CYLINDRICAL_SURFACE ( 'NONE', #15086, 0.09999999999999939493 ) ;
#228964=AXIS2_PLACEMENT_3D ( 'NONE', #12891, #211068, #29889 ) ;
#228967=CARTESIAN_POINT ( 'NONE',  ( -18.79999999999999716, 11.49641995933507843, -1.885425182446133885 ) ) ;
#228976=DIRECTION ( 'NONE',  ( 0.000000000000000000, 0.1618390714546044939, 0.9868171638914228216 ) ) ;
#228982=CARTESIAN_POINT ( 'NONE',  ( 18.79999999999999716, 1.885425182446134107, -11.59641995933507808 ) ) ;
#228987=DIRECTION ( 'NONE',  ( -1.000000000000000000, -1.476360405086644309E-16, 0.000000000000000000 ) ) ;
#228993=EDGE_CURVE ( 'NONE', #102889, #126, #81894, .T. ) ;
#229012=ORIENTED_EDGE ( 'NONE', *, *, #44778, .F. ) ;
#229038=DIRECTION ( 'NONE',  ( -0.000000000000000000, 0.4856429311786307212, 0.8741572761215384846 ) ) ;
#229069=CARTESIAN_POINT ( 'NONE',  ( 22.10000000000000142, -1.467286812112899463, 28.00000000000000000 ) ) ;
#229072=CARTESIAN_POINT ( 'NONE',  ( 18.59999999999999787, -10.74999999999999289, 31.50000000000000000 ) ) ;
#229092=FACE_OUTER_BOUND ( 'NONE', #208194, .T. ) ;
#229119=EDGE_CURVE ( 'NONE', #5669, #89956, #65582, .T. ) ;
#229120=CIRCLE ( 'NONE', #199918, 0.09999999999999993616 ) ;
#229135=VECTOR ( 'NONE', #258059, 1000.000000000000000 ) ;
#229185=DIRECTION ( 'NONE',  ( 0.000000000000000000, -0.1335171055202866441, -0.9910465087640865089 ) ) ;
#229205=SURFACE_STYLE_USAGE ( .BOTH. , #47977 ) ;
#229226=CARTESIAN_POINT ( 'NONE',  ( 18.69999999999999929, -11.65000000000000036, 33.00000000000000000 ) ) ;
#229312=ORIENTED_EDGE ( 'NONE', *, *, #114043, .F. ) ;
#229328=EDGE_LOOP ( 'NONE', ( #56146, #219133, #232404, #4859 ) ) ;
#229335=ORIENTED_EDGE ( 'NONE', *, *, #191230, .F. ) ;
#229368=DIRECTION ( 'NONE',  ( 0.000000000000000000, 0.000000000000000000, -1.000000000000000000 ) ) ;
#229406=FACE_OUTER_BOUND ( 'NONE', #138816, .T. ) ;
#229425=DIRECTION ( 'NONE',  ( 0.000000000000000000, 0.000000000000000000, 1.000000000000000000 ) ) ;
#229453=EDGE_LOOP ( 'NONE', ( #44955, #34218, #212900, #57534 ) ) ;
#229469=EDGE_LOOP ( 'NONE', ( #155859, #253561, #73883, #170830 ) ) ;
#229503=TOROIDAL_SURFACE ( 'NONE', #21241, 0.2000000000000000111, 0.1000000000000000056 ) ;
#229602=CIRCLE ( 'NONE', #62996, 0.09999999999999990841 ) ;
#229641=AXIS2_PLACEMENT_3D ( 'NONE', #128252, #207812, #104787 ) ;
#229643=DIRECTION ( 'NONE',  ( 0.000000000000000000, 1.000000000000000000, 0.000000000000000000 ) ) ;
#229644=EDGE_CURVE ( 'NONE', #223778, #122251, #146044, .T. ) ;
#229665=ORIENTED_EDGE ( 'NONE', *, *, #164491, .F. ) ;
#229667=EDGE_CURVE ( 'NONE', #114049, #73021, #52126, .T. ) ;
#229715=CARTESIAN_POINT ( 'NONE',  ( 18.79999999999999716, -8.150000000000007461, 33.00000000000000000 ) ) ;
#229724=CIRCLE ( 'NONE', #217043, 0.1000000000000028644 ) ;
#229776=ORIENTED_EDGE ( 'NONE', *, *, #64589, .F. ) ;
#229815=AXIS2_PLACEMENT_3D ( 'NONE', #83572, #1491, #99293 ) ;
#229840=CARTESIAN_POINT ( 'NONE',  ( 18.69999999999999929, 0.000000000000000000, 0.000000000000000000 ) ) ;
#229872=CIRCLE ( 'NONE', #184079, 11.65000000000000036 ) ;
#229875=CARTESIAN_POINT ( 'NONE',  ( -19.89999999999999858, 5.488301202077012775, 16.50000000000000000 ) ) ;
#229921=EDGE_CURVE ( 'NONE', #253988, #34850, #175969, .T. ) ;
#229925=DIRECTION ( 'NONE',  ( -0.000000000000000000, -1.000000000000000000, -0.000000000000000000 ) ) ;
#229936=EDGE_LOOP ( 'NONE', ( #79378, #125902, #225320, #178499 ) ) ;
#230015=AXIS2_PLACEMENT_3D ( 'NONE', #105043, #145492, #200346 ) ;
#230025=EDGE_CURVE ( 'NONE', #89611, #235390, #223935, .T. ) ;
#230033=AXIS2_PLACEMENT_3D ( 'NONE', #230125, #188426, #51460 ) ;
#230034=EDGE_CURVE ( 'NONE', #166706, #240745, #228065, .T. ) ;
#230036=ORIENTED_EDGE ( 'NONE', *, *, #221632, .F. ) ;
#230057=ORIENTED_EDGE ( 'NONE', *, *, #254114, .T. ) ;
#230125=CARTESIAN_POINT ( 'NONE',  ( -18.79999999999999716, -11.65000000000000036, 32.89999999999999858 ) ) ;
#230153=ORIENTED_EDGE ( 'NONE', *, *, #217176, .F. ) ;
#230163=CIRCLE ( 'NONE', #117740, 4.000000000000000000 ) ;
#230175=DIRECTION ( 'NONE',  ( -1.000000000000000000, 0.000000000000000000, 0.000000000000000000 ) ) ;
#230193=ORIENTED_EDGE ( 'NONE', *, *, #46938, .F. ) ;
#230202=CONICAL_SURFACE ( 'NONE', #59471, 4.000000000000000000, 0.7853981633974487231 ) ;
#230216=CARTESIAN_POINT ( 'NONE',  ( 5.899999999999997691, -11.34999999999999964, 13.90000000000000213 ) ) ;
#230229=EDGE_CURVE ( 'NONE', #193487, #195790, #198443, .T. ) ;
#230285=CARTESIAN_POINT ( 'NONE',  ( 11.60000000000000320, -8.350000000000004974, 19.04142135623731136 ) ) ;
#230296=VECTOR ( 'NONE', #98512, 1000.000000000000000 ) ;
#230305=ORIENTED_EDGE ( 'NONE', *, *, #104008, .T. ) ;
#230310=CIRCLE ( 'NONE', #117876, 0.09999999999999939493 ) ;
#230323=DIRECTION ( 'NONE',  ( 0.000000000000000000, 0.000000000000000000, -1.000000000000000000 ) ) ;
#230325=DIRECTION ( 'NONE',  ( 0.000000000000000000, -0.9856811345164803173, -0.1686199900910455851 ) ) ;
#230326=ADVANCED_FACE ( 'NONE', ( #218256 ), #196147, .F. ) ;
#230372=VECTOR ( 'NONE', #163954, 1000.000000000000000 ) ;
#230380=SPHERICAL_SURFACE ( 'NONE', #121424, 0.1000000000000000056 ) ;
#230424=ORIENTED_EDGE ( 'NONE', *, *, #73226, .F. ) ;
#230455=EDGE_LOOP ( 'NONE', ( #236410, #127379, #124468, #69309 ) ) ;
#230471=DIRECTION ( 'NONE',  ( 0.000000000000000000, -0.9856811345164832039, -0.1686199900910280158 ) ) ;
#230522=DIRECTION ( 'NONE',  ( 0.000000000000000000, -1.000000000000000000, 0.000000000000000000 ) ) ;
#230560=CARTESIAN_POINT ( 'NONE',  ( -19.89999999999999858, 1.350000000000000089, 21.90000000000000213 ) ) ;
#230585=CARTESIAN_POINT ( 'NONE',  ( 18.79999999999999716, -11.74999999999999645, 33.00000000000000000 ) ) ;
#230600=AXIS2_PLACEMENT_3D ( 'NONE', #178305, #99989, #21787 ) ;
#230601=CARTESIAN_POINT ( 'NONE',  ( -21.00000000000000000, 1.311673547813416718, -7.986648289447971116 ) ) ;
#230633=DIRECTION ( 'NONE',  ( 0.000000000000000000, -1.000000000000000000, 0.000000000000000000 ) ) ;
#230648=EDGE_CURVE ( 'NONE', #63710, #76531, #95460, .T. ) ;
#230650=ORIENTED_EDGE ( 'NONE', *, *, #12245, .T. ) ;
#230690=ADVANCED_FACE ( 'NONE', ( #255781 ), #58878, .F. ) ;
#230700=LINE ( 'NONE', #152460, #168806 ) ;
#230731=DIRECTION ( 'NONE',  ( 1.000000000000000000, -0.000000000000000000, -0.000000000000000000 ) ) ;
#230792=DIRECTION ( 'NONE',  ( 0.000000000000000000, 0.000000000000000000, -1.000000000000000000 ) ) ;
#230794=EDGE_CURVE ( 'NONE', #5568, #12989, #121482, .T. ) ;
#230832=EDGE_CURVE ( 'NONE', #57087, #99741, #86173, .T. ) ;
#230845=DIRECTION ( 'NONE',  ( -0.000000000000000000, 1.000000000000000000, -0.000000000000000000 ) ) ;
#230858=LINE ( 'NONE', #57306, #57240 ) ;
#230895=VECTOR ( 'NONE', #147155, 1000.000000000000000 ) ;
#230931=EDGE_LOOP ( 'NONE', ( #96270, #159573, #46200, #88946 ) ) ;
#230938=AXIS2_PLACEMENT_3D ( 'NONE', #111815, #250030, #230471 ) ;
#230981=ORIENTED_EDGE ( 'NONE', *, *, #41916, .F. ) ;
#231002=CIRCLE ( 'NONE', #126924, 0.1999999999999996503 ) ;
#231003=ORIENTED_EDGE ( 'NONE', *, *, #133144, .T. ) ;
#231013=EDGE_CURVE ( 'NONE', #245971, #223079, #202901, .T. ) ;
#231031=CIRCLE ( 'NONE', #160310, 0.09999999999999990841 ) ;
#231104=DIRECTION ( 'NONE',  ( 0.000000000000000000, 0.1335171055202901413, 0.9910465087640860649 ) ) ;
#231109=CARTESIAN_POINT ( 'NONE',  ( -5.900000000000003020, -11.25000000000000000, 10.10000000000000142 ) ) ;
#231133=VECTOR ( 'NONE', #147295, 1000.000000000000000 ) ;
#231144=LINE ( 'NONE', #192016, #2853 ) ;
#231155=CYLINDRICAL_SURFACE ( 'NONE', #178540, 0.09999999999999939493 ) ;
#231156=CARTESIAN_POINT ( 'NONE',  ( -18.69999999999999929, -11.75000000000000000, 29.89999999999999858 ) ) ;
#231188=CARTESIAN_POINT ( 'NONE',  ( -22.10000000000000142, -11.64999999999999858, 11.99999999999999645 ) ) ;
#231230=DIRECTION ( 'NONE',  ( 0.000000000000000000, 0.000000000000000000, -1.000000000000000000 ) ) ;
#231323=DIRECTION ( 'NONE',  ( 0.000000000000000000, -0.1335171055202901413, -0.9910465087640860649 ) ) ;
#231337=ORIENTED_EDGE ( 'NONE', *, *, #41215, .T. ) ;
#231384=VECTOR ( 'NONE', #108833, 1000.000000000000000 ) ;
#231390=( GEOMETRIC_REPRESENTATION_CONTEXT ( 3 ) GLOBAL_UNCERTAINTY_ASSIGNED_CONTEXT ( ( #110345 ) ) GLOBAL_UNIT_ASSIGNED_CONTEXT ( ( #71424, #106652, #68855 ) ) REPRESENTATION_CONTEXT ( 'NONE', 'WORKASPACE' ) );
#231397=CARTESIAN_POINT ( 'NONE',  ( -20.90000000000000213, 8.000000000000000000, 1.212568896937007867 ) ) ;
#231407=EDGE_LOOP ( 'NONE', ( #14556, #218300, #240494, #28791 ) ) ;
#231449=CARTESIAN_POINT ( 'NONE',  ( 18.79999999999999716, 0.000000000000000000, 0.000000000000000000 ) ) ;
#231559=DIRECTION ( 'NONE',  ( 0.000000000000000000, -1.776356839400250465E-15, -1.000000000000000000 ) ) ;
#231568=AXIS2_PLACEMENT_3D ( 'NONE', #92174, #246127, #54322 ) ;
#231581=ORIENTED_EDGE ( 'NONE', *, *, #104855, .T. ) ;
#231594=TOROIDAL_SURFACE ( 'NONE', #135890, 0.2000000000000000111, 0.1000000000000000056 ) ;
#231639=FACE_OUTER_BOUND ( 'NONE', #229936, .T. ) ;
#231685=ORIENTED_EDGE ( 'NONE', *, *, #23683, .T. ) ;
#231709=CARTESIAN_POINT ( 'NONE',  ( -18.69999999999999929, -11.65000000000000036, 6.000000000000001776 ) ) ;
#231748=ORIENTED_EDGE ( 'NONE', *, *, #87223, .T. ) ;
#231790=ORIENTED_EDGE ( 'NONE', *, *, #36092, .F. ) ;
#231811=DIRECTION ( 'NONE',  ( 0.000000000000000000, 0.000000000000000000, 1.000000000000000000 ) ) ;
#231879=CARTESIAN_POINT ( 'NONE',  ( -22.19999999999999929, -11.65000000000000036, 17.70000000000000639 ) ) ;
#231883=CARTESIAN_POINT ( 'NONE',  ( -6.000000000000003553, -11.34999999999999964, 10.00000000000000178 ) ) ;
#231885=DIRECTION ( 'NONE',  ( 1.000000000000000000, 0.000000000000000000, 0.000000000000000000 ) ) ;
#231900=CARTESIAN_POINT ( 'NONE',  ( -18.69999999999999929, -8.250000000000005329, 30.10000000000000142 ) ) ;
#231925=ORIENTED_EDGE ( 'NONE', *, *, #46105, .T. ) ;
#231941=AXIS2_PLACEMENT_3D ( 'NONE', #150719, #109003, #228976 ) ;
#231944=DIRECTION ( 'NONE',  ( 0.000000000000000000, 0.000000000000000000, -1.000000000000000000 ) ) ;
#231964=EDGE_CURVE ( 'NONE', #186764, #135547, #95439, .T. ) ;
#232125=DIRECTION ( 'NONE',  ( 0.000000000000000000, 4.336808689942043768E-15, -1.000000000000000000 ) ) ;
#232131=CARTESIAN_POINT ( 'NONE',  ( 20.89999999999999503, -1.212568896937008089, -8.000000000000000000 ) ) ;
#232161=AXIS2_PLACEMENT_3D ( 'NONE', #98822, #59710, #2307 ) ;
#232224=DIRECTION ( 'NONE',  ( 0.000000000000000000, 0.000000000000000000, -1.000000000000000000 ) ) ;
#232230=DIRECTION ( 'NONE',  ( -1.000000000000000000, -0.000000000000000000, 0.000000000000000000 ) ) ;
#232241=AXIS2_PLACEMENT_3D ( 'NONE', #104534, #65437, #224511 ) ;
#232249=DIRECTION ( 'NONE',  ( 0.000000000000000000, -1.000000000000000000, -0.000000000000000000 ) ) ;
#232298=ORIENTED_EDGE ( 'NONE', *, *, #80296, .F. ) ;
#232404=ORIENTED_EDGE ( 'NONE', *, *, #39528, .F. ) ;
#232423=CARTESIAN_POINT ( 'NONE',  ( 18.79999999999999716, -1.467286812112899463, 28.00000000000000000 ) ) ;
#232428=DIRECTION ( 'NONE',  ( -0.000000000000000000, -0.9910465087640860649, -0.1335171055202901413 ) ) ;
#232450=CARTESIAN_POINT ( 'NONE',  ( 13.40000000000000036, -8.250000000000005329, 10.95857864376269575 ) ) ;
#232501=CARTESIAN_POINT ( 'NONE',  ( -18.79999999999999716, 3.461118860469513336, 28.84309995045515507 ) ) ;
#232547=VERTEX_POINT ( 'NONE', #106665 ) ;
#232552=CARTESIAN_POINT ( 'NONE',  ( -37.88850191057539973, 11.75000000000000000, 30.00000000000000000 ) ) ;
#232573=ORIENTED_EDGE ( 'NONE', *, *, #196466, .F. ) ;
#232592=DIRECTION ( 'NONE',  ( 1.000000000000000000, -0.000000000000000000, 0.000000000000000000 ) ) ;
#232598=DIRECTION ( 'NONE',  ( 1.000000000000000000, -0.000000000000000000, 0.000000000000000000 ) ) ;
#232605=CARTESIAN_POINT ( 'NONE',  ( 18.79999999999999361, -11.65000000000000036, 30.09999999999999787 ) ) ;
#232669=ORIENTED_EDGE ( 'NONE', *, *, #246009, .T. ) ;
#232693=AXIS2_PLACEMENT_3D ( 'NONE', #20889, #239919, #46815 ) ;
#232708=ORIENTED_EDGE ( 'NONE', *, *, #74921, .F. ) ;
#232727=DIRECTION ( 'NONE',  ( 2.933373889701419960E-15, -0.8164989248600479366, 0.5773469543544730298 ) ) ;
#232735=DIRECTION ( 'NONE',  ( -1.000000000000000000, 0.000000000000000000, 0.000000000000000000 ) ) ;
#232754=ADVANCED_FACE ( 'NONE', ( #98632 ), #256398, .T. ) ;
#232779=EDGE_CURVE ( 'NONE', #89072, #58688, #183170, .T. ) ;
#232793=ADVANCED_FACE ( 'NONE', ( #243310 ), #12492, .F. ) ;
#232803=CARTESIAN_POINT ( 'NONE',  ( -18.79999999999999716, -11.65000000000000036, -15.00000000000000000 ) ) ;
#232809=CARTESIAN_POINT ( 'NONE',  ( -11.60000000000000320, -11.75000000000000000, 15.00000000000000355 ) ) ;
#232863=LINE ( 'NONE', #238958, #137218 ) ;
#232873=CARTESIAN_POINT ( 'NONE',  ( 21.10000000000000142, 0.000000000000000000, 0.000000000000000000 ) ) ;
#232875=TOROIDAL_SURFACE ( 'NONE', #128815, 4.041421356237312246, 0.1000000000000000056 ) ;
#232913=DIRECTION ( 'NONE',  ( 0.000000000000000000, 0.000000000000000000, 1.000000000000000000 ) ) ;
#232939=DIRECTION ( 'NONE',  ( 0.000000000000000000, 0.000000000000000000, -1.000000000000000000 ) ) ;
#232965=CARTESIAN_POINT ( 'NONE',  ( -22.19999999999999929, -11.75000000000000000, 9.900000000000002132 ) ) ;
#232968=EDGE_LOOP ( 'NONE', ( #170674, #143284, #184796, #74920 ) ) ;
#233015=EDGE_CURVE ( 'NONE', #66395, #245624, #29079, .T. ) ;
#233016=DIRECTION ( 'NONE',  ( -0.000000000000000000, -0.1335171055202901413, 0.9910465087640860649 ) ) ;
#233025=VERTEX_POINT ( 'NONE', #33302 ) ;
#233049=FACE_OUTER_BOUND ( 'NONE', #63932, .T. ) ;
#233052=CIRCLE ( 'NONE', #78877, 0.1000000000000028644 ) ;
#233063=AXIS2_PLACEMENT_3D ( 'NONE', #173481, #116030, #211267 ) ;
#233101=EDGE_LOOP ( 'NONE', ( #112795, #244157, #82209, #251899 ) ) ;
#233102=CARTESIAN_POINT ( 'NONE',  ( 18.79999999999999716, 1.350000000000000089, 16.50000000000000000 ) ) ;
#233144=ORIENTED_EDGE ( 'NONE', *, *, #124514, .F. ) ;
#233154=VERTEX_POINT ( 'NONE', #123079 ) ;
#233164=DIRECTION ( 'NONE',  ( -1.000000000000000000, 0.000000000000000000, 0.000000000000000000 ) ) ;
#233182=CARTESIAN_POINT ( 'NONE',  ( -21.10000000000000142, -11.75000000000000000, 11.89999999999999680 ) ) ;
#233217=ORIENTED_EDGE ( 'NONE', *, *, #229921, .F. ) ;
#233241=EDGE_CURVE ( 'NONE', #104540, #237894, #129187, .T. ) ;
#233243=CARTESIAN_POINT ( 'NONE',  ( 0.000000000000000000, -8.350000000000004974, 33.00000000000000000 ) ) ;
#233266=DIRECTION ( 'NONE',  ( 1.000000000000000000, 0.000000000000000000, 0.000000000000000000 ) ) ;
#233271=ORIENTED_EDGE ( 'NONE', *, *, #122454, .T. ) ;
#233286=DIRECTION ( 'NONE',  ( -0.000000000000000000, 1.000000000000000000, -0.000000000000000000 ) ) ;
#233334=AXIS2_PLACEMENT_3D ( 'NONE', #245102, #23525, #61332 ) ;
#233371=DIRECTION ( 'NONE',  ( 0.000000000000000000, -1.000000000000000000, 0.000000000000000000 ) ) ;
#233408=EDGE_CURVE ( 'NONE', #114614, #248722, #200704, .T. ) ;
#233413=CARTESIAN_POINT ( 'NONE',  ( 19.90000000000000568, 1.350000000000000089, 21.90000000000000213 ) ) ;
#233420=DIRECTION ( 'NONE',  ( 0.000000000000000000, 0.000000000000000000, -1.000000000000000000 ) ) ;
#233441=VECTOR ( 'NONE', #1279, 1000.000000000000000 ) ;
#233451=DIRECTION ( 'NONE',  ( 0.000000000000000000, 0.000000000000000000, -1.000000000000000000 ) ) ;
#233456=DIRECTION ( 'NONE',  ( 0.000000000000000000, -0.4856429311786307212, -0.8741572761215384846 ) ) ;
#233531=TOROIDAL_SURFACE ( 'NONE', #121119, 11.65000000000000036, 0.1000000000000000056 ) ;
#233549=EDGE_CURVE ( 'NONE', #204755, #248722, #58416, .T. ) ;
#233559=CYLINDRICAL_SURFACE ( 'NONE', #126851, 0.09999999999999982514 ) ;
#233604=ORIENTED_EDGE ( 'NONE', *, *, #127815, .T. ) ;
#233690=ADVANCED_FACE ( 'NONE', ( #106711 ), #84550, .T. ) ;
#233704=EDGE_CURVE ( 'NONE', #122006, #176334, #175199, .T. ) ;
#233706=DIRECTION ( 'NONE',  ( 0.000000000000000000, 1.000000000000000000, 0.000000000000000000 ) ) ;
#233712=DIRECTION ( 'NONE',  ( 0.000000000000000000, -8.881784197001252323E-16, 1.000000000000000000 ) ) ;
#233727=VECTOR ( 'NONE', #222846, 1000.000000000000000 ) ;
#233780=CARTESIAN_POINT ( 'NONE',  ( 18.79999999999999716, 11.61130914238355771, 16.50000000000000000 ) ) ;
#233781=CARTESIAN_POINT ( 'NONE',  ( -18.69999999999999929, 1.149999999999999911, 21.90000000000000213 ) ) ;
#233784=EDGE_CURVE ( 'NONE', #89234, #132961, #241783, .T. ) ;
#233816=DIRECTION ( 'NONE',  ( 0.000000000000000000, 0.000000000000000000, -1.000000000000000000 ) ) ;
#233831=DIRECTION ( 'NONE',  ( 0.000000000000000000, -0.7071067811865472397, -0.7071067811865479058 ) ) ;
#233873=CIRCLE ( 'NONE', #238137, 0.09999999999999990841 ) ;
#233906=EDGE_CURVE ( 'NONE', #86293, #243012, #200099, .T. ) ;
#233948=DIRECTION ( 'NONE',  ( 0.000000000000000000, 1.000000000000000000, -0.000000000000000000 ) ) ;
#233972=CARTESIAN_POINT ( 'NONE',  ( -19.99999999999999645, 11.61130914238355771, 16.50000000000000000 ) ) ;
#234000=EDGE_LOOP ( 'NONE', ( #19161, #84647, #246552, #246844 ) ) ;
#234024=ORIENTED_EDGE ( 'NONE', *, *, #205126, .T. ) ;
#234031=EDGE_LOOP ( 'NONE', ( #68151, #69445, #11905, #109197 ) ) ;
#234077=VERTEX_POINT ( 'NONE', #193668 ) ;
#234136=LINE ( 'NONE', #157206, #197531 ) ;
#234148=ORIENTED_EDGE ( 'NONE', *, *, #176352, .F. ) ;
#234167=ORIENTED_EDGE ( 'NONE', *, *, #240221, .F. ) ;
#234177=ORIENTED_EDGE ( 'NONE', *, *, #4267, .F. ) ;
#234208=EDGE_CURVE ( 'NONE', #63429, #128297, #29618, .T. ) ;
#234236=CARTESIAN_POINT ( 'NONE',  ( 11.60000000000000320, -11.65000000000000036, 17.60000000000000497 ) ) ;
#234240=ORIENTED_EDGE ( 'NONE', *, *, #50449, .F. ) ;
#234263=ORIENTED_EDGE ( 'NONE', *, *, #51116, .T. ) ;
#234275=DIRECTION ( 'NONE',  ( 0.000000000000000000, 0.000000000000000000, -1.000000000000000000 ) ) ;
#234276=DIRECTION ( 'NONE',  ( 0.000000000000000000, 0.9856811345164832039, 0.1686199900910280158 ) ) ;
#234330=DIRECTION ( 'NONE',  ( 1.000000000000000000, 0.000000000000000000, -0.000000000000000000 ) ) ;
#234361=EDGE_CURVE ( 'NONE', #45068, #186207, #143948, .T. ) ;
#234376=EDGE_CURVE ( 'NONE', #67858, #75809, #142652, .T. ) ;
#234386=CARTESIAN_POINT ( 'NONE',  ( -21.00000000000000000, 6.239477252822117848, 11.95447128030241579 ) ) ;
#234392=DIRECTION ( 'NONE',  ( -0.000000000000000000, 1.000000000000000000, 0.000000000000000000 ) ) ;
#234409=AXIS2_PLACEMENT_3D ( 'NONE', #55504, #178081, #256236 ) ;
#234426=CARTESIAN_POINT ( 'NONE',  ( -18.70000000000000639, -9.849999999999994316, 30.00000000000000000 ) ) ;
#234431=ADVANCED_FACE ( 'NONE', ( #180527 ), #42295, .T. ) ;
#234454=DIRECTION ( 'NONE',  ( -1.476360405086644309E-16, 1.000000000000000000, 1.445602896647339410E-16 ) ) ;
#234470=CARTESIAN_POINT ( 'NONE',  ( 18.59999999999999787, -10.64999999999999325, 31.39999999999999858 ) ) ;
#234472=DIRECTION ( 'NONE',  ( -0.000000000000000000, 0.1335171055202901691, 0.9910465087640861759 ) ) ;
#234479=CARTESIAN_POINT ( 'NONE',  ( 22.94999999999999929, 0.000000000000000000, 0.000000000000000000 ) ) ;
#234493=DIRECTION ( 'NONE',  ( -0.000000000000000000, 0.000000000000000000, 1.000000000000000000 ) ) ;
#234520=EDGE_CURVE ( 'NONE', #163777, #167847, #242138, .T. ) ;
#234542=EDGE_CURVE ( 'NONE', #130397, #217842, #13219, .T. ) ;
#234580=ORIENTED_EDGE ( 'NONE', *, *, #191182, .T. ) ;
#234638=VECTOR ( 'NONE', #67997, 1000.000000000000000 ) ;
#234650=DIRECTION ( 'NONE',  ( -1.000000000000000000, 0.000000000000000000, 0.000000000000000000 ) ) ;
#234657=CIRCLE ( 'NONE', #188863, 0.1999999999999987899 ) ;
#234692=CYLINDRICAL_SURFACE ( 'NONE', #99421, 0.09999999999999939493 ) ;
#234765=ORIENTED_EDGE ( 'NONE', *, *, #99529, .T. ) ;
#234815=AXIS2_PLACEMENT_3D ( 'NONE', #26976, #106449, #186018 ) ;
#234816=AXIS2_PLACEMENT_3D ( 'NONE', #211416, #134416, #52314 ) ;
#234838=ORIENTED_EDGE ( 'NONE', *, *, #117869, .T. ) ;
#234847=AXIS2_PLACEMENT_3D ( 'NONE', #188883, #31132, #87189 ) ;
#234848=AXIS2_PLACEMENT_3D ( 'NONE', #40639, #187502, #64010 ) ;
#234852=ADVANCED_FACE ( 'NONE', ( #61920 ), #180583, .T. ) ;
#234857=ORIENTED_EDGE ( 'NONE', *, *, #99118, .T. ) ;
#234859=FACE_OUTER_BOUND ( 'NONE', #174612, .T. ) ;
#234925=ORIENTED_EDGE ( 'NONE', *, *, #2924, .T. ) ;
#234976=CARTESIAN_POINT ( 'NONE',  ( -11.60000000000000320, -8.279289321881348584, 11.02928932188134503 ) ) ;
#234985=ORIENTED_EDGE ( 'NONE', *, *, #152304, .T. ) ;
#234997=CARTESIAN_POINT ( 'NONE',  ( 18.79999999999999716, 7.973296578895943121, 1.410778198689824903 ) ) ;
#235024=CARTESIAN_POINT ( 'NONE',  ( 20.90000000000000213, 11.61130914238355771, -1.800000000000000044 ) ) ;
#235071=LINE ( 'NONE', #139792, #149285 ) ;
#235115=ORIENTED_EDGE ( 'NONE', *, *, #205032, .T. ) ;
#235127=CARTESIAN_POINT ( 'NONE',  ( 11.60000000000000142, -11.65000000000000036, 12.30000000000000426 ) ) ;
#235142=CYLINDRICAL_SURFACE ( 'NONE', #89507, 0.1000000000000002554 ) ;
#235149=DIRECTION ( 'NONE',  ( -1.000000000000000000, 0.000000000000000000, 0.000000000000000000 ) ) ;
#235151=AXIS2_PLACEMENT_3D ( 'NONE', #31828, #153074, #151769 ) ;
#235159=CARTESIAN_POINT ( 'NONE',  ( -22.19999999999999929, -11.65000000000000036, 14.10000000000000142 ) ) ;
#235214=ORIENTED_EDGE ( 'NONE', *, *, #193902, .F. ) ;
#235235=CARTESIAN_POINT ( 'NONE',  ( -19.89999999999999858, 5.488301202077012775, 16.50000000000000000 ) ) ;
#235256=DIRECTION ( 'NONE',  ( 0.000000000000000000, 0.000000000000000000, 1.000000000000000000 ) ) ;
#235316=VECTOR ( 'NONE', #220704, 1000.000000000000000 ) ;
#235380=ORIENTED_EDGE ( 'NONE', *, *, #46749, .T. ) ;
#235387=CARTESIAN_POINT ( 'NONE',  ( 18.79999999999999716, 0.000000000000000000, 0.000000000000000000 ) ) ;
#235390=VERTEX_POINT ( 'NONE', #225794 ) ;
#235447=AXIS2_PLACEMENT_3D ( 'NONE', #39285, #77093, #12337 ) ;
#235458=STYLED_ITEM ( 'NONE', ( #152252 ), #144814 ) ;
#235465=CARTESIAN_POINT ( 'NONE',  ( 20.90000000000000213, 1.212568896937007645, -8.000000000000000000 ) ) ;
#235508=AXIS2_PLACEMENT_3D ( 'NONE', #57042, #216139, #45208 ) ;
#235534=CARTESIAN_POINT ( 'NONE',  ( -20.90000000000000213, 11.49641995933507843, 1.885425182446133885 ) ) ;
#235582=CARTESIAN_POINT ( 'NONE',  ( 5.899999999999996803, -11.65000000000000036, 14.10000000000000142 ) ) ;
#235614=EDGE_CURVE ( 'NONE', #144975, #71927, #236086, .T. ) ;
#235615=DIRECTION ( 'NONE',  ( 1.462545276649423285E-15, 0.1686199900910279881, -0.9856811345164833149 ) ) ;
#235678=FACE_OUTER_BOUND ( 'NONE', #92478, .T. ) ;
#235772=CARTESIAN_POINT ( 'NONE',  ( -18.69999999999999929, 1.149999999999999911, -15.00000000000000000 ) ) ;
#235814=CARTESIAN_POINT ( 'NONE',  ( -18.79999999999999716, 10.31653824539117714, -11.82383137372478110 ) ) ;
#235821=AXIS2_PLACEMENT_3D ( 'NONE', #45826, #203617, #184049 ) ;
#235861=DIRECTION ( 'NONE',  ( -1.000000000000000000, 0.000000000000000000, -0.000000000000000000 ) ) ;
#235978=DIRECTION ( 'NONE',  ( 0.000000000000000000, -0.000000000000000000, 1.000000000000000000 ) ) ;
#235983=EDGE_CURVE ( 'NONE', #78394, #216154, #33777, .T. ) ;
#236004=DIRECTION ( 'NONE',  ( 1.000000000000000000, -8.673617379884087537E-15, -0.000000000000000000 ) ) ;
#236010=AXIS2_PLACEMENT_3D ( 'NONE', #97115, #35923, #254884 ) ;
#236033=EDGE_CURVE ( 'NONE', #216154, #22402, #161391, .T. ) ;
#236086=LINE ( 'NONE', #256884, #200915 ) ;
#236102=CARTESIAN_POINT ( 'NONE',  ( 13.40000000000000036, -8.279289321881350361, 11.02928932188135036 ) ) ;
#236189=AXIS2_PLACEMENT_3D ( 'NONE', #154879, #171885, #251375 ) ;
#236214=EDGE_CURVE ( 'NONE', #57087, #126102, #43229, .T. ) ;
#236229=AXIS2_PLACEMENT_3D ( 'NONE', #47478, #26676, #10954 ) ;
#236240=DIRECTION ( 'NONE',  ( 0.000000000000000000, 0.000000000000000000, 1.000000000000000000 ) ) ;
#236245=TOROIDAL_SURFACE ( 'NONE', #102958, 4.100000000000000533, 0.1000000000000000056 ) ;
#236248=EDGE_CURVE ( 'NONE', #156269, #92927, #218163, .T. ) ;
#236258=CARTESIAN_POINT ( 'NONE',  ( -20.90000000000000213, 0.000000000000000000, 0.000000000000000000 ) ) ;
#236294=ADVANCED_FACE ( 'NONE', ( #150796 ), #92101, .T. ) ;
#236379=DIRECTION ( 'NONE',  ( 1.000000000000000000, 0.000000000000000000, 0.000000000000000000 ) ) ;
#236402=FACE_OUTER_BOUND ( 'NONE', #152803, .T. ) ;
#236407=CYLINDRICAL_SURFACE ( 'NONE', #173748, 0.09999999999999939493 ) ;
#236410=ORIENTED_EDGE ( 'NONE', *, *, #74431, .T. ) ;
#236459=VERTEX_POINT ( 'NONE', #229715 ) ;
#236462=AXIS2_PLACEMENT_3D ( 'NONE', #39540, #177758, #156915 ) ;
#236465=ORIENTED_EDGE ( 'NONE', *, *, #149758, .T. ) ;
#236481=ORIENTED_EDGE ( 'NONE', *, *, #15944, .F. ) ;
#236515=EDGE_CURVE ( 'NONE', #125866, #25377, #60143, .T. ) ;
#236616=ADVANCED_FACE ( 'NONE', ( #74539 ), #117477, .T. ) ;
#236743=EDGE_CURVE ( 'NONE', #1224, #36331, #22949, .T. ) ;
#236790=CARTESIAN_POINT ( 'NONE',  ( -11.60000000000000320, -9.650000000000005684, 15.00000000000000355 ) ) ;
#236800=ORIENTED_EDGE ( 'NONE', *, *, #132175, .F. ) ;
#236817=CARTESIAN_POINT ( 'NONE',  ( -18.79999999999999716, -1.885425182446133885, -11.59641995933507808 ) ) ;
#236836=DIRECTION ( 'NONE',  ( -1.000000000000000000, 0.000000000000000000, -0.000000000000000000 ) ) ;
#236848=ADVANCED_FACE ( 'NONE', ( #127750 ), #122894, .T. ) ;
#236869=CARTESIAN_POINT ( 'NONE',  ( -13.40000000000000036, -11.65000000000000036, 12.30000000000000426 ) ) ;
#236892=CIRCLE ( 'NONE', #153562, 0.09999999999999939493 ) ;
#236899=CARTESIAN_POINT ( 'NONE',  ( -20.90000000000000213, 1.212568896937007645, -8.000000000000000000 ) ) ;
#236910=LINE ( 'NONE', #140370, #85221 ) ;
#236956=DIRECTION ( 'NONE',  ( 0.000000000000000000, 0.000000000000000000, 1.000000000000000000 ) ) ;
#236973=CYLINDRICAL_SURFACE ( 'NONE', #207988, 0.1000000000000028644 ) ;
#237013=CARTESIAN_POINT ( 'NONE',  ( -22.94999999999999929, 1.212568896937007645, -8.000000000000000000 ) ) ;
#237014=EDGE_CURVE ( 'NONE', #3738, #72694, #131587, .T. ) ;
#237040=CIRCLE ( 'NONE', #24867, 0.09999999999999939493 ) ;
#237049=CARTESIAN_POINT ( 'NONE',  ( 18.79999999999999716, 6.841561409100513025, 9.675512259591560138 ) ) ;
#237103=DIRECTION ( 'NONE',  ( 0.000000000000000000, 0.9868171638914228216, 0.1618390714546044939 ) ) ;
#237134=ORIENTED_EDGE ( 'NONE', *, *, #215541, .F. ) ;
#237138=DIRECTION ( 'NONE',  ( 0.000000000000000000, 0.000000000000000000, -1.000000000000000000 ) ) ;
#237247=CYLINDRICAL_SURFACE ( 'NONE', #41910, 0.1000000000000002554 ) ;
#237264=EDGE_CURVE ( 'NONE', #163484, #120569, #139260, .T. ) ;
#237271=CYLINDRICAL_SURFACE ( 'NONE', #125688, 0.09999999999999939493 ) ;
#237289=DIRECTION ( 'NONE',  ( 0.000000000000000000, 0.1618390714546044939, -0.9868171638914228216 ) ) ;
#237310=EDGE_CURVE ( 'NONE', #169022, #36888, #25758, .T. ) ;
#237382=CYLINDRICAL_SURFACE ( 'NONE', #164220, 0.09999999999999933942 ) ;
#237407=CARTESIAN_POINT ( 'NONE',  ( 18.69999999999999929, 1.350000000000000089, 16.60000000000000142 ) ) ;
#237409=DIRECTION ( 'NONE',  ( 0.000000000000000000, 0.000000000000000000, 1.000000000000000000 ) ) ;
#237415=CIRCLE ( 'NONE', #166517, 0.09999999999999939493 ) ;
#237435=ORIENTED_EDGE ( 'NONE', *, *, #161141, .F. ) ;
#237492=DIRECTION ( 'NONE',  ( 1.000000000000000000, 0.000000000000000000, 0.000000000000000000 ) ) ;
#237505=CARTESIAN_POINT ( 'NONE',  ( 11.60000000000000142, -8.279289321881350361, 11.02928932188135036 ) ) ;
#237555=DIRECTION ( 'NONE',  ( 0.000000000000000000, 1.000000000000000000, -0.000000000000000000 ) ) ;
#237569=EDGE_CURVE ( 'NONE', #171566, #223079, #202359, .T. ) ;
#237590=CARTESIAN_POINT ( 'NONE',  ( -19.89999999999999858, 5.488301202077012775, 16.50000000000000000 ) ) ;
#237614=DIRECTION ( 'NONE',  ( 1.000000000000000000, -0.000000000000000000, -0.000000000000000000 ) ) ;
#237636=DIRECTION ( 'NONE',  ( 0.000000000000000000, 0.1335171055202867274, 0.9910465087640866200 ) ) ;
#237645=DIRECTION ( 'NONE',  ( 1.000000000000000000, 0.000000000000000000, 0.000000000000000000 ) ) ;
#237672=FACE_OUTER_BOUND ( 'NONE', #218328, .T. ) ;
#237696=AXIS2_PLACEMENT_3D ( 'NONE', #53174, #191442, #91020 ) ;
#237698=VECTOR ( 'NONE', #97387, 1000.000000000000000 ) ;
#237717=CARTESIAN_POINT ( 'NONE',  ( 0.8999999999999992450, -8.350000000000004974, 30.04142135623731136 ) ) ;
#237743=DIRECTION ( 'NONE',  ( 1.000000000000000000, 0.000000000000000000, 0.000000000000000000 ) ) ;
#237749=CYLINDRICAL_SURFACE ( 'NONE', #164828, 0.1000000000000028644 ) ;
#237764=ADVANCED_FACE ( 'NONE', ( #162410 ), #187115, .F. ) ;
#237830=ORIENTED_EDGE ( 'NONE', *, *, #157054, .T. ) ;
#237845=ADVANCED_FACE ( 'NONE', ( #28916 ), #108408, .T. ) ;
#237894=VERTEX_POINT ( 'NONE', #247904 ) ;
#237898=CARTESIAN_POINT ( 'NONE',  ( -18.79999999999999716, 4.513204987021268266, 22.10000000000000142 ) ) ;
#237916=DIRECTION ( 'NONE',  ( -1.000000000000000000, 0.000000000000000000, 0.000000000000000000 ) ) ;
#237922=DIRECTION ( 'NONE',  ( 0.000000000000000000, 0.1335171055202901691, -0.9910465087640861759 ) ) ;
#237926=DIRECTION ( 'NONE',  ( 0.000000000000000000, 0.000000000000000000, 1.000000000000000000 ) ) ;
#237971=DIRECTION ( 'NONE',  ( 1.000000000000000000, 0.000000000000000000, 0.000000000000000000 ) ) ;
#237979=ORIENTED_EDGE ( 'NONE', *, *, #127127, .F. ) ;
#237991=CARTESIAN_POINT ( 'NONE',  ( 20.90000000000000213, 1.885425182446133885, -11.49641995933507843 ) ) ;
#237994=CIRCLE ( 'NONE', #46456, 0.1000000000000028644 ) ;
#238063=LINE ( 'NONE', #196372, #230296 ) ;
#238077=EDGE_LOOP ( 'NONE', ( #140191, #195459, #123427, #243810 ) ) ;
#238117=DIRECTION ( 'NONE',  ( 1.000000000000000000, 0.000000000000000000, 0.000000000000000000 ) ) ;
#238137=AXIS2_PLACEMENT_3D ( 'NONE', #95599, #116462, #59007 ) ;
#238170=DIRECTION ( 'NONE',  ( -1.000000000000000000, 0.000000000000000000, 0.000000000000000000 ) ) ;
#238198=CARTESIAN_POINT ( 'NONE',  ( 20.00000000000000355, 5.472724050409166985, 16.54552871969762506 ) ) ;
#238223=DIRECTION ( 'NONE',  ( -1.000000000000000000, 0.000000000000000000, 0.000000000000000000 ) ) ;
#238224=DIRECTION ( 'NONE',  ( 0.000000000000000000, -1.000000000000000000, 0.000000000000000000 ) ) ;
#238239=ORIENTED_EDGE ( 'NONE', *, *, #212472, .F. ) ;
#238273=AXIS2_PLACEMENT_3D ( 'NONE', #35910, #134954, #256146 ) ;
#238332=ORIENTED_EDGE ( 'NONE', *, *, #94194, .F. ) ;
#238387=CARTESIAN_POINT ( 'NONE',  ( 0.8999999999999993561, -9.650000000000003908, 26.00000000000000355 ) ) ;
#238394=VERTEX_POINT ( 'NONE', #98051 ) ;
#238396=AXIS2_PLACEMENT_3D ( 'NONE', #212515, #233371, #255416 ) ;
#238411=CIRCLE ( 'NONE', #212907, 0.1000000000000028644 ) ;
#238419=PLANE ( 'NONE',  #170067 ) ;
#238424=CARTESIAN_POINT ( 'NONE',  ( 19.90000000000000568, 1.350000000000000089, 21.90000000000000213 ) ) ;
#238570=CIRCLE ( 'NONE', #42945, 4.100000000000000533 ) ;
#238597=CIRCLE ( 'NONE', #209958, 0.1000000000000001860 ) ;
#238605=LINE ( 'NONE', #3847, #26747 ) ;
#238609=ORIENTED_EDGE ( 'NONE', *, *, #207301, .T. ) ;
#238612=AXIS2_PLACEMENT_3D ( 'NONE', #250537, #11958, #95324 ) ;
#238656=ORIENTED_EDGE ( 'NONE', *, *, #226217, .T. ) ;
#238686=DIRECTION ( 'NONE',  ( 0.000000000000000000, 1.000000000000000000, -0.000000000000000000 ) ) ;
#238692=VECTOR ( 'NONE', #108825, 1000.000000000000000 ) ;
#238700=VECTOR ( 'NONE', #21695, 1000.000000000000000 ) ;
#238703=CYLINDRICAL_SURFACE ( 'NONE', #180759, 0.09999999999999939493 ) ;
#238750=TOROIDAL_SURFACE ( 'NONE', #30482, 3.900000000000000355, 0.1000000000000000056 ) ;
#238898=CARTESIAN_POINT ( 'NONE',  ( 18.69999999999999929, 11.75000000000000000, -7.800000000000000711 ) ) ;
#238941=AXIS2_PLACEMENT_3D ( 'NONE', #255981, #57816, #156964 ) ;
#238951=ADVANCED_FACE ( 'NONE', ( #202027 ), #23418, .T. ) ;
#238958=CARTESIAN_POINT ( 'NONE',  ( -18.59999999999999787, 11.75000000000000000, 6.000000000000001776 ) ) ;
#238976=AXIS2_PLACEMENT_3D ( 'NONE', #137541, #41053, #16351 ) ;
#239005=CARTESIAN_POINT ( 'NONE',  ( -18.69999999999999929, 6.726092018229619995, 9.512212474619552438 ) ) ;
#239033=ORIENTED_EDGE ( 'NONE', *, *, #249269, .F. ) ;
#239058=ADVANCED_FACE ( 'NONE', ( #125064 ), #99040, .T. ) ;
#239121=CARTESIAN_POINT ( 'NONE',  ( -5.900000000000003020, -11.25000000000000000, 10.10000000000000142 ) ) ;
#239132=CIRCLE ( 'NONE', #209932, 0.2000000000000005107 ) ;
#239238=EDGE_CURVE ( 'NONE', #14935, #105944, #17927, .T. ) ;
#239244=ADVANCED_FACE ( 'NONE', ( #92338 ), #213563, .T. ) ;
#239246=ORIENTED_EDGE ( 'NONE', *, *, #112527, .F. ) ;
#239301=DIRECTION ( 'NONE',  ( 1.000000000000000000, 0.000000000000000000, 0.000000000000000000 ) ) ;
#239316=ADVANCED_FACE ( 'NONE', ( #93628 ), #136410, .T. ) ;
#239320=ORIENTED_EDGE ( 'NONE', *, *, #7108, .T. ) ;
#239323=CIRCLE ( 'NONE', #193541, 0.09999999999999990841 ) ;
#239451=CARTESIAN_POINT ( 'NONE',  ( -0.8999999999999993561, -11.75000000000000000, 23.30000000000000426 ) ) ;
#239478=PLANE ( 'NONE',  #138412 ) ;
#239482=EDGE_CURVE ( 'NONE', #89756, #46601, #14782, .T. ) ;
#239561=CARTESIAN_POINT ( 'NONE',  ( 18.70000000000000284, 1.350000000000000089, 22.00000000000000355 ) ) ;
#239583=ORIENTED_EDGE ( 'NONE', *, *, #3965, .F. ) ;
#239638=DIRECTION ( 'NONE',  ( 0.000000000000000000, 0.000000000000000000, 1.000000000000000000 ) ) ;
#239654=ORIENTED_EDGE ( 'NONE', *, *, #151681, .T. ) ;
#239679=DIRECTION ( 'NONE',  ( -1.000000000000000000, 0.000000000000000000, 0.000000000000000000 ) ) ;
#239715=FACE_OUTER_BOUND ( 'NONE', #153757, .T. ) ;
#239730=ORIENTED_EDGE ( 'NONE', *, *, #188393, .F. ) ;
#239732=CARTESIAN_POINT ( 'NONE',  ( -6.100000000000005862, -11.75000000000000000, 13.90000000000000213 ) ) ;
#239756=CIRCLE ( 'NONE', #147987, 2.699999999999999289 ) ;
#239767=VERTEX_POINT ( 'NONE', #206226 ) ;
#239778=ORIENTED_EDGE ( 'NONE', *, *, #158034, .T. ) ;
#239783=VERTEX_POINT ( 'NONE', #181546 ) ;
#239811=ORIENTED_EDGE ( 'NONE', *, *, #123004, .F. ) ;
#239815=EDGE_CURVE ( 'NONE', #22117, #190676, #257550, .T. ) ;
#239844=AXIS2_PLACEMENT_3D ( 'NONE', #51359, #210484, #244454 ) ;
#239891=AXIS2_PLACEMENT_3D ( 'NONE', #58910, #138452, #217990 ) ;
#239906=ORIENTED_EDGE ( 'NONE', *, *, #246009, .F. ) ;
#239919=DIRECTION ( 'NONE',  ( 1.000000000000000000, -0.000000000000000000, -0.000000000000000000 ) ) ;
#239954=ORIENTED_EDGE ( 'NONE', *, *, #9530, .F. ) ;
#240013=EDGE_LOOP ( 'NONE', ( #125742, #154588, #207583, #56890 ) ) ;
#240080=CARTESIAN_POINT ( 'NONE',  ( 20.98284271247461064, 6.322468214605803993, 12.11686199900910488 ) ) ;
#240176=AXIS2_PLACEMENT_3D ( 'NONE', #209400, #30795, #12514 ) ;
#240200=EDGE_CURVE ( 'NONE', #166243, #195496, #37073, .T. ) ;
#240221=EDGE_CURVE ( 'NONE', #83713, #75451, #88501, .T. ) ;
#240259=ORIENTED_EDGE ( 'NONE', *, *, #46193, .T. ) ;
#240280=CARTESIAN_POINT ( 'NONE',  ( 18.69999999999999574, 6.742993295648862961, 9.658650260582458458 ) ) ;
#240288=CYLINDRICAL_SURFACE ( 'NONE', #14635, 0.09999999999999939493 ) ;
#240329=DIRECTION ( 'NONE',  ( 0.000000000000000000, -0.1335171055202867274, 0.9910465087640866200 ) ) ;
#240353=DIRECTION ( 'NONE',  ( 0.000000000000000000, 0.000000000000000000, -1.000000000000000000 ) ) ;
#240386=CARTESIAN_POINT ( 'NONE',  ( 20.00894256274685645, 4.611773101055291590, 22.11686199560476140 ) ) ;
#240494=ORIENTED_EDGE ( 'NONE', *, *, #110016, .F. ) ;
#240513=AXIS2_PLACEMENT_3D ( 'NONE', #121337, #242522, #120043 ) ;
#240588=VECTOR ( 'NONE', #223218, 1000.000000000000000 ) ;
#240610=CARTESIAN_POINT ( 'NONE',  ( -13.40000000000000213, -11.75000000000000000, 17.70000000000000284 ) ) ;
#240625=ADVANCED_FACE ( 'NONE', ( #170378 ), #50348, .T. ) ;
#240628=CARTESIAN_POINT ( 'NONE',  ( 18.79999999999999716, 0.000000000000000000, 32.89999999999999858 ) ) ;
#240646=LINE ( 'NONE', #41190, #64580 ) ;
#240647=ORIENTED_EDGE ( 'NONE', *, *, #11976, .T. ) ;
#240656=EDGE_CURVE ( 'NONE', #59365, #82535, #228210, .T. ) ;
#240680=AXIS2_PLACEMENT_3D ( 'NONE', #206365, #105946, #245495 ) ;
#240713=FACE_OUTER_BOUND ( 'NONE', #137987, .T. ) ;
#240745=VERTEX_POINT ( 'NONE', #34687 ) ;
#240771=ORIENTED_EDGE ( 'NONE', *, *, #251889, .T. ) ;
#240841=DIRECTION ( 'NONE',  ( 0.000000000000000000, 1.000000000000000000, 0.000000000000000000 ) ) ;
#240930=CIRCLE ( 'NONE', #78424, 0.1000000000000028644 ) ;
#240943=DIRECTION ( 'NONE',  ( 0.000000000000000000, 0.000000000000000000, -1.000000000000000000 ) ) ;
#240962=CARTESIAN_POINT ( 'NONE',  ( -18.59999999999999787, -9.849999999999994316, 30.09999999999999787 ) ) ;
#240982=CARTESIAN_POINT ( 'NONE',  ( -18.79999999999999716, 11.49641995933507843, -1.885425182446134107 ) ) ;
#241050=ADVANCED_FACE ( 'NONE', ( #248280, #168795 ), #48786, .T. ) ;
#241083=VECTOR ( 'NONE', #7884, 1000.000000000000000 ) ;
#241156=EDGE_CURVE ( 'NONE', #79153, #14935, #95616, .T. ) ;
#241169=CARTESIAN_POINT ( 'NONE',  ( -18.79999999999999716, -1.800000000000000044, -11.61130914238355771 ) ) ;
#241175=VECTOR ( 'NONE', #33256, 1000.000000000000114 ) ;
#241189=VERTEX_POINT ( 'NONE', #52635 ) ;
#241200=CARTESIAN_POINT ( 'NONE',  ( -20.90000000000000213, 11.49641995933507843, 1.885425182446133885 ) ) ;
#241285=ORIENTED_EDGE ( 'NONE', *, *, #16669, .T. ) ;
#241288=EDGE_CURVE ( 'NONE', #149370, #142179, #144978, .T. ) ;
#241331=VECTOR ( 'NONE', #205589, 1000.000000000000000 ) ;
#241348=ORIENTED_EDGE ( 'NONE', *, *, #172509, .F. ) ;
#241363=CARTESIAN_POINT ( 'NONE',  ( -22.94999999999999929, 6.783826713665066954, 9.593862367105558064 ) ) ;
#241373=DIRECTION ( 'NONE',  ( -1.000000000000000000, 0.000000000000000000, -0.000000000000000000 ) ) ;
#241418=FACE_OUTER_BOUND ( 'NONE', #55217, .T. ) ;
#241421=EDGE_LOOP ( 'NONE', ( #115651, #63941, #18951 ) ) ;
#241425=CIRCLE ( 'NONE', #108138, 0.09999999999999939493 ) ;
#241433=LINE ( 'NONE', #22396, #217889 ) ;
#241445=CIRCLE ( 'NONE', #33369, 0.09999999999999939493 ) ;
#241472=AXIS2_PLACEMENT_3D ( 'NONE', #249127, #209992, #151312 ) ;
#241474=EDGE_LOOP ( 'NONE', ( #172860, #92499, #155302 ) ) ;
#241479=EDGE_LOOP ( 'NONE', ( #250595, #145987, #64400, #214050 ) ) ;
#241514=DIRECTION ( 'NONE',  ( 0.000000000000000000, 1.000000000000000000, 0.000000000000000000 ) ) ;
#241543=CARTESIAN_POINT ( 'NONE',  ( 18.79999999999999716, 1.212568896937007645, -7.800000000000000711 ) ) ;
#241692=ORIENTED_EDGE ( 'NONE', *, *, #182700, .F. ) ;
#241697=ADVANCED_FACE ( 'NONE', ( #249773 ), #58029, .F. ) ;
#241712=ORIENTED_EDGE ( 'NONE', *, *, #23162, .T. ) ;
#241767=CARTESIAN_POINT ( 'NONE',  ( -22.94999999999999929, 6.783826713665066954, 9.593862367105558064 ) ) ;
#241783=CIRCLE ( 'NONE', #225005, 0.09999999999999963085 ) ;
#241885=ADVANCED_FACE ( 'NONE', ( #172574 ), #109965, .F. ) ;
#241917=CARTESIAN_POINT ( 'NONE',  ( 18.59999999999999787, -9.849999999999996092, 31.39999999999999858 ) ) ;
#241945=EDGE_CURVE ( 'NONE', #16903, #247452, #195453, .T. ) ;
#241949=CARTESIAN_POINT ( 'NONE',  ( 18.59999999999999787, -9.749999999999994671, 30.09999999999999076 ) ) ;
#241973=AXIS2_PLACEMENT_3D ( 'NONE', #182331, #223993, #28416 ) ;
#242015=EDGE_CURVE ( 'NONE', #166805, #247452, #156837, .T. ) ;
#242085=ORIENTED_EDGE ( 'NONE', *, *, #144860, .F. ) ;
#242087=DIRECTION ( 'NONE',  ( 1.000000000000000000, 0.000000000000000000, 0.000000000000000000 ) ) ;
#242118=FACE_OUTER_BOUND ( 'NONE', #219883, .T. ) ;
#242119=LINE ( 'NONE', #143005, #14879 ) ;
#242125=ORIENTED_EDGE ( 'NONE', *, *, #236515, .F. ) ;
#242136=DIRECTION ( 'NONE',  ( -1.000000000000000000, 0.000000000000000000, 0.000000000000000000 ) ) ;
#242138=CIRCLE ( 'NONE', #34090, 0.09999999999999990841 ) ;
#242162=ORIENTED_EDGE ( 'NONE', *, *, #233906, .T. ) ;
#242194=DIRECTION ( 'NONE',  ( 0.000000000000000000, 0.000000000000000000, -1.000000000000000000 ) ) ;
#242238=DIRECTION ( 'NONE',  ( -0.000000000000000000, -1.000000000000000000, 0.000000000000000000 ) ) ;
#242251=CARTESIAN_POINT ( 'NONE',  ( -18.59999999999999787, -11.65000000000000036, 5.900000000000001243 ) ) ;
#242291=FACE_OUTER_BOUND ( 'NONE', #139674, .T. ) ;
#242317=CARTESIAN_POINT ( 'NONE',  ( 22.84999999999999787, 4.898587196589412829E-16, -4.000000000000000000 ) ) ;
#242362=VERTEX_POINT ( 'NONE', #249190 ) ;
#242372=CARTESIAN_POINT ( 'NONE',  ( 18.79999999999999716, 11.75000000000000000, 16.39999999999999858 ) ) ;
#242415=CARTESIAN_POINT ( 'NONE',  ( -18.79999999999999716, -1.467286812112899463, 28.00000000000000000 ) ) ;
#242445=DIRECTION ( 'NONE',  ( -0.000000000000000000, 1.000000000000000000, -0.000000000000000000 ) ) ;
#242477=AXIS2_PLACEMENT_3D ( 'NONE', #161619, #220298, #157791 ) ;
#242486=ORIENTED_EDGE ( 'NONE', *, *, #85271, .F. ) ;
#242493=AXIS2_PLACEMENT_3D ( 'NONE', #161524, #97653, #101482 ) ;
#242522=DIRECTION ( 'NONE',  ( -0.000000000000000000, -0.000000000000000000, -1.000000000000000000 ) ) ;
#242613=DIRECTION ( 'NONE',  ( -1.000000000000000000, -0.000000000000000000, -0.000000000000000000 ) ) ;
#242638=TOROIDAL_SURFACE ( 'NONE', #159278, 11.65000000000000036, 0.1000000000000000056 ) ;
#242651=DIRECTION ( 'NONE',  ( 0.000000000000000000, 0.000000000000000000, 1.000000000000000000 ) ) ;
#242698=DIRECTION ( 'NONE',  ( 0.000000000000000000, -0.1335171055202867274, -0.9910465087640865089 ) ) ;
#242748=ORIENTED_EDGE ( 'NONE', *, *, #240656, .F. ) ;
#242777=CARTESIAN_POINT ( 'NONE',  ( -18.59999999999999787, -9.849999999999942801, -15.00000000000002309 ) ) ;
#242794=CIRCLE ( 'NONE', #201275, 5.000000000000003553 ) ;
#242804=ADVANCED_FACE ( 'NONE', ( #157511 ), #136603, .F. ) ;
#242810=EDGE_CURVE ( 'NONE', #99187, #171946, #135323, .T. ) ;
#242836=CARTESIAN_POINT ( 'NONE',  ( -20.09999999999999787, 5.552655413246003313, 16.61686199900910310 ) ) ;
#242857=DIRECTION ( 'NONE',  ( 0.000000000000000000, 0.9856811345164832039, 0.1686199900910280158 ) ) ;
#242862=EDGE_CURVE ( 'NONE', #174523, #181466, #175771, .T. ) ;
#242863=AXIS2_PLACEMENT_3D ( 'NONE', #28901, #69276, #74102 ) ;
#242900=DIRECTION ( 'NONE',  ( -1.000000000000000000, 0.000000000000000000, 0.000000000000000000 ) ) ;
#242916=ORIENTED_EDGE ( 'NONE', *, *, #171175, .F. ) ;
#242918=ORIENTED_EDGE ( 'NONE', *, *, #42561, .F. ) ;
#242958=DIRECTION ( 'NONE',  ( -0.000000000000000000, 0.1686199900910313187, -0.9856811345164828708 ) ) ;
#242996=AXIS2_PLACEMENT_3D ( 'NONE', #187954, #229643, #191829 ) ;
#243012=VERTEX_POINT ( 'NONE', #26973 ) ;
#243054=EDGE_LOOP ( 'NONE', ( #252184, #172371, #92663, #86675 ) ) ;
#243055=CARTESIAN_POINT ( 'NONE',  ( -22.10000000000000497, 10.88519226655716565, -15.14794223642649840 ) ) ;
#243069=AXIS2_PLACEMENT_3D ( 'NONE', #102629, #218737, #119673 ) ;
#243116=DIRECTION ( 'NONE',  ( 0.000000000000000000, 1.000000000000000000, 0.000000000000000000 ) ) ;
#243128=ADVANCED_FACE ( 'NONE', ( #208164 ), #249842, .F. ) ;
#243141=CARTESIAN_POINT ( 'NONE',  ( 11.60000000000000142, -8.250000000000003553, 17.60000000000000497 ) ) ;
#243184=ORIENTED_EDGE ( 'NONE', *, *, #152466, .F. ) ;
#243198=ORIENTED_EDGE ( 'NONE', *, *, #20655, .F. ) ;
#243222=FACE_OUTER_BOUND ( 'NONE', #148263, .T. ) ;
#243251=EDGE_LOOP ( 'NONE', ( #16573, #77950, #30523, #150493 ) ) ;
#243300=ORIENTED_EDGE ( 'NONE', *, *, #100042, .T. ) ;
#243310=FACE_OUTER_BOUND ( 'NONE', #115831, .T. ) ;
#243313=CARTESIAN_POINT ( 'NONE',  ( -5.900000000000002132, -11.34999999999999964, 13.90000000000000213 ) ) ;
#243347=CARTESIAN_POINT ( 'NONE',  ( 18.59999999999999787, -8.350000000000004974, 33.00000000000000000 ) ) ;
#243350=CARTESIAN_POINT ( 'NONE',  ( 21.10000000000000142, -11.65000000000000036, 11.99999999999999645 ) ) ;
#243374=DIRECTION ( 'NONE',  ( -0.000000000000000000, 1.000000000000000000, -0.000000000000000000 ) ) ;
#243429=CARTESIAN_POINT ( 'NONE',  ( -18.59999999999999787, -9.849999999999990763, 31.50000000000000000 ) ) ;
#243451=ORIENTED_EDGE ( 'NONE', *, *, #11570, .F. ) ;
#243495=AXIS2_PLACEMENT_3D ( 'NONE', #1352, #43073, #78326 ) ;
#243505=AXIS2_PLACEMENT_3D ( 'NONE', #140459, #184407, #58340 ) ;
#243512=CARTESIAN_POINT ( 'NONE',  ( -19.99999999999999645, 5.572646938319271825, 16.60000000000000142 ) ) ;
#243549=FACE_OUTER_BOUND ( 'NONE', #56607, .T. ) ;
#243607=DIRECTION ( 'NONE',  ( 0.000000000000000000, 0.000000000000000000, 1.000000000000000000 ) ) ;
#243620=ORIENTED_EDGE ( 'NONE', *, *, #146470, .F. ) ;
#243637=ORIENTED_EDGE ( 'NONE', *, *, #69359, .F. ) ;
#243645=EDGE_CURVE ( 'NONE', #47981, #127870, #58695, .T. ) ;
#243676=EDGE_CURVE ( 'NONE', #214793, #189932, #121373, .T. ) ;
#243678=CARTESIAN_POINT ( 'NONE',  ( -6.000000000000003553, -11.65000000000000036, 10.00000000000000178 ) ) ;
#243682=FACE_OUTER_BOUND ( 'NONE', #69208, .T. ) ;
#243714=LINE ( 'NONE', #202025, #257330 ) ;
#243766=ORIENTED_EDGE ( 'NONE', *, *, #48190, .T. ) ;
#243810=ORIENTED_EDGE ( 'NONE', *, *, #135117, .F. ) ;
#243824=VECTOR ( 'NONE', #143289, 1000.000000000000114 ) ;
#243832=VERTEX_POINT ( 'NONE', #191535 ) ;
#243874=ORIENTED_EDGE ( 'NONE', *, *, #155762, .F. ) ;
#243876=CARTESIAN_POINT ( 'NONE',  ( -22.94999999999999929, 11.49641995933507843, 1.885425182446134107 ) ) ;
#243888=VERTEX_POINT ( 'NONE', #168138 ) ;
#243889=LINE ( 'NONE', #104361, #206643 ) ;
#243899=DIRECTION ( 'NONE',  ( 0.000000000000000000, 0.000000000000000000, -1.000000000000000000 ) ) ;
#243909=ORIENTED_EDGE ( 'NONE', *, *, #23802, .T. ) ;
#243938=DIRECTION ( 'NONE',  ( 0.000000000000000000, 0.000000000000000000, 1.000000000000000000 ) ) ;
#243954=DIRECTION ( 'NONE',  ( 1.000000000000000000, -0.000000000000000000, -0.000000000000000000 ) ) ;
#243955=DIRECTION ( 'NONE',  ( 1.000000000000000000, 0.000000000000000000, 0.000000000000000000 ) ) ;
#243962=EDGE_CURVE ( 'NONE', #29621, #66961, #96238, .T. ) ;
#243980=ORIENTED_EDGE ( 'NONE', *, *, #204758, .T. ) ;
#243984=VECTOR ( 'NONE', #153345, 1000.000000000000000 ) ;
#244004=ORIENTED_EDGE ( 'NONE', *, *, #90004, .T. ) ;
#244008=EDGE_CURVE ( 'NONE', #31617, #8702, #196520, .T. ) ;
#244023=ORIENTED_EDGE ( 'NONE', *, *, #157121, .T. ) ;
#244101=CARTESIAN_POINT ( 'NONE',  ( -20.09999999999999787, 4.645987002755569861, 21.91686199900910736 ) ) ;
#244135=CIRCLE ( 'NONE', #60978, 0.09999999999999939493 ) ;
#244144=ORIENTED_EDGE ( 'NONE', *, *, #74431, .F. ) ;
#244148=DIRECTION ( 'NONE',  ( 0.000000000000000000, -1.000000000000000000, 0.000000000000000000 ) ) ;
#244153=DIRECTION ( 'NONE',  ( -0.000000000000000000, 0.9910465087640861759, 0.1335171055202901691 ) ) ;
#244157=ORIENTED_EDGE ( 'NONE', *, *, #135523, .T. ) ;
#244165=DIRECTION ( 'NONE',  ( 0.000000000000000000, 0.000000000000000000, -1.000000000000000000 ) ) ;
#244173=CARTESIAN_POINT ( 'NONE',  ( -18.69999999999999929, 0.000000000000000000, 0.000000000000000000 ) ) ;
#244217=EDGE_LOOP ( 'NONE', ( #157863, #185630, #156319, #13002 ) ) ;
#244270=CIRCLE ( 'NONE', #127772, 0.1000000000000002554 ) ;
#244291=ADVANCED_FACE ( 'NONE', ( #93367 ), #1037, .T. ) ;
#244295=CARTESIAN_POINT ( 'NONE',  ( -21.00000000000000000, 0.000000000000000000, 4.100000000000000533 ) ) ;
#244305=CARTESIAN_POINT ( 'NONE',  ( 18.59999999999999787, -9.749999999999996447, 31.39999999999999858 ) ) ;
#244318=CARTESIAN_POINT ( 'NONE',  ( 18.79999999999999716, 11.61130914238355771, -1.800000000000000044 ) ) ;
#244320=CIRCLE ( 'NONE', #119446, 0.09999999999999939493 ) ;
#244330=CARTESIAN_POINT ( 'NONE',  ( 11.60000000000000320, -12.24999999999999822, 15.00000000000000355 ) ) ;
#244339=VERTEX_POINT ( 'NONE', #257519 ) ;
#244385=CIRCLE ( 'NONE', #231941, 0.09999999999999993616 ) ;
#244402=ORIENTED_EDGE ( 'NONE', *, *, #7442, .T. ) ;
#244437=DIRECTION ( 'NONE',  ( 0.000000000000000000, 0.000000000000000000, -1.000000000000000000 ) ) ;
#244454=DIRECTION ( 'NONE',  ( 1.000000000000000000, 0.000000000000000000, 0.000000000000000000 ) ) ;
#244527=AXIS2_PLACEMENT_3D ( 'NONE', #56767, #192467, #210743 ) ;
#244548=DIRECTION ( 'NONE',  ( -1.000000000000000000, 0.000000000000000000, 0.000000000000000000 ) ) ;
#244551=FACE_BOUND ( 'NONE', #139722, .T. ) ;
#244578=AXIS2_PLACEMENT_3D ( 'NONE', #93544, #235615, #72738 ) ;
#244615=AXIS2_PLACEMENT_3D ( 'NONE', #169301, #248806, #70186 ) ;
#244632=DIRECTION ( 'NONE',  ( 0.000000000000000000, -0.1686199900910312910, 0.9856811345164826488 ) ) ;
#244697=DIRECTION ( 'NONE',  ( 0.000000000000000000, 0.9856811345164827598, 0.1686199900910313187 ) ) ;
#244705=ORIENTED_EDGE ( 'NONE', *, *, #255489, .F. ) ;
#244743=AXIS2_PLACEMENT_3D ( 'NONE', #66085, #206884, #89487 ) ;
#244791=CARTESIAN_POINT ( 'NONE',  ( -22.94999999999999929, 5.586869315528661062, 16.41686199900910736 ) ) ;
#244792=AXIS2_PLACEMENT_3D ( 'NONE', #219932, #140382, #120867 ) ;
#244803=DIRECTION ( 'NONE',  ( -0.000000000000000000, 0.1335171055202901413, 0.9910465087640860649 ) ) ;
#244809=DIRECTION ( 'NONE',  ( 0.000000000000000000, 0.000000000000000000, -1.000000000000000000 ) ) ;
#244810=ORIENTED_EDGE ( 'NONE', *, *, #118486, .F. ) ;
#244851=ORIENTED_EDGE ( 'NONE', *, *, #197254, .F. ) ;
#244916=CARTESIAN_POINT ( 'NONE',  ( -6.000000000000003553, -11.34999999999999964, 10.00000000000000178 ) ) ;
#244928=DIRECTION ( 'NONE',  ( 0.000000000000000000, -0.000000000000000000, 1.000000000000000000 ) ) ;
#244929=ORIENTED_EDGE ( 'NONE', *, *, #49825, .T. ) ;
#244935=CYLINDRICAL_SURFACE ( 'NONE', #186275, 0.09999999999999945044 ) ;
#244941=LINE ( 'NONE', #224085, #179086 ) ;
#244955=LINE ( 'NONE', #243678, #110475 ) ;
#244968=CIRCLE ( 'NONE', #178355, 0.1999999999999996503 ) ;
#244973=FACE_OUTER_BOUND ( 'NONE', #19532, .T. ) ;
#244998=EDGE_CURVE ( 'NONE', #163484, #93865, #22597, .T. ) ;
#245021=VERTEX_POINT ( 'NONE', #239005 ) ;
#245043=CARTESIAN_POINT ( 'NONE',  ( 0.8999999999999993561, -8.250000000000005329, 26.00000000000000355 ) ) ;
#245102=CARTESIAN_POINT ( 'NONE',  ( -20.90000000000000213, 11.59795743183152972, -1.899104650876408451 ) ) ;
#245129=ORIENTED_EDGE ( 'NONE', *, *, #151824, .F. ) ;
#245145=ADVANCED_FACE ( 'NONE', ( #147600 ), #11970, .T. ) ;
#245158=DIRECTION ( 'NONE',  ( 1.000000000000000000, 0.000000000000000000, 0.000000000000000000 ) ) ;
#245163=DIRECTION ( 'NONE',  ( -0.000000000000000000, 1.000000000000000000, -0.000000000000000000 ) ) ;
#245189=ADVANCED_FACE ( 'NONE', ( #211430 ), #73240, .T. ) ;
#245190=CARTESIAN_POINT ( 'NONE',  ( -19.89999999999999858, 4.513204987021263825, 22.00000000000000355 ) ) ;
#245202=EDGE_CURVE ( 'NONE', #32241, #13384, #205918, .T. ) ;
#245227=DIRECTION ( 'NONE',  ( 0.000000000000000000, 0.000000000000000000, -1.000000000000000000 ) ) ;
#245233=ORIENTED_EDGE ( 'NONE', *, *, #103394, .T. ) ;
#245272=AXIS2_PLACEMENT_3D ( 'NONE', #137216, #216747, #124092 ) ;
#245282=VECTOR ( 'NONE', #230633, 1000.000000000000000 ) ;
#245317=EDGE_CURVE ( 'NONE', #71198, #247436, #89740, .T. ) ;
#245349=AXIS2_PLACEMENT_3D ( 'NONE', #40024, #216044, #257688 ) ;
#245369=DIRECTION ( 'NONE',  ( -1.000000000000000000, 0.000000000000000000, 0.000000000000000000 ) ) ;
#245399=CARTESIAN_POINT ( 'NONE',  ( 18.79999999999999716, 7.900000000000000355, -1.300000000000000044 ) ) ;
#245402=AXIS2_PLACEMENT_3D ( 'NONE', #224304, #245163, #187767 ) ;
#245448=VECTOR ( 'NONE', #133710, 1000.000000000000000 ) ;
#245477=VERTEX_POINT ( 'NONE', #115039 ) ;
#245482=ORIENTED_EDGE ( 'NONE', *, *, #16207, .T. ) ;
#245495=DIRECTION ( 'NONE',  ( 1.476360405086644309E-16, -1.000000000000000000, 0.000000000000000000 ) ) ;
#245526=CARTESIAN_POINT ( 'NONE',  ( 5.899999999999995914, -11.65000000000000036, 10.10000000000000142 ) ) ;
#245562=VECTOR ( 'NONE', #223900, 1000.000000000000000 ) ;
#245573=VERTEX_POINT ( 'NONE', #77186 ) ;
#245618=DIRECTION ( 'NONE',  ( -1.000000000000000000, -0.000000000000000000, -0.000000000000000000 ) ) ;
#245624=VERTEX_POINT ( 'NONE', #133323 ) ;
#245662=DIRECTION ( 'NONE',  ( -1.000000000000000000, 0.000000000000000000, -0.000000000000000000 ) ) ;
#245675=EDGE_LOOP ( 'NONE', ( #91704, #72043, #47639, #148614 ) ) ;
#245709=DIRECTION ( 'NONE',  ( 0.000000000000000000, -1.000000000000000000, 0.000000000000000000 ) ) ;
#245743=EDGE_CURVE ( 'NONE', #10423, #181665, #253138, .T. ) ;
#245748=ORIENTED_EDGE ( 'NONE', *, *, #194459, .F. ) ;
#245761=CARTESIAN_POINT ( 'NONE',  ( 11.60000000000000142, -12.24999999999999822, 15.00000000000000355 ) ) ;
#245794=CARTESIAN_POINT ( 'NONE',  ( -18.79999999999999716, -1.467286812112899463, 33.00000000000000000 ) ) ;
#245856=DIRECTION ( 'NONE',  ( 1.000000000000000000, 0.000000000000000000, 0.000000000000000000 ) ) ;
#245877=EDGE_CURVE ( 'NONE', #147074, #184295, #203565, .T. ) ;
#245901=CARTESIAN_POINT ( 'NONE',  ( 18.59999999999999787, -10.84999999999999076, 33.00000000000000000 ) ) ;
#245906=CARTESIAN_POINT ( 'NONE',  ( -22.10000000000000497, 3.362550747017869046, 28.82623795144604983 ) ) ;
#245935=DIRECTION ( 'NONE',  ( 0.000000000000000000, 0.9856811345164827598, 0.1686199900910313187 ) ) ;
#245971=VERTEX_POINT ( 'NONE', #194299 ) ;
#245994=VECTOR ( 'NONE', #194964, 1000.000000000000227 ) ;
#246009=EDGE_CURVE ( 'NONE', #105564, #5669, #257866, .T. ) ;
#246034=CARTESIAN_POINT ( 'NONE',  ( 19.90000000000000568, 5.488301202077012775, 16.50000000000000000 ) ) ;
#246055=AXIS2_PLACEMENT_3D ( 'NONE', #61210, #161623, #222836 ) ;
#246068=EDGE_CURVE ( 'NONE', #42394, #245021, #182926, .T. ) ;
#246069=DIRECTION ( 'NONE',  ( 0.000000000000000000, 0.000000000000000000, 1.000000000000000000 ) ) ;
#246077=ORIENTED_EDGE ( 'NONE', *, *, #227790, .F. ) ;
#246089=FACE_OUTER_BOUND ( 'NONE', #194517, .T. ) ;
#246097=CARTESIAN_POINT ( 'NONE',  ( -13.40000000000000213, -8.279289321881350361, 11.02928932188134503 ) ) ;
#246100=ORIENTED_EDGE ( 'NONE', *, *, #242862, .T. ) ;
#246127=DIRECTION ( 'NONE',  ( -0.000000000000000000, -1.000000000000000000, -0.000000000000000000 ) ) ;
#246137=VERTEX_POINT ( 'NONE', #102843 ) ;
#246154=CARTESIAN_POINT ( 'NONE',  ( -20.09999999999999787, 4.645987002755569861, 21.91686199900910736 ) ) ;
#246164=CARTESIAN_POINT ( 'NONE',  ( 11.60000000000000142, -8.250000000000003553, 15.00000000000000355 ) ) ;
#246173=ORIENTED_EDGE ( 'NONE', *, *, #222194, .F. ) ;
#246191=PLANE ( 'NONE',  #182992 ) ;
#246195=SHAPE_REPRESENTATION_RELATIONSHIP ( 'NONE' , 'NONE' ,  #205135, #144814 ) ;
#246232=LINE ( 'NONE', #67588, #50503 ) ;
#246238=LINE ( 'NONE', #8910, #25338 ) ;
#246249=ADVANCED_FACE ( 'NONE', ( #186272 ), #125018, .T. ) ;
#246326=CARTESIAN_POINT ( 'NONE',  ( -18.79999999999999716, 1.250000000000000000, 16.60000000000000142 ) ) ;
#246378=VERTEX_POINT ( 'NONE', #115709 ) ;
#246388=EDGE_CURVE ( 'NONE', #243888, #88949, #214799, .T. ) ;
#246419=TOROIDAL_SURFACE ( 'NONE', #21568, 0.2000000000000000111, 0.1000000000000000056 ) ;
#246439=DIRECTION ( 'NONE',  ( 0.000000000000000000, 0.000000000000000000, -1.000000000000000000 ) ) ;
#246502=CARTESIAN_POINT ( 'NONE',  ( -18.69999999999999929, 7.973296578895943121, 1.410778198689827345 ) ) ;
#246552=ORIENTED_EDGE ( 'NONE', *, *, #63541, .F. ) ;
#246618=ORIENTED_EDGE ( 'NONE', *, *, #64339, .F. ) ;
#246624=CARTESIAN_POINT ( 'NONE',  ( -11.60000000000000320, -8.279289321881348584, 18.97071067811866030 ) ) ;
#246665=CARTESIAN_POINT ( 'NONE',  ( -19.99999999999999645, 4.528782138689107839, 21.95447128030237849 ) ) ;
#246669=AXIS2_PLACEMENT_3D ( 'NONE', #54846, #58691, #134379 ) ;
#246685=DIRECTION ( 'NONE',  ( 1.000000000000000000, 0.000000000000000000, 0.000000000000000000 ) ) ;
#246694=ORIENTED_EDGE ( 'NONE', *, *, #156190, .T. ) ;
#246719=ORIENTED_EDGE ( 'NONE', *, *, #65886, .F. ) ;
#246783=FACE_OUTER_BOUND ( 'NONE', #109353, .T. ) ;
#246789=EDGE_LOOP ( 'NONE', ( #21606, #157342, #21336, #10411 ) ) ;
#246805=CARTESIAN_POINT ( 'NONE',  ( -22.94999999999999929, 0.000000000000000000, 0.000000000000000000 ) ) ;
#246831=LINE ( 'NONE', #147749, #97800 ) ;
#246844=ORIENTED_EDGE ( 'NONE', *, *, #205126, .F. ) ;
#246868=EDGE_CURVE ( 'NONE', #135547, #86293, #143619, .T. ) ;
#246877=FACE_OUTER_BOUND ( 'NONE', #40857, .T. ) ;
#246883=ORIENTED_EDGE ( 'NONE', *, *, #69908, .T. ) ;
#246933=EDGE_LOOP ( 'NONE', ( #83235, #22879, #111143, #117491 ) ) ;
#246935=ORIENTED_EDGE ( 'NONE', *, *, #111160, .T. ) ;
#246943=ORIENTED_EDGE ( 'NONE', *, *, #41890, .F. ) ;
#246963=AXIS2_PLACEMENT_3D ( 'NONE', #61838, #141362, #121819 ) ;
#246970=CIRCLE ( 'NONE', #184432, 4.041421356237306917 ) ;
#247060=AXIS2_PLACEMENT_3D ( 'NONE', #135732, #195746, #17105 ) ;
#247115=CARTESIAN_POINT ( 'NONE',  ( 5.899999999999995914, -11.65000000000000036, 9.900000000000002132 ) ) ;
#247121=CARTESIAN_POINT ( 'NONE',  ( 18.79999999999999716, 1.149999999999999911, 16.60000000000000142 ) ) ;
#247133=EDGE_LOOP ( 'NONE', ( #113819, #64993, #82267, #234240 ) ) ;
#247169=CARTESIAN_POINT ( 'NONE',  ( -21.00000000000000000, -1.212568896937008089, -7.800000000000000711 ) ) ;
#247195=AXIS2_PLACEMENT_3D ( 'NONE', #167502, #68383, #41455 ) ;
#247221=ORIENTED_EDGE ( 'NONE', *, *, #17319, .F. ) ;
#247237=FACE_OUTER_BOUND ( 'NONE', #195263, .T. ) ;
#247294=CIRCLE ( 'NONE', #234848, 0.09999999999999961697 ) ;
#247313=DIRECTION ( 'NONE',  ( 0.000000000000000000, 0.000000000000000000, -1.000000000000000000 ) ) ;
#247331=DIRECTION ( 'NONE',  ( -0.000000000000000000, -1.000000000000000000, 0.000000000000000000 ) ) ;
#247346=ORIENTED_EDGE ( 'NONE', *, *, #131754, .F. ) ;
#247373=LINE ( 'NONE', #209546, #90702 ) ;
#247380=EDGE_CURVE ( 'NONE', #92448, #136069, #121233, .T. ) ;
#247387=LINE ( 'NONE', #127456, #119009 ) ;
#247404=ORIENTED_EDGE ( 'NONE', *, *, #36224, .F. ) ;
#247436=VERTEX_POINT ( 'NONE', #182466 ) ;
#247442=AXIS2_PLACEMENT_3D ( 'NONE', #161315, #240841, #3491 ) ;
#247452=VERTEX_POINT ( 'NONE', #205858 ) ;
#247465=AXIS2_PLACEMENT_3D ( 'NONE', #116130, #195683, #136957 ) ;
#247470=ORIENTED_EDGE ( 'NONE', *, *, #5094, .T. ) ;
#247476=PLANE ( 'NONE',  #15716 ) ;
#247506=VERTEX_POINT ( 'NONE', #208454 ) ;
#247509=ORIENTED_EDGE ( 'NONE', *, *, #233704, .F. ) ;
#247548=DIRECTION ( 'NONE',  ( 0.000000000000000000, 0.000000000000000000, -1.000000000000000000 ) ) ;
#247557=EDGE_LOOP ( 'NONE', ( #156771, #243874, #151799 ) ) ;
#247629=CARTESIAN_POINT ( 'NONE',  ( -22.94999999999999929, 11.49641995933507843, -1.885425182446134107 ) ) ;
#247664=ORIENTED_EDGE ( 'NONE', *, *, #112688, .F. ) ;
#247685=ORIENTED_EDGE ( 'NONE', *, *, #253646, .F. ) ;
#247785=EDGE_LOOP ( 'NONE', ( #25273, #227633, #159206, #49504 ) ) ;
#247852=CARTESIAN_POINT ( 'NONE',  ( -18.69999999999999929, -1.467286812112899463, 32.89999999999999858 ) ) ;
#247853=ORIENTED_EDGE ( 'NONE', *, *, #26813, .T. ) ;
#247904=CARTESIAN_POINT ( 'NONE',  ( -18.79999999999999716, 1.311673547813416718, -7.986648289447971116 ) ) ;
#247918=EDGE_LOOP ( 'NONE', ( #15253, #79822, #138342, #242918 ) ) ;
#247927=CARTESIAN_POINT ( 'NONE',  ( -20.90000000000000213, 11.59510167572422112, -1.901609089591594470 ) ) ;
#247972=AXIS2_PLACEMENT_3D ( 'NONE', #105850, #165870, #27663 ) ;
#247977=CARTESIAN_POINT ( 'NONE',  ( 20.90000000000000213, -1.885425182446133885, -11.49641995933507843 ) ) ;
#248038=DIRECTION ( 'NONE',  ( 0.000000000000000000, 0.000000000000000000, -1.000000000000000000 ) ) ;
#248086=DIRECTION ( 'NONE',  ( 0.000000000000000000, 1.000000000000000000, -0.000000000000000000 ) ) ;
#248131=ORIENTED_EDGE ( 'NONE', *, *, #45763, .F. ) ;
#248143=AXIS2_PLACEMENT_3D ( 'NONE', #241917, #163683, #204074 ) ;
#248161=ORIENTED_EDGE ( 'NONE', *, *, #173914, .F. ) ;
#248205=ORIENTED_EDGE ( 'NONE', *, *, #244998, .F. ) ;
#248206=DIRECTION ( 'NONE',  ( 0.000000000000000000, 0.1618390714546044939, 0.9868171638914228216 ) ) ;
#248280=FACE_BOUND ( 'NONE', #180031, .T. ) ;
#248287=CARTESIAN_POINT ( 'NONE',  ( 19.90000000000000568, 5.572646938319270937, 16.50000000000000000 ) ) ;
#248318=VERTEX_POINT ( 'NONE', #202669 ) ;
#248319=VERTEX_POINT ( 'NONE', #166158 ) ;
#248360=ORIENTED_EDGE ( 'NONE', *, *, #199853, .T. ) ;
#248363=AXIS2_PLACEMENT_3D ( 'NONE', #174314, #193837, #70052 ) ;
#248397=CIRCLE ( 'NONE', #119240, 0.09999999999999939493 ) ;
#248444=VERTEX_POINT ( 'NONE', #100666 ) ;
#248449=CARTESIAN_POINT ( 'NONE',  ( -22.10000000000000142, 3.461118860469513336, 28.84309995045515507 ) ) ;
#248480=ORIENTED_EDGE ( 'NONE', *, *, #226217, .F. ) ;
#248507=CARTESIAN_POINT ( 'NONE',  ( 20.90000000000000213, 7.800000000000000711, -1.300000000000000044 ) ) ;
#248541=LINE ( 'NONE', #128603, #16587 ) ;
#248550=DIRECTION ( 'NONE',  ( 0.000000000000000000, 0.000000000000000000, 1.000000000000000000 ) ) ;
#248553=CYLINDRICAL_SURFACE ( 'NONE', #234815, 0.09999999999999939493 ) ;
#248673=ADVANCED_FACE ( 'NONE', ( #74126 ), #17955, .T. ) ;
#248696=DIRECTION ( 'NONE',  ( 0.000000000000000000, 1.000000000000000000, 0.000000000000000000 ) ) ;
#248699=VERTEX_POINT ( 'NONE', #131494 ) ;
#248710=AXIS2_PLACEMENT_3D ( 'NONE', #237407, #176170, #64 ) ;
#248719=VECTOR ( 'NONE', #218025, 1000.000000000000000 ) ;
#248722=VERTEX_POINT ( 'NONE', #174538 ) ;
#248766=DIRECTION ( 'NONE',  ( -1.000000000000000000, -0.000000000000000000, -0.000000000000000000 ) ) ;
#248806=DIRECTION ( 'NONE',  ( -0.000000000000000000, 1.000000000000000000, -0.000000000000000000 ) ) ;
#248810=DIRECTION ( 'NONE',  ( -0.000000000000000000, 0.000000000000000000, -1.000000000000000000 ) ) ;
#248813=CARTESIAN_POINT ( 'NONE',  ( 18.79999999999999716, 7.800000000000000711, -1.212568896937008089 ) ) ;
#248824=EDGE_CURVE ( 'NONE', #40449, #155056, #221279, .T. ) ;
#248840=DIRECTION ( 'NONE',  ( -2.168404344971008868E-16, 0.000000000000000000, -1.000000000000000000 ) ) ;
#248849=ORIENTED_EDGE ( 'NONE', *, *, #153227, .F. ) ;
#248932=VECTOR ( 'NONE', #104080, 1000.000000000000000 ) ;
#248955=EDGE_LOOP ( 'NONE', ( #172233, #44531, #40010, #46114 ) ) ;
#248974=ADVANCED_FACE ( 'NONE', ( #148175 ), #129886, .T. ) ;
#248988=DIRECTION ( 'NONE',  ( -1.000000000000000000, 0.000000000000000000, 0.000000000000000000 ) ) ;
#249007=ORIENTED_EDGE ( 'NONE', *, *, #94389, .T. ) ;
#249092=VERTEX_POINT ( 'NONE', #73809 ) ;
#249105=DIRECTION ( 'NONE',  ( -1.000000000000000000, 0.000000000000000000, 3.469446951953515108E-14 ) ) ;
#249120=CARTESIAN_POINT ( 'NONE',  ( 20.90000000000000213, -1.300000000000000044, -7.900000000000000355 ) ) ;
#249127=CARTESIAN_POINT ( 'NONE',  ( -18.59999999999999787, -8.350000000000004974, 10.52591260281975138 ) ) ;
#249167=ORIENTED_EDGE ( 'NONE', *, *, #219413, .F. ) ;
#249174=CIRCLE ( 'NONE', #219940, 0.2000000000000005107 ) ;
#249190=CARTESIAN_POINT ( 'NONE',  ( -18.59999999999999787, -11.65000000000000036, 6.000000000000001776 ) ) ;
#249206=CARTESIAN_POINT ( 'NONE',  ( 20.90000000000000213, 6.356682116888462630, 11.91686199900910381 ) ) ;
#249213=FACE_OUTER_BOUND ( 'NONE', #180535, .T. ) ;
#249269=EDGE_CURVE ( 'NONE', #88476, #136640, #88120, .T. ) ;
#249273=EDGE_LOOP ( 'NONE', ( #123136, #239033, #255860, #257803 ) ) ;
#249292=ORIENTED_EDGE ( 'NONE', *, *, #191182, .F. ) ;
#249361=AXIS2_PLACEMENT_3D ( 'NONE', #224647, #164691, #146381 ) ;
#249404=DIRECTION ( 'NONE',  ( 0.000000000000000000, 0.000000000000000000, -1.000000000000000000 ) ) ;
#249462=DIRECTION ( 'NONE',  ( -1.000000000000000000, 0.000000000000000000, 0.000000000000000000 ) ) ;
#249465=ORIENTED_EDGE ( 'NONE', *, *, #219405, .F. ) ;
#249541=ADVANCED_FACE ( 'NONE', ( #80101 ), #221559, .T. ) ;
#249589=EDGE_CURVE ( 'NONE', #72694, #41292, #56693, .T. ) ;
#249597=SPHERICAL_SURFACE ( 'NONE', #210706, 0.1000000000000000056 ) ;
#249603=AXIS2_PLACEMENT_3D ( 'NONE', #99087, #176111, #178689 ) ;
#249625=AXIS2_PLACEMENT_3D ( 'NONE', #29530, #127315, #231559 ) ;
#249659=CIRCLE ( 'NONE', #45463, 0.1000000000000002554 ) ;
#249674=CIRCLE ( 'NONE', #245402, 0.09999999999999939493 ) ;
#249691=DIRECTION ( 'NONE',  ( -3.356945627403450689E-14, 0.9868171638914230437, 0.1618390714546045217 ) ) ;
#249693=ORIENTED_EDGE ( 'NONE', *, *, #153176, .T. ) ;
#249704=ORIENTED_EDGE ( 'NONE', *, *, #101636, .T. ) ;
#249749=DIRECTION ( 'NONE',  ( 0.000000000000000000, 0.1686199900910448357, -0.9856811345164804283 ) ) ;
#249773=FACE_OUTER_BOUND ( 'NONE', #216604, .T. ) ;
#249795=DIRECTION ( 'NONE',  ( -1.000000000000000000, 0.000000000000000000, 0.000000000000000000 ) ) ;
#249842=PLANE ( 'NONE',  #87622 ) ;
#249884=EDGE_CURVE ( 'NONE', #57087, #90690, #195960, .T. ) ;
#249886=CARTESIAN_POINT ( 'NONE',  ( 22.10000000000000142, 3.461118860469513336, 28.84309995045515507 ) ) ;
#249913=VECTOR ( 'NONE', #131563, 1000.000000000000000 ) ;
#249918=DIRECTION ( 'NONE',  ( 0.000000000000000000, 0.000000000000000000, 1.000000000000000000 ) ) ;
#249954=ORIENTED_EDGE ( 'NONE', *, *, #250668, .T. ) ;
#249970=ORIENTED_EDGE ( 'NONE', *, *, #131614, .T. ) ;
#250030=DIRECTION ( 'NONE',  ( -0.000000000000000000, 0.1686199900910294591, -0.9856811345164832039 ) ) ;
#250090=VECTOR ( 'NONE', #103147, 1000.000000000000000 ) ;
#250122=CARTESIAN_POINT ( 'NONE',  ( -19.99999999999999645, 1.250000000000000000, 16.60000000000000142 ) ) ;
#250142=CARTESIAN_POINT ( 'NONE',  ( 21.00000000000000000, 11.49641995933507843, -1.885425182446133885 ) ) ;
#250172=CIRCLE ( 'NONE', #179447, 0.09999999999999939493 ) ;
#250181=LINE ( 'NONE', #71564, #50058 ) ;
#250270=DIRECTION ( 'NONE',  ( 0.000000000000000000, 0.000000000000000000, 1.000000000000000000 ) ) ;
#250334=ADVANCED_FACE ( 'NONE', ( #155256 ), #99068, .F. ) ;
#250372=CARTESIAN_POINT ( 'NONE',  ( -21.00000000000000000, 1.212568896937007645, -8.000000000000000000 ) ) ;
#250376=ORIENTED_EDGE ( 'NONE', *, *, #71398, .T. ) ;
#250402=AXIS2_PLACEMENT_3D ( 'NONE', #21727, #197781, #3419 ) ;
#250403=CIRCLE ( 'NONE', #54590, 0.09999999999999939493 ) ;
#250468=CARTESIAN_POINT ( 'NONE',  ( 21.00983514138059505, 6.346420624576639469, 11.97684634237456613 ) ) ;
#250480=EDGE_LOOP ( 'NONE', ( #135500, #169513, #24143, #198095 ) ) ;
#250512=EDGE_CURVE ( 'NONE', #207912, #41292, #155357, .T. ) ;
#250537=CARTESIAN_POINT ( 'NONE',  ( 22.84999999999999787, 0.000000000000000000, 0.000000000000000000 ) ) ;
#250539=DIRECTION ( 'NONE',  ( 0.000000000000000000, 0.9856811345164832039, 0.1686199900910280158 ) ) ;
#250546=AXIS2_PLACEMENT_3D ( 'NONE', #108896, #183972, #242651 ) ;
#250595=ORIENTED_EDGE ( 'NONE', *, *, #236743, .T. ) ;
#250599=ORIENTED_EDGE ( 'NONE', *, *, #245317, .T. ) ;
#250611=DIRECTION ( 'NONE',  ( 0.000000000000000000, 1.156482317317873105E-15, -1.000000000000000000 ) ) ;
#250634=CARTESIAN_POINT ( 'NONE',  ( 22.94999999999999929, 0.000000000000000000, 4.000000000000000000 ) ) ;
#250659=ORIENTED_EDGE ( 'NONE', *, *, #59360, .T. ) ;
#250668=EDGE_CURVE ( 'NONE', #59743, #132097, #114499, .T. ) ;
#250693=FACE_OUTER_BOUND ( 'NONE', #65256, .T. ) ;
#250718=CARTESIAN_POINT ( 'NONE',  ( -22.94999999999999929, -1.212568896937008089, -8.000000000000000000 ) ) ;
#250730=FACE_OUTER_BOUND ( 'NONE', #246933, .T. ) ;
#250837=DIRECTION ( 'NONE',  ( -0.000000000000000000, -0.000000000000000000, -1.000000000000000000 ) ) ;
#250860=CIRCLE ( 'NONE', #155054, 4.000000000000000000 ) ;
#250883=ORIENTED_EDGE ( 'NONE', *, *, #37189, .F. ) ;
#250912=ORIENTED_EDGE ( 'NONE', *, *, #26293, .T. ) ;
#250927=DIRECTION ( 'NONE',  ( 0.000000000000000000, 0.7071067811865472397, -0.7071067811865479058 ) ) ;
#251026=ADVANCED_FACE ( 'NONE', ( #199856 ), #175186, .T. ) ;
#251049=CARTESIAN_POINT ( 'NONE',  ( -13.40000000000000036, -12.25000000000000178, 15.00000000000000355 ) ) ;
#251056=DIRECTION ( 'NONE',  ( 0.000000000000000000, 0.000000000000000000, -1.000000000000000000 ) ) ;
#251138=ORIENTED_EDGE ( 'NONE', *, *, #38623, .F. ) ;
#251165=ORIENTED_EDGE ( 'NONE', *, *, #116347, .T. ) ;
#251191=CIRCLE ( 'NONE', #201145, 0.2000000000000005107 ) ;
#251205=ORIENTED_EDGE ( 'NONE', *, *, #91802, .F. ) ;
#251265=ORIENTED_EDGE ( 'NONE', *, *, #164262, .F. ) ;
#251294=CIRCLE ( 'NONE', #205505, 0.09999999999999939493 ) ;
#251335=AXIS2_PLACEMENT_3D ( 'NONE', #132144, #207858, #29236 ) ;
#251343=ORIENTED_EDGE ( 'NONE', *, *, #62665, .F. ) ;
#251357=AXIS2_PLACEMENT_3D ( 'NONE', #17356, #138546, #79856 ) ;
#251375=DIRECTION ( 'NONE',  ( 0.000000000000000000, 0.000000000000000000, -1.000000000000000000 ) ) ;
#251424=AXIS2_PLACEMENT_3D ( 'NONE', #227838, #248696, #49204 ) ;
#251434=CIRCLE ( 'NONE', #18210, 0.09999999999999939493 ) ;
#251436=LINE ( 'NONE', #230601, #68927 ) ;
#251452=CARTESIAN_POINT ( 'NONE',  ( -6.100000000000012079, -11.65000000000000036, -15.00000000000000355 ) ) ;
#251490=ORIENTED_EDGE ( 'NONE', *, *, #114524, .T. ) ;
#251501=CARTESIAN_POINT ( 'NONE',  ( 18.79999999999999716, 8.000000000000000000, -1.212568896937008089 ) ) ;
#251551=ORIENTED_EDGE ( 'NONE', *, *, #234208, .F. ) ;
#251575=ADVANCED_FACE ( 'NONE', ( #85957 ), #183809, .T. ) ;
#251577=DIRECTION ( 'NONE',  ( 0.000000000000000000, 0.000000000000000000, 1.000000000000000000 ) ) ;
#251584=AXIS2_PLACEMENT_3D ( 'NONE', #216010, #139014, #200317 ) ;
#251616=CARTESIAN_POINT ( 'NONE',  ( 20.90000000000000213, -1.311673547813416718, -7.986648289447971116 ) ) ;
#251679=AXIS2_PLACEMENT_3D ( 'NONE', #161346, #40132, #83036 ) ;
#251682=EDGE_CURVE ( 'NONE', #171946, #206620, #214313, .T. ) ;
#251689=CARTESIAN_POINT ( 'NONE',  ( 21.00000000000000000, 6.258114003436814343, 11.90000000000000036 ) ) ;
#251707=CIRCLE ( 'NONE', #214300, 0.09999999999999990841 ) ;
#251761=DIRECTION ( 'NONE',  ( -1.000000000000000000, -0.000000000000000000, -0.000000000000000000 ) ) ;
#251793=ORIENTED_EDGE ( 'NONE', *, *, #186327, .T. ) ;
#251814=DIRECTION ( 'NONE',  ( 0.000000000000000000, 0.000000000000000000, -1.000000000000000000 ) ) ;
#251817=DIRECTION ( 'NONE',  ( 0.000000000000000000, 0.000000000000000000, -1.000000000000000000 ) ) ;
#251827=EDGE_CURVE ( 'NONE', #131589, #21663, #122756, .T. ) ;
#251833=CARTESIAN_POINT ( 'NONE',  ( -22.94999999999999929, -1.467286812112899463, 28.00000000000000000 ) ) ;
#251861=ORIENTED_EDGE ( 'NONE', *, *, #86158, .F. ) ;
#251889=EDGE_CURVE ( 'NONE', #238394, #224002, #43629, .T. ) ;
#251899=ORIENTED_EDGE ( 'NONE', *, *, #123908, .T. ) ;
#251961=CIRCLE ( 'NONE', #143806, 0.09999999999999939493 ) ;
#251963=CARTESIAN_POINT ( 'NONE',  ( 18.79999999999999716, 3.461118860469513336, 28.84309995045515507 ) ) ;
#251999=DIRECTION ( 'NONE',  ( -7.312726383247846713E-15, 0.1686199900910448357, -0.9856811345164804283 ) ) ;
#252070=AXIS2_PLACEMENT_3D ( 'NONE', #183471, #25681, #106460 ) ;
#252078=ORIENTED_EDGE ( 'NONE', *, *, #253546, .F. ) ;
#252091=CARTESIAN_POINT ( 'NONE',  ( 18.69999999999999929, 11.75000000000000000, 22.10000000000000142 ) ) ;
#252113=CARTESIAN_POINT ( 'NONE',  ( 0.000000000000000000, 1.350000000000000089, 16.60000000000000142 ) ) ;
#252167=CIRCLE ( 'NONE', #139736, 5.000000000000003553 ) ;
#252184=ORIENTED_EDGE ( 'NONE', *, *, #57736, .T. ) ;
#252186=EDGE_CURVE ( 'NONE', #81824, #157545, #135557, .T. ) ;
#252192=CARTESIAN_POINT ( 'NONE',  ( -21.00000000000000000, 11.49641995933507843, -1.885425182446133885 ) ) ;
#252208=( GEOMETRIC_REPRESENTATION_CONTEXT ( 3 ) GLOBAL_UNCERTAINTY_ASSIGNED_CONTEXT ( ( #71247 ) ) GLOBAL_UNIT_ASSIGNED_CONTEXT ( ( #148376, #209630, #87093 ) ) REPRESENTATION_CONTEXT ( 'NONE', 'WORKASPACE' ) );
#252213=EDGE_LOOP ( 'NONE', ( #214658, #59880, #52816, #37344 ) ) ;
#252246=DIRECTION ( 'NONE',  ( 1.000000000000000000, 0.000000000000000000, 0.000000000000000000 ) ) ;
#252252=AXIS2_PLACEMENT_3D ( 'NONE', #130473, #170947, #52210 ) ;
#252263=FACE_OUTER_BOUND ( 'NONE', #192347, .T. ) ;
#252293=DIRECTION ( 'NONE',  ( 1.000000000000000000, 0.000000000000000000, 0.000000000000000000 ) ) ;
#252359=CARTESIAN_POINT ( 'NONE',  ( -22.94999999999999929, 1.786320531569725478, -11.50977166988710820 ) ) ;
#252375=LINE ( 'NONE', #56724, #178919 ) ;
#252381=AXIS2_PLACEMENT_3D ( 'NONE', #139098, #221223, #236956 ) ;
#252417=DIRECTION ( 'NONE',  ( 0.000000000000000000, 0.9910465087640866200, 0.1335171055202867274 ) ) ;
#252440=VERTEX_POINT ( 'NONE', #205302 ) ;
#252469=ORIENTED_EDGE ( 'NONE', *, *, #17407, .T. ) ;
#252506=CIRCLE ( 'NONE', #40170, 0.09999999999999939493 ) ;
#252536=ORIENTED_EDGE ( 'NONE', *, *, #205007, .F. ) ;
#252550=ORIENTED_EDGE ( 'NONE', *, *, #39528, .T. ) ;
#252584=ORIENTED_EDGE ( 'NONE', *, *, #193313, .T. ) ;
#252608=ORIENTED_EDGE ( 'NONE', *, *, #249269, .T. ) ;
#252659=ORIENTED_EDGE ( 'NONE', *, *, #173899, .F. ) ;
#252660=EDGE_LOOP ( 'NONE', ( #154260, #217449, #74306, #220794 ) ) ;
#252669=ORIENTED_EDGE ( 'NONE', *, *, #44767, .F. ) ;
#252670=LINE ( 'NONE', #153642, #255446 ) ;
#252718=ADVANCED_FACE ( 'NONE', ( #190484 ), #146182, .F. ) ;
#252739=VERTEX_POINT ( 'NONE', #86187 ) ;
#252746=EDGE_CURVE ( 'NONE', #255181, #136640, #194035, .T. ) ;
#252756=ORIENTED_EDGE ( 'NONE', *, *, #104167, .F. ) ;
#252839=EDGE_CURVE ( 'NONE', #41107, #217842, #27466, .T. ) ;
#252852=ORIENTED_EDGE ( 'NONE', *, *, #69982, .F. ) ;
#252860=CARTESIAN_POINT ( 'NONE',  ( -18.79999999999999716, 1.350000000000000089, 22.10000000000000142 ) ) ;
#252874=CARTESIAN_POINT ( 'NONE',  ( -20.90000000000000213, 7.986648289447971116, 1.311673547813416718 ) ) ;
#252946=DIRECTION ( 'NONE',  ( 1.000000000000000000, 0.000000000000000000, 0.000000000000000000 ) ) ;
#252965=ADVANCED_FACE ( 'NONE', ( #73113 ), #152645, .F. ) ;
#252968=DIRECTION ( 'NONE',  ( 1.000000000000000000, -0.000000000000000000, -0.000000000000000000 ) ) ;
#252977=DIRECTION ( 'NONE',  ( 0.000000000000000000, -1.000000000000000000, 0.000000000000000000 ) ) ;
#253042=ADVANCED_FACE ( 'NONE', ( #183564 ), #195138, .T. ) ;
#253056=CARTESIAN_POINT ( 'NONE',  ( -22.10000000000000142, -11.65000000000000036, 32.89999999999999858 ) ) ;
#253108=ORIENTED_EDGE ( 'NONE', *, *, #194459, .T. ) ;
#253125=ORIENTED_EDGE ( 'NONE', *, *, #234376, .F. ) ;
#253138=( BOUNDED_CURVE ( )  B_SPLINE_CURVE ( 3, ( #69216, #84857, #104433, #90023 ),
 .UNSPECIFIED., .F., .F. ) 
 B_SPLINE_CURVE_WITH_KNOTS ( ( 4, 4 ),
 ( 3.141592653589793116, 4.712388980384689674 ),
 .UNSPECIFIED. ) 
 CURVE ( )  GEOMETRIC_REPRESENTATION_ITEM ( )  RATIONAL_B_SPLINE_CURVE ( ( 1.000000000000000000, 0.8047378541243649375, 0.8047378541243649375, 1.000000000000000000 ) ) 
 REPRESENTATION_ITEM ( '' )  );
#253207=CARTESIAN_POINT ( 'NONE',  ( 18.79999999999999361, -11.65000000000000036, -15.00000000000000000 ) ) ;
#253263=AXIS2_PLACEMENT_3D ( 'NONE', #41021, #180514, #81368 ) ;
#253273=DIRECTION ( 'NONE',  ( 0.000000000000000000, 0.9856811345164800953, 0.1686199900910462790 ) ) ;
#253305=FACE_OUTER_BOUND ( 'NONE', #28472, .T. ) ;
#253380=FACE_OUTER_BOUND ( 'NONE', #90235, .T. ) ;
#253397=AXIS2_PLACEMENT_3D ( 'NONE', #256110, #134915, #171542 ) ;
#253419=FACE_OUTER_BOUND ( 'NONE', #803, .T. ) ;
#253429=VECTOR ( 'NONE', #245618, 1000.000000000000000 ) ;
#253440=ORIENTED_EDGE ( 'NONE', *, *, #31853, .T. ) ;
#253454=ORIENTED_EDGE ( 'NONE', *, *, #216199, .T. ) ;
#253493=VECTOR ( 'NONE', #50632, 1000.000000000000000 ) ;
#253502=FACE_OUTER_BOUND ( 'NONE', #84188, .T. ) ;
#253508=VECTOR ( 'NONE', #128952, 1000.000000000000227 ) ;
#253515=VECTOR ( 'NONE', #221747, 1000.000000000000000 ) ;
#253530=DIRECTION ( 'NONE',  ( -1.000000000000000000, 0.000000000000000000, 0.000000000000000000 ) ) ;
#253546=EDGE_CURVE ( 'NONE', #25360, #82095, #77100, .T. ) ;
#253561=ORIENTED_EDGE ( 'NONE', *, *, #153792, .T. ) ;
#253563=AXIS2_PLACEMENT_3D ( 'NONE', #128231, #85205, #64404 ) ;
#253629=AXIS2_PLACEMENT_3D ( 'NONE', #183981, #5313, #84843 ) ;
#253646=EDGE_CURVE ( 'NONE', #238394, #213256, #81254, .T. ) ;
#253658=ORIENTED_EDGE ( 'NONE', *, *, #158539, .F. ) ;
#253681=EDGE_CURVE ( 'NONE', #113056, #166805, #185626, .T. ) ;
#253747=VERTEX_POINT ( 'NONE', #167269 ) ;
#253806=ADVANCED_FACE ( 'NONE', ( #70732 ), #193230, .F. ) ;
#253818=ORIENTED_EDGE ( 'NONE', *, *, #219564, .T. ) ;
#253847=CARTESIAN_POINT ( 'NONE',  ( 20.90000000000000213, -1.212568896937008089, -8.000000000000000000 ) ) ;
#253864=CARTESIAN_POINT ( 'NONE',  ( 20.90000000000000213, 1.410778198689825347, -7.973296578895943121 ) ) ;
#253943=FACE_OUTER_BOUND ( 'NONE', #144942, .T. ) ;
#253958=ADVANCED_FACE ( 'NONE', ( #195813 ), #143917, .T. ) ;
#253967=CARTESIAN_POINT ( 'NONE',  ( 13.40000000000000036, -8.350000000000004974, 15.00000000000000355 ) ) ;
#253988=VERTEX_POINT ( 'NONE', #35466 ) ;
#254013=CARTESIAN_POINT ( 'NONE',  ( 20.90000000000000213, 1.885425182446133885, -11.49641995933507843 ) ) ;
#254047=LINE ( 'NONE', #233243, #71816 ) ;
#254062=CARTESIAN_POINT ( 'NONE',  ( -22.94999999999999929, 11.59510167572422112, -1.901609089591594692 ) ) ;
#254080=VERTEX_POINT ( 'NONE', #245190 ) ;
#254098=DIRECTION ( 'NONE',  ( 1.000000000000000000, 0.000000000000000000, 0.000000000000000000 ) ) ;
#254114=EDGE_CURVE ( 'NONE', #145044, #109487, #243889, .T. ) ;
#254130=ADVANCED_FACE ( 'NONE', ( #65257 ), #200919, .T. ) ;
#254137=CARTESIAN_POINT ( 'NONE',  ( -19.99999999999999645, 11.61130914238355771, 22.00000000000000355 ) ) ;
#254139=VERTEX_POINT ( 'NONE', #172106 ) ;
#254168=EDGE_LOOP ( 'NONE', ( #161633, #32025, #143181, #169969 ) ) ;
#254214=DIRECTION ( 'NONE',  ( 0.000000000000000000, 0.000000000000000000, -1.000000000000000000 ) ) ;
#254216=CARTESIAN_POINT ( 'NONE',  ( 18.59999999999999787, 11.75000000000000000, 5.900000000000001243 ) ) ;
#254242=CARTESIAN_POINT ( 'NONE',  ( -21.10000000000000142, 4.898587196589412829E-16, 4.000000000000000000 ) ) ;
#254250=EDGE_CURVE ( 'NONE', #175526, #154676, #170835, .T. ) ;
#254298=VECTOR ( 'NONE', #103097, 1000.000000000000000 ) ;
#254313=FACE_OUTER_BOUND ( 'NONE', #20795, .T. ) ;
#254350=DIRECTION ( 'NONE',  ( 1.000000000000000000, 0.000000000000000000, 0.000000000000000000 ) ) ;
#254370=EDGE_LOOP ( 'NONE', ( #257360, #166645, #167782 ) ) ;
#254395=DIRECTION ( 'NONE',  ( 0.000000000000000000, 0.000000000000000000, -1.000000000000000000 ) ) ;
#254397=VERTEX_POINT ( 'NONE', #252874 ) ;
#254419=DIRECTION ( 'NONE',  ( 0.000000000000000000, -0.000000000000000000, 1.000000000000000000 ) ) ;
#254436=ORIENTED_EDGE ( 'NONE', *, *, #48446, .T. ) ;
#254469=CARTESIAN_POINT ( 'NONE',  ( -18.79999999999999716, 1.350000000000000089, 16.39999999999999858 ) ) ;
#254509=DIRECTION ( 'NONE',  ( 1.476360405086644309E-16, -1.000000000000000000, -1.445602896647339410E-16 ) ) ;
#254536=LINE ( 'NONE', #113766, #98535 ) ;
#254545=DIRECTION ( 'NONE',  ( 0.000000000000000000, 1.000000000000000000, 0.000000000000000000 ) ) ;
#254552=CIRCLE ( 'NONE', #217141, 0.09999999999999939493 ) ;
#254650=CIRCLE ( 'NONE', #204788, 0.09999999999999939493 ) ;
#254752=DIRECTION ( 'NONE',  ( 1.000000000000000000, 0.000000000000000000, 0.000000000000000000 ) ) ;
#254761=VECTOR ( 'NONE', #244928, 1000.000000000000000 ) ;
#254778=DIRECTION ( 'NONE',  ( 0.000000000000000000, 0.000000000000000000, 1.000000000000000000 ) ) ;
#254792=CARTESIAN_POINT ( 'NONE',  ( 18.69999999999999929, -8.150000000000007461, 32.89999999999999858 ) ) ;
#254824=ORIENTED_EDGE ( 'NONE', *, *, #250512, .T. ) ;
#254826=DIRECTION ( 'NONE',  ( 1.000000000000000000, 0.000000000000000000, 0.000000000000000000 ) ) ;
#254876=FACE_OUTER_BOUND ( 'NONE', #97774, .T. ) ;
#254884=DIRECTION ( 'NONE',  ( 0.000000000000000000, -0.1335171055202867274, -0.9910465087640866200 ) ) ;
#254958=DIRECTION ( 'NONE',  ( -1.000000000000000000, 0.000000000000000000, -0.000000000000000000 ) ) ;
#254985=ADVANCED_FACE ( 'NONE', ( #18475 ), #135834, .T. ) ;
#255060=FACE_OUTER_BOUND ( 'NONE', #189162, .T. ) ;
#255174=DIRECTION ( 'NONE',  ( -0.000000000000000000, -1.000000000000000000, -0.000000000000000000 ) ) ;
#255181=VERTEX_POINT ( 'NONE', #246502 ) ;
#255186=LINE ( 'NONE', #58306, #134709 ) ;
#255187=DIRECTION ( 'NONE',  ( 0.000000000000000000, 0.000000000000000000, 1.000000000000000000 ) ) ;
#255212=AXIS2_PLACEMENT_3D ( 'NONE', #196331, #195082, #35999 ) ;
#255233=CARTESIAN_POINT ( 'NONE',  ( 21.04552871983375795, 6.223900101736508539, 12.00000000000000178 ) ) ;
#255278=PLANE ( 'NONE',  #222804 ) ;
#255294=ADVANCED_FACE ( 'NONE', ( #70481 ), #131696, .T. ) ;
#255298=DIRECTION ( 'NONE',  ( -0.000000000000000000, -0.1335171055202867274, -0.9910465087640865089 ) ) ;
#255336=CARTESIAN_POINT ( 'NONE',  ( -19.89999999999999858, 4.513204987021263825, 22.10000000000000142 ) ) ;
#255341=CARTESIAN_POINT ( 'NONE',  ( 13.40000000000000036, -8.250000000000003553, 15.00000000000000355 ) ) ;
#255362=ORIENTED_EDGE ( 'NONE', *, *, #183752, .F. ) ;
#255392=ORIENTED_EDGE ( 'NONE', *, *, #202062, .F. ) ;
#255408=CYLINDRICAL_SURFACE ( 'NONE', #77782, 4.000000000000000000 ) ;
#255416=DIRECTION ( 'NONE',  ( 0.000000000000000000, 0.000000000000000000, -1.000000000000000000 ) ) ;
#255423=CARTESIAN_POINT ( 'NONE',  ( -5.900000000000003020, -11.75000000000000000, 10.00000000000000178 ) ) ;
#255446=VECTOR ( 'NONE', #213546, 1000.000000000000000 ) ;
#255464=CARTESIAN_POINT ( 'NONE',  ( 20.90000000000000213, 6.841561409100513025, 9.675512259591560138 ) ) ;
#255488=CARTESIAN_POINT ( 'NONE',  ( 11.60000000000000142, -11.75000000000000000, 17.70000000000000284 ) ) ;
#255489=EDGE_CURVE ( 'NONE', #36888, #86236, #22035, .T. ) ;
#255506=CARTESIAN_POINT ( 'NONE',  ( -22.94999999999999929, -1.467286812112899463, 28.00000000000000000 ) ) ;
#255584=CARTESIAN_POINT ( 'NONE',  ( -18.69999999999999929, 1.250000000000000000, 21.90000000000000213 ) ) ;
#255596=EDGE_CURVE ( 'NONE', #59508, #12728, #161550, .T. ) ;
#255607=ADVANCED_FACE ( 'NONE', ( #63704 ), #45432, .F. ) ;
#255611=CARTESIAN_POINT ( 'NONE',  ( -22.19999999999999929, -1.467286812112899463, 32.89999999999999858 ) ) ;
#255675=CIRCLE ( 'NONE', #80737, 0.1000000000000000472 ) ;
#255683=DIRECTION ( 'NONE',  ( -0.000000000000000000, 1.000000000000000000, -0.000000000000000000 ) ) ;
#255688=FACE_OUTER_BOUND ( 'NONE', #203345, .T. ) ;
#255693=DIRECTION ( 'NONE',  ( 0.000000000000000000, 0.000000000000000000, -1.000000000000000000 ) ) ;
#255708=CARTESIAN_POINT ( 'NONE',  ( 5.899999999999995914, -11.75000000000000000, 9.900000000000002132 ) ) ;
#255781=FACE_OUTER_BOUND ( 'NONE', #110601, .T. ) ;
#255799=EDGE_CURVE ( 'NONE', #131374, #69570, #92553, .T. ) ;
#255821=AXIS2_PLACEMENT_3D ( 'NONE', #50208, #90619, #73672 ) ;
#255857=CARTESIAN_POINT ( 'NONE',  ( -20.90000000000000213, 11.49641995933507843, -1.885425182446133885 ) ) ;
#255860=ORIENTED_EDGE ( 'NONE', *, *, #106544, .F. ) ;
#255881=ORIENTED_EDGE ( 'NONE', *, *, #173357, .F. ) ;
#255884=VECTOR ( 'NONE', #99773, 1000.000000000000000 ) ;
#255967=VERTEX_POINT ( 'NONE', #825 ) ;
#255969=ORIENTED_EDGE ( 'NONE', *, *, #98558, .T. ) ;
#255981=CARTESIAN_POINT ( 'NONE',  ( -20.90000000000000213, -11.65000000000000036, -15.00000000000000000 ) ) ;
#255993=CARTESIAN_POINT ( 'NONE',  ( -13.40000000000000213, -11.65000000000000036, 17.70000000000000284 ) ) ;
#256004=ORIENTED_EDGE ( 'NONE', *, *, #229667, .F. ) ;
#256018=CARTESIAN_POINT ( 'NONE',  ( 22.10000000000000853, 3.461118860469513336, 28.84309995045515507 ) ) ;
#256037=CIRCLE ( 'NONE', #51888, 0.09999999999999939493 ) ;
#256052=ADVANCED_FACE ( 'NONE', ( #134586 ), #112495, .F. ) ;
#256065=CIRCLE ( 'NONE', #139409, 0.09999999999999939493 ) ;
#256110=CARTESIAN_POINT ( 'NONE',  ( -21.10000000000000142, 0.000000000000000000, 4.100000000000000533 ) ) ;
#256118=DIRECTION ( 'NONE',  ( 1.000000000000000000, 0.000000000000000000, 0.000000000000000000 ) ) ;
#256123=DIRECTION ( 'NONE',  ( 0.000000000000000000, 0.000000000000000000, -1.000000000000000000 ) ) ;
#256146=DIRECTION ( 'NONE',  ( 0.000000000000000000, 0.000000000000000000, 1.000000000000000000 ) ) ;
#256218=CARTESIAN_POINT ( 'NONE',  ( 18.59999999999999787, -8.350000000000004974, 10.52591260281975138 ) ) ;
#256233=AXIS2_PLACEMENT_3D ( 'NONE', #9732, #129687, #8468 ) ;
#256236=DIRECTION ( 'NONE',  ( 0.000000000000000000, 0.000000000000000000, 1.000000000000000000 ) ) ;
#256305=EDGE_CURVE ( 'NONE', #84823, #254080, #226154, .T. ) ;
#256316=DIRECTION ( 'NONE',  ( 1.000000000000000000, 0.000000000000000000, 0.000000000000000000 ) ) ;
#256329=DIRECTION ( 'NONE',  ( 0.000000000000000000, 0.000000000000000000, -1.000000000000000000 ) ) ;
#256343=ORIENTED_EDGE ( 'NONE', *, *, #138721, .T. ) ;
#256387=VERTEX_POINT ( 'NONE', #59729 ) ;
#256395=DIRECTION ( 'NONE',  ( 1.000000000000000000, -1.476360405086644309E-16, 0.000000000000000000 ) ) ;
#256398=SPHERICAL_SURFACE ( 'NONE', #245349, 0.1000000000000000056 ) ;
#256423=DIRECTION ( 'NONE',  ( -1.000000000000000000, 0.000000000000000000, 0.000000000000000000 ) ) ;
#256430=AXIS2_PLACEMENT_3D ( 'NONE', #157239, #254958, #155955 ) ;
#256432=CIRCLE ( 'NONE', #135868, 0.1000000000000000749 ) ;
#256505=CARTESIAN_POINT ( 'NONE',  ( 21.10000000000000142, 6.223900101154155706, 12.00000000000000178 ) ) ;
#256543=EDGE_CURVE ( 'NONE', #172709, #88008, #206004, .T. ) ;
#256556=EDGE_CURVE ( 'NONE', #171323, #139155, #9899, .T. ) ;
#256561=EDGE_CURVE ( 'NONE', #234077, #27940, #147308, .T. ) ;
#256567=CARTESIAN_POINT ( 'NONE',  ( -22.94999999999999929, 1.885425182446134107, -11.59641995933507808 ) ) ;
#256628=EDGE_LOOP ( 'NONE', ( #45102, #99189, #104646, #115672 ) ) ;
#256657=CARTESIAN_POINT ( 'NONE',  ( -37.88850191057539973, -10.80884033489985363, 6.100000000000002309 ) ) ;
#256719=VERTEX_POINT ( 'NONE', #37656 ) ;
#256752=PLANE ( 'NONE',  #137335 ) ;
#256872=ORIENTED_EDGE ( 'NONE', *, *, #151809, .F. ) ;
#256884=CARTESIAN_POINT ( 'NONE',  ( -11.60000000000000320, -11.65000000000000036, 12.40000000000000391 ) ) ;
#256894=EDGE_CURVE ( 'NONE', #158009, #1224, #18468, .T. ) ;
#256931=ORIENTED_EDGE ( 'NONE', *, *, #257421, .F. ) ;
#257022=CYLINDRICAL_SURFACE ( 'NONE', #188867, 0.1000000000000002554 ) ;
#257032=LINE ( 'NONE', #17208, #215410 ) ;
#257039=CYLINDRICAL_SURFACE ( 'NONE', #250546, 0.09999999999999939493 ) ;
#257073=AXIS2_PLACEMENT_3D ( 'NONE', #174635, #254098, #167234 ) ;
#257092=FACE_OUTER_BOUND ( 'NONE', #174648, .T. ) ;
#257098=CIRCLE ( 'NONE', #165591, 11.75000000000000000 ) ;
#257114=DIRECTION ( 'NONE',  ( 0.000000000000000000, 0.000000000000000000, -1.000000000000000000 ) ) ;
#257161=AXIS2_PLACEMENT_3D ( 'NONE', #168845, #227472, #48842 ) ;
#257199=VECTOR ( 'NONE', #76623, 1000.000000000000000 ) ;
#257219=DIRECTION ( 'NONE',  ( 0.000000000000000000, 0.1335171055202864221, 0.9910465087640865089 ) ) ;
#257310=LINE ( 'NONE', #34497, #3734 ) ;
#257319=CARTESIAN_POINT ( 'NONE',  ( -18.69999999999999929, -1.885425182446132997, -11.49641995933507843 ) ) ;
#257330=VECTOR ( 'NONE', #65073, 999.9999999999998863 ) ;
#257360=ORIENTED_EDGE ( 'NONE', *, *, #51566, .F. ) ;
#257388=CARTESIAN_POINT ( 'NONE',  ( 20.90000000000000213, 7.800000000000000711, 1.212568896937007867 ) ) ;
#257420=DIRECTION ( 'NONE',  ( -1.000000000000000000, -0.000000000000000000, -0.000000000000000000 ) ) ;
#257421=EDGE_CURVE ( 'NONE', #56541, #44902, #51939, .T. ) ;
#257422=DIRECTION ( 'NONE',  ( 0.000000000000000000, 0.000000000000000000, 1.000000000000000000 ) ) ;
#257433=CIRCLE ( 'NONE', #253397, 0.1000000000000002554 ) ;
#257493=VECTOR ( 'NONE', #133899, 1000.000000000000227 ) ;
#257506=DIRECTION ( 'NONE',  ( 0.000000000000000000, -1.000000000000000000, 0.000000000000000000 ) ) ;
#257513=ORIENTED_EDGE ( 'NONE', *, *, #217302, .F. ) ;
#257519=CARTESIAN_POINT ( 'NONE',  ( -6.000000000000003553, -11.34999999999999964, 10.10000000000000142 ) ) ;
#257550=CIRCLE ( 'NONE', #16050, 0.1000000000000001860 ) ;
#257594=CARTESIAN_POINT ( 'NONE',  ( 20.90000000000000213, 1.885425182446133885, -11.49641995933507843 ) ) ;
#257597=CIRCLE ( 'NONE', #228459, 0.09999999999999939493 ) ;
#257600=ADVANCED_FACE ( 'NONE', ( #126507 ), #122676, .T. ) ;
#257616=DIRECTION ( 'NONE',  ( 0.000000000000000000, 0.000000000000000000, -1.000000000000000000 ) ) ;
#257626=CARTESIAN_POINT ( 'NONE',  ( -20.90000000000000213, 7.800000000000000711, -1.300000000000000044 ) ) ;
#257631=DIRECTION ( 'NONE',  ( -1.000000000000000000, 0.000000000000000000, 0.000000000000000000 ) ) ;
#257637=ORIENTED_EDGE ( 'NONE', *, *, #236214, .T. ) ;
#257656=DIRECTION ( 'NONE',  ( -1.000000000000000000, 0.000000000000000000, -0.000000000000000000 ) ) ;
#257660=EDGE_LOOP ( 'NONE', ( #185991, #196593, #242916, #199962 ) ) ;
#257688=DIRECTION ( 'NONE',  ( 1.000000000000000000, 0.000000000000000000, 0.000000000000000000 ) ) ;
#257691=SPHERICAL_SURFACE ( 'NONE', #202255, 0.1000000000000000056 ) ;
#257694=EDGE_LOOP ( 'NONE', ( #55881, #6406, #45492, #120158 ) ) ;
#257726=ORIENTED_EDGE ( 'NONE', *, *, #155913, .T. ) ;
#257741=EDGE_LOOP ( 'NONE', ( #65209, #200820, #93750, #205789 ) ) ;
#257773=EDGE_LOOP ( 'NONE', ( #158027, #120442, #32988, #97530 ) ) ;
#257782=DIRECTION ( 'NONE',  ( 0.000000000000000000, -0.9910465087640865089, -0.1335171055202864221 ) ) ;
#257795=LINE ( 'NONE', #81740, #143725 ) ;
#257803=ORIENTED_EDGE ( 'NONE', *, *, #48142, .F. ) ;
#257810=ORIENTED_EDGE ( 'NONE', *, *, #70681, .F. ) ;
#257812=EDGE_CURVE ( 'NONE', #163992, #114614, #48050, .T. ) ;
#257838=DIRECTION ( 'NONE',  ( 0.000000000000000000, 0.000000000000000000, 1.000000000000000000 ) ) ;
#257866=CIRCLE ( 'NONE', #20429, 11.65000000000000036 ) ;
#257919=ADVANCED_FACE ( 'NONE', ( #117214 ), #174672, .T. ) ;
#257929=AXIS2_PLACEMENT_3D ( 'NONE', #4689, #45123, #2129 ) ;
#257930=DIRECTION ( 'NONE',  ( 0.000000000000000000, 1.000000000000000000, 0.000000000000000000 ) ) ;
#257939=DIRECTION ( 'NONE',  ( 1.000000000000000000, -0.000000000000000000, -0.000000000000000000 ) ) ;
#257950=ORIENTED_EDGE ( 'NONE', *, *, #154004, .T. ) ;
#257969=DIRECTION ( 'NONE',  ( 0.000000000000000000, 0.9910465087640866200, -0.1335171055202867274 ) ) ;
#257982=VERTEX_POINT ( 'NONE', #239732 ) ;
#258051=( BOUNDED_CURVE ( )  B_SPLINE_CURVE ( 3, ( #181269, #183812, #44316, #63867 ),
 .UNSPECIFIED., .F., .F. ) 
 B_SPLINE_CURVE_WITH_KNOTS ( ( 4, 4 ),
 ( 1.570796326794893893, 3.141592653589793116 ),
 .UNSPECIFIED. ) 
 CURVE ( )  GEOMETRIC_REPRESENTATION_ITEM ( )  RATIONAL_B_SPLINE_CURVE ( ( 1.000000000000000000, 0.8047378541243643824, 0.8047378541243643824, 1.000000000000000000 ) ) 
 REPRESENTATION_ITEM ( '' )  );
#258059=DIRECTION ( 'NONE',  ( -0.000000000000000000, 1.000000000000000000, 0.000000000000000000 ) ) ;
ENDSEC;
END-ISO-10303-21;
